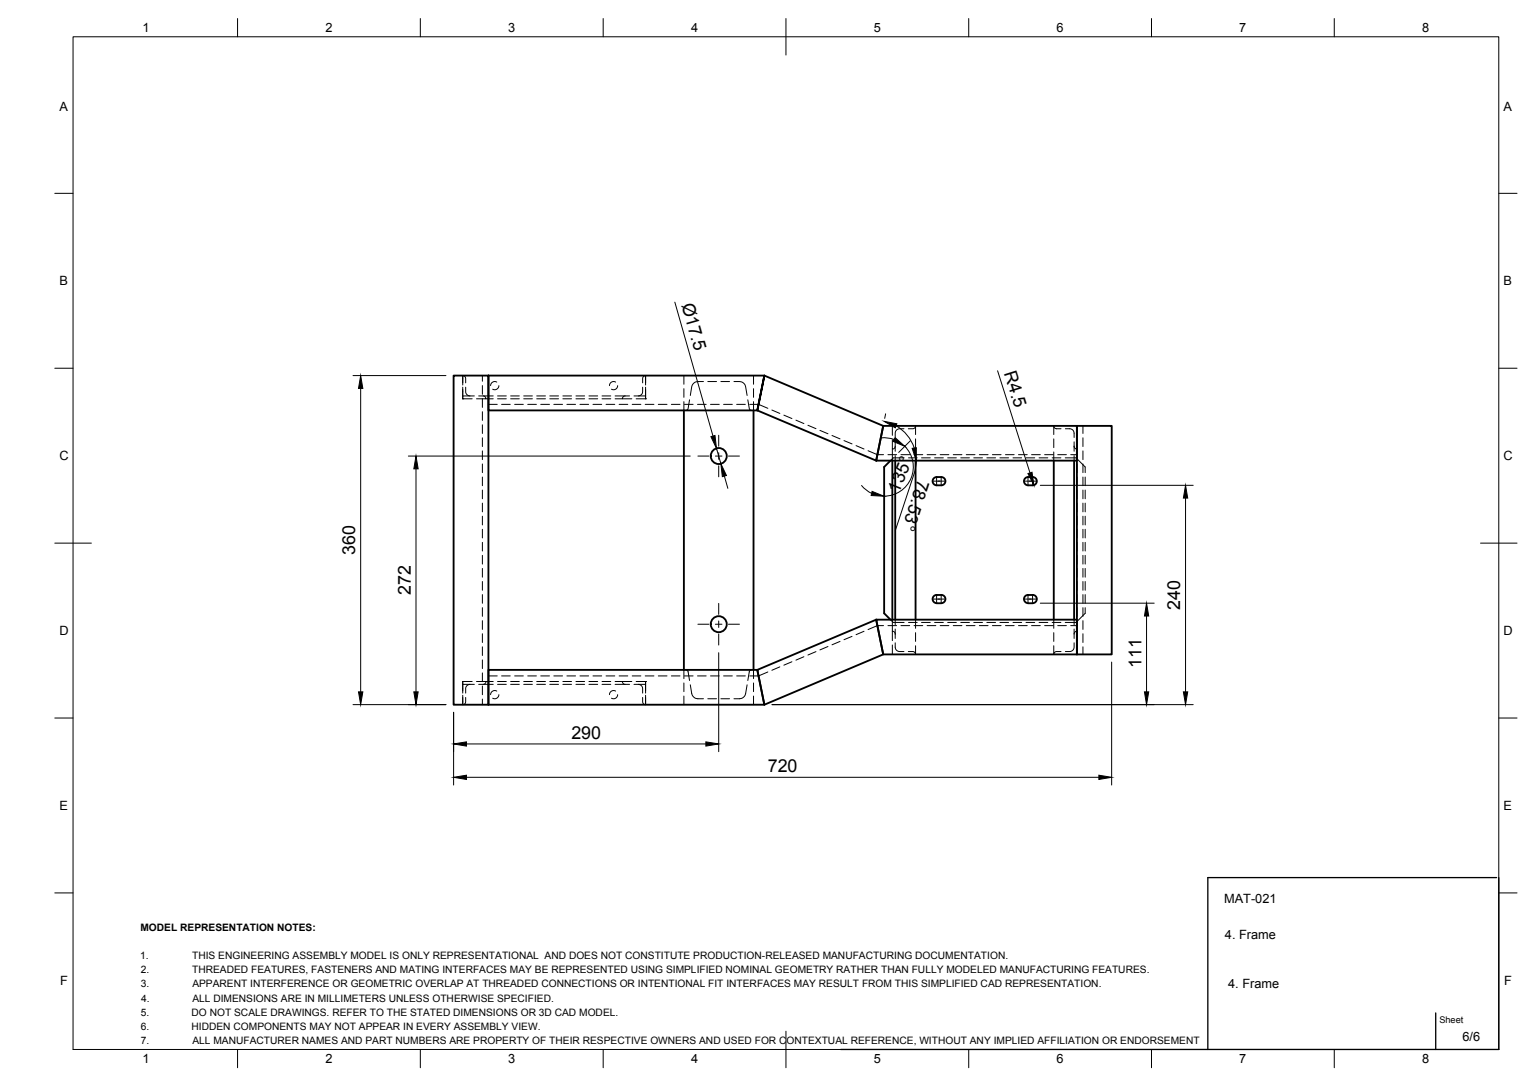
ISO-10303-21;
HEADER;
/* Generated by software containing ST-Developer
 * from STEP Tools, Inc. (www.steptools.com) 
 */

FILE_DESCRIPTION(
/* description */ ('STEP AP214'),
/* implementation_level */ '2;1');

FILE_NAME(
/* name */ '4. Frame.step',
/* time_stamp */ '2026-11-14T06:27:21-08:00',
/* author */ (''),
/* organization */ (''),
/* preprocessor_version */ 'ST-DEVELOPER v20.2',
/* originating_system */ 'Autodesk Translation Framework v15.17.0.0',
/* authorisation */ '');

FILE_SCHEMA (('AUTOMOTIVE_DESIGN { 1 0 10303 214 3 1 1 }'));
ENDSEC;

DATA;
#10=MECHANICAL_DESIGN_GEOMETRIC_PRESENTATION_REPRESENTATION('',(#38,#39,#40,#41,#42,#43,#44,#45,#46,#47,#48,#49,#50,#51,#52,#53,#54,#55,#56,#57,#58,#59,#60,#61),#27541);
#30=SHAPE_REPRESENTATION_RELATIONSHIP('SRR','None',#27564,#34);
#34=ADVANCED_BREP_SHAPE_REPRESENTATION('',(#65,#66,#67,#68,#69,#70,#71,
#72,#73,#74,#75,#76,#77,#78,#79,#80,#81,#82,#83,#84,#85,#86,#87,#88),#27540);
#38=STYLED_ITEM('',(#27590),#65);
#39=STYLED_ITEM('',(#27590),#66);
#40=STYLED_ITEM('',(#27590),#67);
#41=STYLED_ITEM('',(#27590),#68);
#42=STYLED_ITEM('',(#27590),#69);
#43=STYLED_ITEM('',(#27590),#70);
#44=STYLED_ITEM('',(#27590),#71);
#45=STYLED_ITEM('',(#27590),#72);
#46=STYLED_ITEM('',(#27590),#73);
#47=STYLED_ITEM('',(#27590),#74);
#48=STYLED_ITEM('',(#27590),#75);
#49=STYLED_ITEM('',(#27590),#76);
#50=STYLED_ITEM('',(#27590),#77);
#51=STYLED_ITEM('',(#27590),#78);
#52=STYLED_ITEM('',(#27590),#79);
#53=STYLED_ITEM('',(#27590),#80);
#54=STYLED_ITEM('',(#27590),#81);
#55=STYLED_ITEM('',(#27590),#82);
#56=STYLED_ITEM('',(#27590),#83);
#57=STYLED_ITEM('',(#27590),#84);
#58=STYLED_ITEM('',(#27590),#85);
#59=STYLED_ITEM('',(#27590),#86);
#60=STYLED_ITEM('',(#27590),#87);
#61=STYLED_ITEM('',(#27590),#88);
#65=MANIFOLD_SOLID_BREP('Body1',#11826);
#66=MANIFOLD_SOLID_BREP('Body2',#11827);
#67=MANIFOLD_SOLID_BREP('Body3',#11828);
#68=MANIFOLD_SOLID_BREP('Body4',#11829);
#69=MANIFOLD_SOLID_BREP('Body5',#11830);
#70=MANIFOLD_SOLID_BREP('Body6',#11831);
#71=MANIFOLD_SOLID_BREP('Body7',#11832);
#72=MANIFOLD_SOLID_BREP('Body8',#11833);
#73=MANIFOLD_SOLID_BREP('Body9',#11834);
#74=MANIFOLD_SOLID_BREP('Body10',#11835);
#75=MANIFOLD_SOLID_BREP('Body11',#11836);
#76=MANIFOLD_SOLID_BREP('Body12',#11837);
#77=MANIFOLD_SOLID_BREP('Body13',#11838);
#78=MANIFOLD_SOLID_BREP('Body14',#11839);
#79=MANIFOLD_SOLID_BREP('Body15',#11840);
#80=MANIFOLD_SOLID_BREP('Body16',#11841);
#81=MANIFOLD_SOLID_BREP('Body17',#11842);
#82=MANIFOLD_SOLID_BREP('Body18',#11843);
#83=MANIFOLD_SOLID_BREP('Body19',#11844);
#84=MANIFOLD_SOLID_BREP('Body20',#11845);
#85=MANIFOLD_SOLID_BREP('Body21',#11846);
#86=MANIFOLD_SOLID_BREP('Body22',#11847);
#87=MANIFOLD_SOLID_BREP('Body23',#11848);
#88=MANIFOLD_SOLID_BREP('Body24',#11849);
#133=ELLIPSE('',#12698,2.59172390171958,2.54000000000056);
#134=ELLIPSE('',#12701,6.9976545346413,6.85800000000022);
#135=ELLIPSE('',#12704,6.99765453464393,6.85800000000241);
#136=ELLIPSE('',#12707,2.59172390171943,2.54000000000021);
#137=ELLIPSE('',#12712,2.59172390172017,2.54000000000112);
#138=ELLIPSE('',#12713,6.99765453464255,6.8580000000014);
#139=ELLIPSE('',#12714,6.99765453464257,6.85800000000131);
#140=ELLIPSE('',#12715,2.59172390172489,2.5400000000054);
#141=ELLIPSE('',#12720,2.59172390172243,2.54000000000345);
#142=ELLIPSE('',#12723,6.99765453464225,6.85800000000097);
#143=ELLIPSE('',#12726,6.99765453464551,6.8580000000038);
#144=ELLIPSE('',#12729,2.59172390171343,2.53999999999498);
#145=ELLIPSE('',#12737,2.59172390171873,2.53999999999979);
#146=ELLIPSE('',#12741,6.99765453464068,6.85799999999964);
#147=ELLIPSE('',#12745,6.99765453464442,6.85800000000265);
#148=ELLIPSE('',#12749,2.5917239017157,2.53999999999687);
#149=ELLIPSE('',#12786,2.59172390172123,2.54000000000197);
#150=ELLIPSE('',#12789,6.99765453463971,6.85799999999854);
#151=ELLIPSE('',#12792,6.99765453464465,6.85800000000273);
#152=ELLIPSE('',#12795,2.59172390171767,2.53999999999863);
#153=ELLIPSE('',#12802,2.59172390172269,2.54000000000292);
#154=ELLIPSE('',#12806,6.99765453464155,6.85800000000042);
#155=ELLIPSE('',#12810,6.99765453463736,6.85799999999707);
#156=ELLIPSE('',#12814,2.59172390171622,2.5399999999978);
#157=ELLIPSE('',#12822,2.59172390171995,2.54000000000139);
#158=ELLIPSE('',#12823,6.99765453464566,6.85800000000388);
#159=ELLIPSE('',#12824,6.99765453464157,6.85800000000006);
#160=ELLIPSE('',#12825,2.59172390171781,2.53999999999902);
#161=ELLIPSE('',#12830,2.59172390171478,2.53999999999635);
#162=ELLIPSE('',#12833,6.99765453464405,6.85800000000235);
#163=ELLIPSE('',#12836,6.99765453464219,6.85800000000072);
#164=ELLIPSE('',#12839,2.59172390171126,2.53999999999298);
#165=ELLIPSE('',#12852,3.59210244842959,2.54000000000127);
#166=ELLIPSE('',#12855,9.69867661075609,6.8580000000008);
#167=ELLIPSE('',#12858,9.69867661075375,6.85799999999966);
#168=ELLIPSE('',#12861,3.59210244842762,2.54000000000046);
#169=ELLIPSE('',#12874,3.59210244842275,2.53999999999717);
#170=ELLIPSE('',#12877,9.69867661074225,6.8579999999926);
#171=ELLIPSE('',#12880,9.69867661075566,6.85800000000089);
#172=ELLIPSE('',#12883,3.59210244842444,2.53999999999849);
#173=ELLIPSE('',#12962,4.48294385563966,3.16992000000064);
#174=ELLIPSE('',#12965,6.73519209081142,4.76250000000638);
#175=ELLIPSE('',#12968,4.48294385563524,3.16991999999855);
#176=ELLIPSE('',#12975,4.48294385564325,3.16992000000392);
#177=ELLIPSE('',#12976,4.48294385563259,3.16991999999665);
#178=ELLIPSE('',#12979,6.73519209080091,4.76249999999985);
#179=ELLIPSE('',#12980,6.735192090809,4.76250000000462);
#180=ELLIPSE('',#12983,4.48294385564188,3.16992000000291);
#181=ELLIPSE('',#12984,4.48294385563158,3.16991999999587);
#182=ELLIPSE('',#12996,4.48294385563683,3.16991999999945);
#183=ELLIPSE('',#12999,6.73519209079765,4.7624999999967);
#184=ELLIPSE('',#13002,4.48294385564503,3.16992000000453);
#185=ELLIPSE('',#13013,4.482943855623,3.16991999998934);
#186=ELLIPSE('',#13016,6.73519209079788,4.76249999999742);
#187=ELLIPSE('',#13019,4.48294385563564,3.16991999999873);
#188=ELLIPSE('',#13026,4.48294385563249,3.16991999999556);
#189=ELLIPSE('',#13027,4.48294385564679,3.16992000000566);
#190=ELLIPSE('',#13030,6.73519209079125,4.76249999999378);
#191=ELLIPSE('',#13031,6.73519209079818,4.76249999999747);
#192=ELLIPSE('',#13034,4.48294385563025,3.16991999999552);
#193=ELLIPSE('',#13035,4.48294385563672,3.16991999999823);
#194=ELLIPSE('',#13047,4.48294385564801,3.16992000000646);
#195=ELLIPSE('',#13050,6.73519209080312,4.76250000000048);
#196=ELLIPSE('',#13053,4.48294385563554,3.16991999999886);
#197=ELLIPSE('',#13108,3.59210244842469,2.53999999999847);
#198=ELLIPSE('',#13109,3.59210244843125,2.54000000000209);
#199=ELLIPSE('',#13112,9.69867661075553,6.85800000000037);
#200=ELLIPSE('',#13113,9.69867661075507,6.85800000000035);
#201=ELLIPSE('',#13116,9.69867661075306,6.85799999999952);
#202=ELLIPSE('',#13117,9.6986766107561,6.85800000000094);
#203=ELLIPSE('',#13120,3.592102448417,2.53999999999353);
#204=ELLIPSE('',#13121,3.59210244843681,2.54000000000594);
#318=PLANE('',#12667);
#319=PLANE('',#12668);
#320=PLANE('',#12672);
#321=PLANE('',#12676);
#322=PLANE('',#12680);
#323=PLANE('',#12684);
#324=PLANE('',#12685);
#325=PLANE('',#12686);
#326=PLANE('',#12687);
#327=PLANE('',#12688);
#328=PLANE('',#12689);
#329=PLANE('',#12694);
#330=PLANE('',#12695);
#331=PLANE('',#12696);
#332=PLANE('',#12699);
#333=PLANE('',#12702);
#334=PLANE('',#12705);
#335=PLANE('',#12708);
#336=PLANE('',#12709);
#337=PLANE('',#12710);
#338=PLANE('',#12711);
#339=PLANE('',#12716);
#340=PLANE('',#12717);
#341=PLANE('',#12718);
#342=PLANE('',#12721);
#343=PLANE('',#12724);
#344=PLANE('',#12727);
#345=PLANE('',#12730);
#346=PLANE('',#12731);
#347=PLANE('',#12732);
#348=PLANE('',#12733);
#349=PLANE('',#12734);
#350=PLANE('',#12738);
#351=PLANE('',#12742);
#352=PLANE('',#12746);
#353=PLANE('',#12750);
#354=PLANE('',#12751);
#355=PLANE('',#12752);
#356=PLANE('',#12753);
#357=PLANE('',#12754);
#358=PLANE('',#12755);
#359=PLANE('',#12756);
#360=PLANE('',#12760);
#361=PLANE('',#12764);
#362=PLANE('',#12768);
#363=PLANE('',#12772);
#364=PLANE('',#12773);
#365=PLANE('',#12774);
#366=PLANE('',#12775);
#367=PLANE('',#12776);
#368=PLANE('',#12777);
#369=PLANE('',#12782);
#370=PLANE('',#12783);
#371=PLANE('',#12784);
#372=PLANE('',#12787);
#373=PLANE('',#12790);
#374=PLANE('',#12793);
#375=PLANE('',#12796);
#376=PLANE('',#12797);
#377=PLANE('',#12798);
#378=PLANE('',#12799);
#379=PLANE('',#12800);
#380=PLANE('',#12804);
#381=PLANE('',#12808);
#382=PLANE('',#12812);
#383=PLANE('',#12816);
#384=PLANE('',#12817);
#385=PLANE('',#12818);
#386=PLANE('',#12819);
#387=PLANE('',#12820);
#388=PLANE('',#12821);
#389=PLANE('',#12826);
#390=PLANE('',#12827);
#391=PLANE('',#12828);
#392=PLANE('',#12831);
#393=PLANE('',#12834);
#394=PLANE('',#12837);
#395=PLANE('',#12840);
#396=PLANE('',#12841);
#397=PLANE('',#12842);
#398=PLANE('',#12843);
#399=PLANE('',#12848);
#400=PLANE('',#12849);
#401=PLANE('',#12850);
#402=PLANE('',#12853);
#403=PLANE('',#12856);
#404=PLANE('',#12859);
#405=PLANE('',#12862);
#406=PLANE('',#12863);
#407=PLANE('',#12864);
#408=PLANE('',#12865);
#409=PLANE('',#12870);
#410=PLANE('',#12871);
#411=PLANE('',#12872);
#412=PLANE('',#12875);
#413=PLANE('',#12878);
#414=PLANE('',#12881);
#415=PLANE('',#12884);
#416=PLANE('',#12885);
#417=PLANE('',#12886);
#418=PLANE('',#12887);
#419=PLANE('',#12888);
#420=PLANE('',#12892);
#421=PLANE('',#12896);
#422=PLANE('',#12900);
#423=PLANE('',#12901);
#424=PLANE('',#12902);
#425=PLANE('',#12903);
#426=PLANE('',#12904);
#427=PLANE('',#12905);
#428=PLANE('',#12909);
#429=PLANE('',#12913);
#430=PLANE('',#12917);
#431=PLANE('',#12918);
#432=PLANE('',#12919);
#433=PLANE('',#12920);
#434=PLANE('',#12921);
#435=PLANE('',#12922);
#436=PLANE('',#12926);
#437=PLANE('',#12930);
#438=PLANE('',#12934);
#439=PLANE('',#12935);
#440=PLANE('',#12936);
#441=PLANE('',#12937);
#442=PLANE('',#12938);
#443=PLANE('',#12939);
#444=PLANE('',#12943);
#445=PLANE('',#12947);
#446=PLANE('',#12951);
#447=PLANE('',#12952);
#448=PLANE('',#12953);
#449=PLANE('',#12954);
#450=PLANE('',#12955);
#451=PLANE('',#12959);
#452=PLANE('',#12960);
#453=PLANE('',#12963);
#454=PLANE('',#12966);
#455=PLANE('',#12969);
#456=PLANE('',#12970);
#457=PLANE('',#12971);
#458=PLANE('',#12972);
#459=PLANE('',#12973);
#460=PLANE('',#12977);
#461=PLANE('',#12981);
#462=PLANE('',#12985);
#463=PLANE('',#12986);
#464=PLANE('',#12987);
#465=PLANE('',#12988);
#466=PLANE('',#12989);
#467=PLANE('',#12993);
#468=PLANE('',#12994);
#469=PLANE('',#12997);
#470=PLANE('',#13000);
#471=PLANE('',#13003);
#472=PLANE('',#13004);
#473=PLANE('',#13005);
#474=PLANE('',#13006);
#475=PLANE('',#13010);
#476=PLANE('',#13011);
#477=PLANE('',#13014);
#478=PLANE('',#13017);
#479=PLANE('',#13020);
#480=PLANE('',#13021);
#481=PLANE('',#13022);
#482=PLANE('',#13023);
#483=PLANE('',#13024);
#484=PLANE('',#13028);
#485=PLANE('',#13032);
#486=PLANE('',#13036);
#487=PLANE('',#13037);
#488=PLANE('',#13038);
#489=PLANE('',#13039);
#490=PLANE('',#13040);
#491=PLANE('',#13044);
#492=PLANE('',#13045);
#493=PLANE('',#13048);
#494=PLANE('',#13051);
#495=PLANE('',#13054);
#496=PLANE('',#13055);
#497=PLANE('',#13056);
#498=PLANE('',#13069);
#499=PLANE('',#13070);
#500=PLANE('',#13071);
#501=PLANE('',#13072);
#502=PLANE('',#13073);
#503=PLANE('',#13078);
#504=PLANE('',#13083);
#505=PLANE('',#13085);
#506=PLANE('',#13086);
#507=PLANE('',#13088);
#508=PLANE('',#13089);
#509=PLANE('',#13091);
#510=PLANE('',#13092);
#511=PLANE('',#13094);
#512=PLANE('',#13095);
#513=PLANE('',#13096);
#514=PLANE('',#13097);
#515=PLANE('',#13098);
#516=PLANE('',#13105);
#517=PLANE('',#13106);
#518=PLANE('',#13110);
#519=PLANE('',#13114);
#520=PLANE('',#13118);
#521=PLANE('',#13122);
#522=PLANE('',#13123);
#523=PLANE('',#13124);
#524=PLANE('',#13125);
#525=PLANE('',#13126);
#526=PLANE('',#13133);
#527=PLANE('',#13134);
#528=PLANE('',#13138);
#529=PLANE('',#13142);
#530=PLANE('',#13146);
#531=PLANE('',#13147);
#532=PLANE('',#13148);
#533=PLANE('',#13149);
#534=PLANE('',#13156);
#535=PLANE('',#13157);
#536=PLANE('',#13161);
#537=PLANE('',#13165);
#538=PLANE('',#13169);
#539=PLANE('',#13170);
#540=PLANE('',#13171);
#541=PLANE('',#13172);
#597=FACE_BOUND('',#2061,.T.);
#598=FACE_BOUND('',#2062,.T.);
#599=FACE_BOUND('',#2063,.T.);
#600=FACE_BOUND('',#2064,.T.);
#601=FACE_BOUND('',#2066,.T.);
#602=FACE_BOUND('',#2067,.T.);
#603=FACE_BOUND('',#2068,.T.);
#604=FACE_BOUND('',#2069,.T.);
#605=FACE_BOUND('',#2094,.T.);
#606=FACE_BOUND('',#2095,.T.);
#607=FACE_BOUND('',#2102,.T.);
#608=FACE_BOUND('',#2103,.T.);
#609=FACE_BOUND('',#2109,.T.);
#610=FACE_BOUND('',#2110,.T.);
#611=FACE_BOUND('',#2114,.T.);
#612=FACE_BOUND('',#2115,.T.);
#613=FACE_BOUND('',#2126,.T.);
#614=FACE_BOUND('',#2127,.T.);
#615=FACE_BOUND('',#2131,.T.);
#616=FACE_BOUND('',#2132,.T.);
#1066=FACE_OUTER_BOUND('',#1802,.T.);
#1067=FACE_OUTER_BOUND('',#1803,.T.);
#1068=FACE_OUTER_BOUND('',#1804,.T.);
#1069=FACE_OUTER_BOUND('',#1805,.T.);
#1070=FACE_OUTER_BOUND('',#1806,.T.);
#1071=FACE_OUTER_BOUND('',#1807,.T.);
#1072=FACE_OUTER_BOUND('',#1808,.T.);
#1073=FACE_OUTER_BOUND('',#1809,.T.);
#1074=FACE_OUTER_BOUND('',#1810,.T.);
#1075=FACE_OUTER_BOUND('',#1811,.T.);
#1076=FACE_OUTER_BOUND('',#1812,.T.);
#1077=FACE_OUTER_BOUND('',#1813,.T.);
#1078=FACE_OUTER_BOUND('',#1814,.T.);
#1079=FACE_OUTER_BOUND('',#1815,.T.);
#1080=FACE_OUTER_BOUND('',#1816,.T.);
#1081=FACE_OUTER_BOUND('',#1817,.T.);
#1082=FACE_OUTER_BOUND('',#1818,.T.);
#1083=FACE_OUTER_BOUND('',#1819,.T.);
#1084=FACE_OUTER_BOUND('',#1820,.T.);
#1085=FACE_OUTER_BOUND('',#1821,.T.);
#1086=FACE_OUTER_BOUND('',#1822,.T.);
#1087=FACE_OUTER_BOUND('',#1823,.T.);
#1088=FACE_OUTER_BOUND('',#1824,.T.);
#1089=FACE_OUTER_BOUND('',#1825,.T.);
#1090=FACE_OUTER_BOUND('',#1826,.T.);
#1091=FACE_OUTER_BOUND('',#1827,.T.);
#1092=FACE_OUTER_BOUND('',#1828,.T.);
#1093=FACE_OUTER_BOUND('',#1829,.T.);
#1094=FACE_OUTER_BOUND('',#1830,.T.);
#1095=FACE_OUTER_BOUND('',#1831,.T.);
#1096=FACE_OUTER_BOUND('',#1832,.T.);
#1097=FACE_OUTER_BOUND('',#1833,.T.);
#1098=FACE_OUTER_BOUND('',#1834,.T.);
#1099=FACE_OUTER_BOUND('',#1835,.T.);
#1100=FACE_OUTER_BOUND('',#1836,.T.);
#1101=FACE_OUTER_BOUND('',#1837,.T.);
#1102=FACE_OUTER_BOUND('',#1838,.T.);
#1103=FACE_OUTER_BOUND('',#1839,.T.);
#1104=FACE_OUTER_BOUND('',#1840,.T.);
#1105=FACE_OUTER_BOUND('',#1841,.T.);
#1106=FACE_OUTER_BOUND('',#1842,.T.);
#1107=FACE_OUTER_BOUND('',#1843,.T.);
#1108=FACE_OUTER_BOUND('',#1844,.T.);
#1109=FACE_OUTER_BOUND('',#1845,.T.);
#1110=FACE_OUTER_BOUND('',#1846,.T.);
#1111=FACE_OUTER_BOUND('',#1847,.T.);
#1112=FACE_OUTER_BOUND('',#1848,.T.);
#1113=FACE_OUTER_BOUND('',#1849,.T.);
#1114=FACE_OUTER_BOUND('',#1850,.T.);
#1115=FACE_OUTER_BOUND('',#1851,.T.);
#1116=FACE_OUTER_BOUND('',#1852,.T.);
#1117=FACE_OUTER_BOUND('',#1853,.T.);
#1118=FACE_OUTER_BOUND('',#1854,.T.);
#1119=FACE_OUTER_BOUND('',#1855,.T.);
#1120=FACE_OUTER_BOUND('',#1856,.T.);
#1121=FACE_OUTER_BOUND('',#1857,.T.);
#1122=FACE_OUTER_BOUND('',#1858,.T.);
#1123=FACE_OUTER_BOUND('',#1859,.T.);
#1124=FACE_OUTER_BOUND('',#1860,.T.);
#1125=FACE_OUTER_BOUND('',#1861,.T.);
#1126=FACE_OUTER_BOUND('',#1862,.T.);
#1127=FACE_OUTER_BOUND('',#1863,.T.);
#1128=FACE_OUTER_BOUND('',#1864,.T.);
#1129=FACE_OUTER_BOUND('',#1865,.T.);
#1130=FACE_OUTER_BOUND('',#1866,.T.);
#1131=FACE_OUTER_BOUND('',#1867,.T.);
#1132=FACE_OUTER_BOUND('',#1868,.T.);
#1133=FACE_OUTER_BOUND('',#1869,.T.);
#1134=FACE_OUTER_BOUND('',#1870,.T.);
#1135=FACE_OUTER_BOUND('',#1871,.T.);
#1136=FACE_OUTER_BOUND('',#1872,.T.);
#1137=FACE_OUTER_BOUND('',#1873,.T.);
#1138=FACE_OUTER_BOUND('',#1874,.T.);
#1139=FACE_OUTER_BOUND('',#1875,.T.);
#1140=FACE_OUTER_BOUND('',#1876,.T.);
#1141=FACE_OUTER_BOUND('',#1877,.T.);
#1142=FACE_OUTER_BOUND('',#1878,.T.);
#1143=FACE_OUTER_BOUND('',#1879,.T.);
#1144=FACE_OUTER_BOUND('',#1880,.T.);
#1145=FACE_OUTER_BOUND('',#1881,.T.);
#1146=FACE_OUTER_BOUND('',#1882,.T.);
#1147=FACE_OUTER_BOUND('',#1883,.T.);
#1148=FACE_OUTER_BOUND('',#1884,.T.);
#1149=FACE_OUTER_BOUND('',#1885,.T.);
#1150=FACE_OUTER_BOUND('',#1886,.T.);
#1151=FACE_OUTER_BOUND('',#1887,.T.);
#1152=FACE_OUTER_BOUND('',#1888,.T.);
#1153=FACE_OUTER_BOUND('',#1889,.T.);
#1154=FACE_OUTER_BOUND('',#1890,.T.);
#1155=FACE_OUTER_BOUND('',#1891,.T.);
#1156=FACE_OUTER_BOUND('',#1892,.T.);
#1157=FACE_OUTER_BOUND('',#1893,.T.);
#1158=FACE_OUTER_BOUND('',#1894,.T.);
#1159=FACE_OUTER_BOUND('',#1895,.T.);
#1160=FACE_OUTER_BOUND('',#1896,.T.);
#1161=FACE_OUTER_BOUND('',#1897,.T.);
#1162=FACE_OUTER_BOUND('',#1898,.T.);
#1163=FACE_OUTER_BOUND('',#1899,.T.);
#1164=FACE_OUTER_BOUND('',#1900,.T.);
#1165=FACE_OUTER_BOUND('',#1901,.T.);
#1166=FACE_OUTER_BOUND('',#1902,.T.);
#1167=FACE_OUTER_BOUND('',#1903,.T.);
#1168=FACE_OUTER_BOUND('',#1904,.T.);
#1169=FACE_OUTER_BOUND('',#1905,.T.);
#1170=FACE_OUTER_BOUND('',#1906,.T.);
#1171=FACE_OUTER_BOUND('',#1907,.T.);
#1172=FACE_OUTER_BOUND('',#1908,.T.);
#1173=FACE_OUTER_BOUND('',#1909,.T.);
#1174=FACE_OUTER_BOUND('',#1910,.T.);
#1175=FACE_OUTER_BOUND('',#1911,.T.);
#1176=FACE_OUTER_BOUND('',#1912,.T.);
#1177=FACE_OUTER_BOUND('',#1913,.T.);
#1178=FACE_OUTER_BOUND('',#1914,.T.);
#1179=FACE_OUTER_BOUND('',#1915,.T.);
#1180=FACE_OUTER_BOUND('',#1916,.T.);
#1181=FACE_OUTER_BOUND('',#1917,.T.);
#1182=FACE_OUTER_BOUND('',#1918,.T.);
#1183=FACE_OUTER_BOUND('',#1919,.T.);
#1184=FACE_OUTER_BOUND('',#1920,.T.);
#1185=FACE_OUTER_BOUND('',#1921,.T.);
#1186=FACE_OUTER_BOUND('',#1922,.T.);
#1187=FACE_OUTER_BOUND('',#1923,.T.);
#1188=FACE_OUTER_BOUND('',#1924,.T.);
#1189=FACE_OUTER_BOUND('',#1925,.T.);
#1190=FACE_OUTER_BOUND('',#1926,.T.);
#1191=FACE_OUTER_BOUND('',#1927,.T.);
#1192=FACE_OUTER_BOUND('',#1928,.T.);
#1193=FACE_OUTER_BOUND('',#1929,.T.);
#1194=FACE_OUTER_BOUND('',#1930,.T.);
#1195=FACE_OUTER_BOUND('',#1931,.T.);
#1196=FACE_OUTER_BOUND('',#1932,.T.);
#1197=FACE_OUTER_BOUND('',#1933,.T.);
#1198=FACE_OUTER_BOUND('',#1934,.T.);
#1199=FACE_OUTER_BOUND('',#1935,.T.);
#1200=FACE_OUTER_BOUND('',#1936,.T.);
#1201=FACE_OUTER_BOUND('',#1937,.T.);
#1202=FACE_OUTER_BOUND('',#1938,.T.);
#1203=FACE_OUTER_BOUND('',#1939,.T.);
#1204=FACE_OUTER_BOUND('',#1940,.T.);
#1205=FACE_OUTER_BOUND('',#1941,.T.);
#1206=FACE_OUTER_BOUND('',#1942,.T.);
#1207=FACE_OUTER_BOUND('',#1943,.T.);
#1208=FACE_OUTER_BOUND('',#1944,.T.);
#1209=FACE_OUTER_BOUND('',#1945,.T.);
#1210=FACE_OUTER_BOUND('',#1946,.T.);
#1211=FACE_OUTER_BOUND('',#1947,.T.);
#1212=FACE_OUTER_BOUND('',#1948,.T.);
#1213=FACE_OUTER_BOUND('',#1949,.T.);
#1214=FACE_OUTER_BOUND('',#1950,.T.);
#1215=FACE_OUTER_BOUND('',#1951,.T.);
#1216=FACE_OUTER_BOUND('',#1952,.T.);
#1217=FACE_OUTER_BOUND('',#1953,.T.);
#1218=FACE_OUTER_BOUND('',#1954,.T.);
#1219=FACE_OUTER_BOUND('',#1955,.T.);
#1220=FACE_OUTER_BOUND('',#1956,.T.);
#1221=FACE_OUTER_BOUND('',#1957,.T.);
#1222=FACE_OUTER_BOUND('',#1958,.T.);
#1223=FACE_OUTER_BOUND('',#1959,.T.);
#1224=FACE_OUTER_BOUND('',#1960,.T.);
#1225=FACE_OUTER_BOUND('',#1961,.T.);
#1226=FACE_OUTER_BOUND('',#1962,.T.);
#1227=FACE_OUTER_BOUND('',#1963,.T.);
#1228=FACE_OUTER_BOUND('',#1964,.T.);
#1229=FACE_OUTER_BOUND('',#1965,.T.);
#1230=FACE_OUTER_BOUND('',#1966,.T.);
#1231=FACE_OUTER_BOUND('',#1967,.T.);
#1232=FACE_OUTER_BOUND('',#1968,.T.);
#1233=FACE_OUTER_BOUND('',#1969,.T.);
#1234=FACE_OUTER_BOUND('',#1970,.T.);
#1235=FACE_OUTER_BOUND('',#1971,.T.);
#1236=FACE_OUTER_BOUND('',#1972,.T.);
#1237=FACE_OUTER_BOUND('',#1973,.T.);
#1238=FACE_OUTER_BOUND('',#1974,.T.);
#1239=FACE_OUTER_BOUND('',#1975,.T.);
#1240=FACE_OUTER_BOUND('',#1976,.T.);
#1241=FACE_OUTER_BOUND('',#1977,.T.);
#1242=FACE_OUTER_BOUND('',#1978,.T.);
#1243=FACE_OUTER_BOUND('',#1979,.T.);
#1244=FACE_OUTER_BOUND('',#1980,.T.);
#1245=FACE_OUTER_BOUND('',#1981,.T.);
#1246=FACE_OUTER_BOUND('',#1982,.T.);
#1247=FACE_OUTER_BOUND('',#1983,.T.);
#1248=FACE_OUTER_BOUND('',#1984,.T.);
#1249=FACE_OUTER_BOUND('',#1985,.T.);
#1250=FACE_OUTER_BOUND('',#1986,.T.);
#1251=FACE_OUTER_BOUND('',#1987,.T.);
#1252=FACE_OUTER_BOUND('',#1988,.T.);
#1253=FACE_OUTER_BOUND('',#1989,.T.);
#1254=FACE_OUTER_BOUND('',#1990,.T.);
#1255=FACE_OUTER_BOUND('',#1991,.T.);
#1256=FACE_OUTER_BOUND('',#1992,.T.);
#1257=FACE_OUTER_BOUND('',#1993,.T.);
#1258=FACE_OUTER_BOUND('',#1994,.T.);
#1259=FACE_OUTER_BOUND('',#1995,.T.);
#1260=FACE_OUTER_BOUND('',#1996,.T.);
#1261=FACE_OUTER_BOUND('',#1997,.T.);
#1262=FACE_OUTER_BOUND('',#1998,.T.);
#1263=FACE_OUTER_BOUND('',#1999,.T.);
#1264=FACE_OUTER_BOUND('',#2000,.T.);
#1265=FACE_OUTER_BOUND('',#2001,.T.);
#1266=FACE_OUTER_BOUND('',#2002,.T.);
#1267=FACE_OUTER_BOUND('',#2003,.T.);
#1268=FACE_OUTER_BOUND('',#2004,.T.);
#1269=FACE_OUTER_BOUND('',#2005,.T.);
#1270=FACE_OUTER_BOUND('',#2006,.T.);
#1271=FACE_OUTER_BOUND('',#2007,.T.);
#1272=FACE_OUTER_BOUND('',#2008,.T.);
#1273=FACE_OUTER_BOUND('',#2009,.T.);
#1274=FACE_OUTER_BOUND('',#2010,.T.);
#1275=FACE_OUTER_BOUND('',#2011,.T.);
#1276=FACE_OUTER_BOUND('',#2012,.T.);
#1277=FACE_OUTER_BOUND('',#2013,.T.);
#1278=FACE_OUTER_BOUND('',#2014,.T.);
#1279=FACE_OUTER_BOUND('',#2015,.T.);
#1280=FACE_OUTER_BOUND('',#2016,.T.);
#1281=FACE_OUTER_BOUND('',#2017,.T.);
#1282=FACE_OUTER_BOUND('',#2018,.T.);
#1283=FACE_OUTER_BOUND('',#2019,.T.);
#1284=FACE_OUTER_BOUND('',#2020,.T.);
#1285=FACE_OUTER_BOUND('',#2021,.T.);
#1286=FACE_OUTER_BOUND('',#2022,.T.);
#1287=FACE_OUTER_BOUND('',#2023,.T.);
#1288=FACE_OUTER_BOUND('',#2024,.T.);
#1289=FACE_OUTER_BOUND('',#2025,.T.);
#1290=FACE_OUTER_BOUND('',#2026,.T.);
#1291=FACE_OUTER_BOUND('',#2027,.T.);
#1292=FACE_OUTER_BOUND('',#2028,.T.);
#1293=FACE_OUTER_BOUND('',#2029,.T.);
#1294=FACE_OUTER_BOUND('',#2030,.T.);
#1295=FACE_OUTER_BOUND('',#2031,.T.);
#1296=FACE_OUTER_BOUND('',#2032,.T.);
#1297=FACE_OUTER_BOUND('',#2033,.T.);
#1298=FACE_OUTER_BOUND('',#2034,.T.);
#1299=FACE_OUTER_BOUND('',#2035,.T.);
#1300=FACE_OUTER_BOUND('',#2036,.T.);
#1301=FACE_OUTER_BOUND('',#2037,.T.);
#1302=FACE_OUTER_BOUND('',#2038,.T.);
#1303=FACE_OUTER_BOUND('',#2039,.T.);
#1304=FACE_OUTER_BOUND('',#2040,.T.);
#1305=FACE_OUTER_BOUND('',#2041,.T.);
#1306=FACE_OUTER_BOUND('',#2042,.T.);
#1307=FACE_OUTER_BOUND('',#2043,.T.);
#1308=FACE_OUTER_BOUND('',#2044,.T.);
#1309=FACE_OUTER_BOUND('',#2045,.T.);
#1310=FACE_OUTER_BOUND('',#2046,.T.);
#1311=FACE_OUTER_BOUND('',#2047,.T.);
#1312=FACE_OUTER_BOUND('',#2048,.T.);
#1313=FACE_OUTER_BOUND('',#2049,.T.);
#1314=FACE_OUTER_BOUND('',#2050,.T.);
#1315=FACE_OUTER_BOUND('',#2051,.T.);
#1316=FACE_OUTER_BOUND('',#2052,.T.);
#1317=FACE_OUTER_BOUND('',#2053,.T.);
#1318=FACE_OUTER_BOUND('',#2054,.T.);
#1319=FACE_OUTER_BOUND('',#2055,.T.);
#1320=FACE_OUTER_BOUND('',#2056,.T.);
#1321=FACE_OUTER_BOUND('',#2057,.T.);
#1322=FACE_OUTER_BOUND('',#2058,.T.);
#1323=FACE_OUTER_BOUND('',#2059,.T.);
#1324=FACE_OUTER_BOUND('',#2060,.T.);
#1325=FACE_OUTER_BOUND('',#2065,.T.);
#1326=FACE_OUTER_BOUND('',#2070,.T.);
#1327=FACE_OUTER_BOUND('',#2071,.T.);
#1328=FACE_OUTER_BOUND('',#2072,.T.);
#1329=FACE_OUTER_BOUND('',#2073,.T.);
#1330=FACE_OUTER_BOUND('',#2074,.T.);
#1331=FACE_OUTER_BOUND('',#2075,.T.);
#1332=FACE_OUTER_BOUND('',#2076,.T.);
#1333=FACE_OUTER_BOUND('',#2077,.T.);
#1334=FACE_OUTER_BOUND('',#2078,.T.);
#1335=FACE_OUTER_BOUND('',#2079,.T.);
#1336=FACE_OUTER_BOUND('',#2080,.T.);
#1337=FACE_OUTER_BOUND('',#2081,.T.);
#1338=FACE_OUTER_BOUND('',#2082,.T.);
#1339=FACE_OUTER_BOUND('',#2083,.T.);
#1340=FACE_OUTER_BOUND('',#2084,.T.);
#1341=FACE_OUTER_BOUND('',#2085,.T.);
#1342=FACE_OUTER_BOUND('',#2086,.T.);
#1343=FACE_OUTER_BOUND('',#2087,.T.);
#1344=FACE_OUTER_BOUND('',#2088,.T.);
#1345=FACE_OUTER_BOUND('',#2089,.T.);
#1346=FACE_OUTER_BOUND('',#2090,.T.);
#1347=FACE_OUTER_BOUND('',#2091,.T.);
#1348=FACE_OUTER_BOUND('',#2092,.T.);
#1349=FACE_OUTER_BOUND('',#2093,.T.);
#1350=FACE_OUTER_BOUND('',#2096,.T.);
#1351=FACE_OUTER_BOUND('',#2097,.T.);
#1352=FACE_OUTER_BOUND('',#2098,.T.);
#1353=FACE_OUTER_BOUND('',#2099,.T.);
#1354=FACE_OUTER_BOUND('',#2100,.T.);
#1355=FACE_OUTER_BOUND('',#2101,.T.);
#1356=FACE_OUTER_BOUND('',#2104,.T.);
#1357=FACE_OUTER_BOUND('',#2105,.T.);
#1358=FACE_OUTER_BOUND('',#2106,.T.);
#1359=FACE_OUTER_BOUND('',#2107,.T.);
#1360=FACE_OUTER_BOUND('',#2108,.T.);
#1361=FACE_OUTER_BOUND('',#2111,.T.);
#1362=FACE_OUTER_BOUND('',#2112,.T.);
#1363=FACE_OUTER_BOUND('',#2113,.T.);
#1364=FACE_OUTER_BOUND('',#2116,.T.);
#1365=FACE_OUTER_BOUND('',#2117,.T.);
#1366=FACE_OUTER_BOUND('',#2118,.T.);
#1367=FACE_OUTER_BOUND('',#2119,.T.);
#1368=FACE_OUTER_BOUND('',#2120,.T.);
#1369=FACE_OUTER_BOUND('',#2121,.T.);
#1370=FACE_OUTER_BOUND('',#2122,.T.);
#1371=FACE_OUTER_BOUND('',#2123,.T.);
#1372=FACE_OUTER_BOUND('',#2124,.T.);
#1373=FACE_OUTER_BOUND('',#2125,.T.);
#1374=FACE_OUTER_BOUND('',#2128,.T.);
#1375=FACE_OUTER_BOUND('',#2129,.T.);
#1376=FACE_OUTER_BOUND('',#2130,.T.);
#1377=FACE_OUTER_BOUND('',#2133,.T.);
#1378=FACE_OUTER_BOUND('',#2134,.T.);
#1379=FACE_OUTER_BOUND('',#2135,.T.);
#1380=FACE_OUTER_BOUND('',#2136,.T.);
#1381=FACE_OUTER_BOUND('',#2137,.T.);
#1382=FACE_OUTER_BOUND('',#2138,.T.);
#1383=FACE_OUTER_BOUND('',#2139,.T.);
#1802=EDGE_LOOP('',(#9300,#9301,#9302,#9303));
#1803=EDGE_LOOP('',(#9304,#9305,#9306,#9307));
#1804=EDGE_LOOP('',(#9308,#9309,#9310,#9311));
#1805=EDGE_LOOP('',(#9312,#9313,#9314,#9315));
#1806=EDGE_LOOP('',(#9316,#9317,#9318,#9319));
#1807=EDGE_LOOP('',(#9320,#9321,#9322,#9323));
#1808=EDGE_LOOP('',(#9324,#9325,#9326,#9327));
#1809=EDGE_LOOP('',(#9328,#9329,#9330,#9331));
#1810=EDGE_LOOP('',(#9332,#9333,#9334,#9335));
#1811=EDGE_LOOP('',(#9336,#9337,#9338,#9339));
#1812=EDGE_LOOP('',(#9340,#9341,#9342,#9343));
#1813=EDGE_LOOP('',(#9344,#9345,#9346,#9347));
#1814=EDGE_LOOP('',(#9348,#9349,#9350,#9351,#9352,#9353,#9354,#9355,#9356,
#9357,#9358,#9359));
#1815=EDGE_LOOP('',(#9360,#9361,#9362,#9363,#9364,#9365,#9366,#9367,#9368,
#9369,#9370,#9371));
#1816=EDGE_LOOP('',(#9372,#9373,#9374,#9375,#9376,#9377,#9378,#9379,#9380,
#9381,#9382,#9383));
#1817=EDGE_LOOP('',(#9384,#9385,#9386,#9387));
#1818=EDGE_LOOP('',(#9388,#9389,#9390,#9391));
#1819=EDGE_LOOP('',(#9392,#9393,#9394,#9395));
#1820=EDGE_LOOP('',(#9396,#9397,#9398,#9399));
#1821=EDGE_LOOP('',(#9400,#9401,#9402,#9403));
#1822=EDGE_LOOP('',(#9404,#9405,#9406,#9407));
#1823=EDGE_LOOP('',(#9408,#9409,#9410,#9411));
#1824=EDGE_LOOP('',(#9412,#9413,#9414,#9415));
#1825=EDGE_LOOP('',(#9416,#9417,#9418,#9419));
#1826=EDGE_LOOP('',(#9420,#9421,#9422,#9423));
#1827=EDGE_LOOP('',(#9424,#9425,#9426,#9427));
#1828=EDGE_LOOP('',(#9428,#9429,#9430,#9431));
#1829=EDGE_LOOP('',(#9432,#9433,#9434,#9435,#9436,#9437,#9438,#9439,#9440,
#9441,#9442,#9443));
#1830=EDGE_LOOP('',(#9444,#9445,#9446,#9447,#9448,#9449,#9450,#9451,#9452,
#9453,#9454,#9455));
#1831=EDGE_LOOP('',(#9456,#9457,#9458,#9459));
#1832=EDGE_LOOP('',(#9460,#9461,#9462,#9463));
#1833=EDGE_LOOP('',(#9464,#9465,#9466,#9467));
#1834=EDGE_LOOP('',(#9468,#9469,#9470,#9471));
#1835=EDGE_LOOP('',(#9472,#9473,#9474,#9475));
#1836=EDGE_LOOP('',(#9476,#9477,#9478,#9479));
#1837=EDGE_LOOP('',(#9480,#9481,#9482,#9483));
#1838=EDGE_LOOP('',(#9484,#9485,#9486,#9487));
#1839=EDGE_LOOP('',(#9488,#9489,#9490,#9491));
#1840=EDGE_LOOP('',(#9492,#9493,#9494,#9495));
#1841=EDGE_LOOP('',(#9496,#9497,#9498,#9499));
#1842=EDGE_LOOP('',(#9500,#9501,#9502,#9503));
#1843=EDGE_LOOP('',(#9504,#9505,#9506,#9507,#9508,#9509,#9510,#9511,#9512,
#9513,#9514,#9515));
#1844=EDGE_LOOP('',(#9516,#9517,#9518,#9519));
#1845=EDGE_LOOP('',(#9520,#9521,#9522,#9523));
#1846=EDGE_LOOP('',(#9524,#9525,#9526,#9527));
#1847=EDGE_LOOP('',(#9528,#9529,#9530,#9531));
#1848=EDGE_LOOP('',(#9532,#9533,#9534,#9535));
#1849=EDGE_LOOP('',(#9536,#9537,#9538,#9539));
#1850=EDGE_LOOP('',(#9540,#9541,#9542,#9543));
#1851=EDGE_LOOP('',(#9544,#9545,#9546,#9547));
#1852=EDGE_LOOP('',(#9548,#9549,#9550,#9551));
#1853=EDGE_LOOP('',(#9552,#9553,#9554,#9555));
#1854=EDGE_LOOP('',(#9556,#9557,#9558,#9559));
#1855=EDGE_LOOP('',(#9560,#9561,#9562,#9563));
#1856=EDGE_LOOP('',(#9564,#9565,#9566,#9567,#9568,#9569,#9570,#9571,#9572,
#9573,#9574,#9575));
#1857=EDGE_LOOP('',(#9576,#9577,#9578,#9579,#9580,#9581,#9582,#9583,#9584,
#9585,#9586,#9587));
#1858=EDGE_LOOP('',(#9588,#9589,#9590,#9591));
#1859=EDGE_LOOP('',(#9592,#9593,#9594,#9595));
#1860=EDGE_LOOP('',(#9596,#9597,#9598,#9599));
#1861=EDGE_LOOP('',(#9600,#9601,#9602,#9603));
#1862=EDGE_LOOP('',(#9604,#9605,#9606,#9607));
#1863=EDGE_LOOP('',(#9608,#9609,#9610,#9611));
#1864=EDGE_LOOP('',(#9612,#9613,#9614,#9615));
#1865=EDGE_LOOP('',(#9616,#9617,#9618,#9619));
#1866=EDGE_LOOP('',(#9620,#9621,#9622,#9623));
#1867=EDGE_LOOP('',(#9624,#9625,#9626,#9627));
#1868=EDGE_LOOP('',(#9628,#9629,#9630,#9631));
#1869=EDGE_LOOP('',(#9632,#9633,#9634,#9635));
#1870=EDGE_LOOP('',(#9636,#9637,#9638,#9639,#9640,#9641,#9642,#9643,#9644,
#9645,#9646,#9647));
#1871=EDGE_LOOP('',(#9648,#9649,#9650,#9651,#9652,#9653,#9654,#9655,#9656,
#9657,#9658,#9659));
#1872=EDGE_LOOP('',(#9660,#9661,#9662,#9663,#9664,#9665,#9666,#9667,#9668,
#9669,#9670,#9671));
#1873=EDGE_LOOP('',(#9672,#9673,#9674,#9675));
#1874=EDGE_LOOP('',(#9676,#9677,#9678,#9679));
#1875=EDGE_LOOP('',(#9680,#9681,#9682,#9683));
#1876=EDGE_LOOP('',(#9684,#9685,#9686,#9687));
#1877=EDGE_LOOP('',(#9688,#9689,#9690,#9691));
#1878=EDGE_LOOP('',(#9692,#9693,#9694,#9695));
#1879=EDGE_LOOP('',(#9696,#9697,#9698,#9699));
#1880=EDGE_LOOP('',(#9700,#9701,#9702,#9703));
#1881=EDGE_LOOP('',(#9704,#9705,#9706,#9707));
#1882=EDGE_LOOP('',(#9708,#9709,#9710,#9711));
#1883=EDGE_LOOP('',(#9712,#9713,#9714,#9715));
#1884=EDGE_LOOP('',(#9716,#9717,#9718,#9719));
#1885=EDGE_LOOP('',(#9720,#9721,#9722,#9723,#9724,#9725,#9726,#9727,#9728,
#9729,#9730,#9731));
#1886=EDGE_LOOP('',(#9732,#9733,#9734,#9735));
#1887=EDGE_LOOP('',(#9736,#9737,#9738,#9739));
#1888=EDGE_LOOP('',(#9740,#9741,#9742,#9743));
#1889=EDGE_LOOP('',(#9744,#9745,#9746,#9747));
#1890=EDGE_LOOP('',(#9748,#9749,#9750,#9751));
#1891=EDGE_LOOP('',(#9752,#9753,#9754,#9755));
#1892=EDGE_LOOP('',(#9756,#9757,#9758,#9759));
#1893=EDGE_LOOP('',(#9760,#9761,#9762,#9763));
#1894=EDGE_LOOP('',(#9764,#9765,#9766,#9767));
#1895=EDGE_LOOP('',(#9768,#9769,#9770,#9771));
#1896=EDGE_LOOP('',(#9772,#9773,#9774,#9775));
#1897=EDGE_LOOP('',(#9776,#9777,#9778,#9779));
#1898=EDGE_LOOP('',(#9780,#9781,#9782,#9783,#9784,#9785,#9786,#9787,#9788,
#9789,#9790,#9791));
#1899=EDGE_LOOP('',(#9792,#9793,#9794,#9795,#9796,#9797,#9798,#9799,#9800,
#9801,#9802,#9803));
#1900=EDGE_LOOP('',(#9804,#9805,#9806,#9807,#9808,#9809,#9810,#9811,#9812,
#9813,#9814,#9815));
#1901=EDGE_LOOP('',(#9816,#9817,#9818,#9819));
#1902=EDGE_LOOP('',(#9820,#9821,#9822,#9823));
#1903=EDGE_LOOP('',(#9824,#9825,#9826,#9827));
#1904=EDGE_LOOP('',(#9828,#9829,#9830,#9831));
#1905=EDGE_LOOP('',(#9832,#9833,#9834,#9835));
#1906=EDGE_LOOP('',(#9836,#9837,#9838,#9839));
#1907=EDGE_LOOP('',(#9840,#9841,#9842,#9843));
#1908=EDGE_LOOP('',(#9844,#9845,#9846,#9847));
#1909=EDGE_LOOP('',(#9848,#9849,#9850,#9851));
#1910=EDGE_LOOP('',(#9852,#9853,#9854,#9855));
#1911=EDGE_LOOP('',(#9856,#9857,#9858,#9859));
#1912=EDGE_LOOP('',(#9860,#9861,#9862,#9863));
#1913=EDGE_LOOP('',(#9864,#9865,#9866,#9867,#9868,#9869,#9870,#9871,#9872,
#9873,#9874,#9875));
#1914=EDGE_LOOP('',(#9876,#9877,#9878,#9879,#9880,#9881,#9882,#9883,#9884,
#9885,#9886,#9887));
#1915=EDGE_LOOP('',(#9888,#9889,#9890,#9891));
#1916=EDGE_LOOP('',(#9892,#9893,#9894,#9895));
#1917=EDGE_LOOP('',(#9896,#9897,#9898,#9899));
#1918=EDGE_LOOP('',(#9900,#9901,#9902,#9903));
#1919=EDGE_LOOP('',(#9904,#9905,#9906,#9907));
#1920=EDGE_LOOP('',(#9908,#9909,#9910,#9911));
#1921=EDGE_LOOP('',(#9912,#9913,#9914,#9915));
#1922=EDGE_LOOP('',(#9916,#9917,#9918,#9919));
#1923=EDGE_LOOP('',(#9920,#9921,#9922,#9923));
#1924=EDGE_LOOP('',(#9924,#9925,#9926,#9927));
#1925=EDGE_LOOP('',(#9928,#9929,#9930,#9931));
#1926=EDGE_LOOP('',(#9932,#9933,#9934,#9935));
#1927=EDGE_LOOP('',(#9936,#9937,#9938,#9939,#9940,#9941,#9942,#9943,#9944,
#9945,#9946,#9947));
#1928=EDGE_LOOP('',(#9948,#9949,#9950,#9951,#9952,#9953,#9954,#9955,#9956,
#9957,#9958,#9959));
#1929=EDGE_LOOP('',(#9960,#9961,#9962,#9963));
#1930=EDGE_LOOP('',(#9964,#9965,#9966,#9967));
#1931=EDGE_LOOP('',(#9968,#9969,#9970,#9971));
#1932=EDGE_LOOP('',(#9972,#9973,#9974,#9975));
#1933=EDGE_LOOP('',(#9976,#9977,#9978,#9979));
#1934=EDGE_LOOP('',(#9980,#9981,#9982,#9983));
#1935=EDGE_LOOP('',(#9984,#9985,#9986,#9987));
#1936=EDGE_LOOP('',(#9988,#9989,#9990,#9991));
#1937=EDGE_LOOP('',(#9992,#9993,#9994,#9995));
#1938=EDGE_LOOP('',(#9996,#9997,#9998,#9999));
#1939=EDGE_LOOP('',(#10000,#10001,#10002,#10003));
#1940=EDGE_LOOP('',(#10004,#10005,#10006,#10007));
#1941=EDGE_LOOP('',(#10008,#10009,#10010,#10011,#10012,#10013,#10014,#10015,
#10016,#10017,#10018,#10019));
#1942=EDGE_LOOP('',(#10020,#10021,#10022,#10023));
#1943=EDGE_LOOP('',(#10024,#10025,#10026,#10027));
#1944=EDGE_LOOP('',(#10028,#10029,#10030,#10031));
#1945=EDGE_LOOP('',(#10032,#10033,#10034,#10035));
#1946=EDGE_LOOP('',(#10036,#10037,#10038,#10039));
#1947=EDGE_LOOP('',(#10040,#10041,#10042,#10043));
#1948=EDGE_LOOP('',(#10044,#10045,#10046,#10047));
#1949=EDGE_LOOP('',(#10048,#10049,#10050,#10051));
#1950=EDGE_LOOP('',(#10052,#10053,#10054,#10055));
#1951=EDGE_LOOP('',(#10056,#10057,#10058,#10059,#10060,#10061,#10062,#10063,
#10064));
#1952=EDGE_LOOP('',(#10065,#10066,#10067,#10068,#10069,#10070,#10071,#10072,
#10073));
#1953=EDGE_LOOP('',(#10074,#10075,#10076,#10077));
#1954=EDGE_LOOP('',(#10078,#10079,#10080,#10081));
#1955=EDGE_LOOP('',(#10082,#10083,#10084,#10085));
#1956=EDGE_LOOP('',(#10086,#10087,#10088,#10089));
#1957=EDGE_LOOP('',(#10090,#10091,#10092,#10093));
#1958=EDGE_LOOP('',(#10094,#10095,#10096,#10097));
#1959=EDGE_LOOP('',(#10098,#10099,#10100,#10101));
#1960=EDGE_LOOP('',(#10102,#10103,#10104,#10105));
#1961=EDGE_LOOP('',(#10106,#10107,#10108,#10109));
#1962=EDGE_LOOP('',(#10110,#10111,#10112,#10113,#10114,#10115,#10116,#10117,
#10118));
#1963=EDGE_LOOP('',(#10119,#10120,#10121,#10122,#10123,#10124,#10125,#10126,
#10127));
#1964=EDGE_LOOP('',(#10128,#10129,#10130,#10131));
#1965=EDGE_LOOP('',(#10132,#10133,#10134,#10135));
#1966=EDGE_LOOP('',(#10136,#10137,#10138,#10139));
#1967=EDGE_LOOP('',(#10140,#10141,#10142,#10143));
#1968=EDGE_LOOP('',(#10144,#10145,#10146,#10147));
#1969=EDGE_LOOP('',(#10148,#10149,#10150,#10151));
#1970=EDGE_LOOP('',(#10152,#10153,#10154,#10155));
#1971=EDGE_LOOP('',(#10156,#10157,#10158,#10159));
#1972=EDGE_LOOP('',(#10160,#10161,#10162,#10163));
#1973=EDGE_LOOP('',(#10164,#10165,#10166,#10167,#10168,#10169,#10170,#10171,
#10172));
#1974=EDGE_LOOP('',(#10173,#10174,#10175,#10176,#10177,#10178,#10179,#10180,
#10181));
#1975=EDGE_LOOP('',(#10182,#10183,#10184,#10185));
#1976=EDGE_LOOP('',(#10186,#10187,#10188,#10189));
#1977=EDGE_LOOP('',(#10190,#10191,#10192,#10193));
#1978=EDGE_LOOP('',(#10194,#10195,#10196,#10197));
#1979=EDGE_LOOP('',(#10198,#10199,#10200,#10201));
#1980=EDGE_LOOP('',(#10202,#10203,#10204,#10205));
#1981=EDGE_LOOP('',(#10206,#10207,#10208,#10209));
#1982=EDGE_LOOP('',(#10210,#10211,#10212,#10213));
#1983=EDGE_LOOP('',(#10214,#10215,#10216,#10217));
#1984=EDGE_LOOP('',(#10218,#10219,#10220,#10221,#10222,#10223,#10224,#10225,
#10226));
#1985=EDGE_LOOP('',(#10227,#10228,#10229,#10230,#10231,#10232,#10233,#10234,
#10235));
#1986=EDGE_LOOP('',(#10236,#10237,#10238,#10239,#10240,#10241,#10242,#10243,
#10244));
#1987=EDGE_LOOP('',(#10245,#10246,#10247,#10248));
#1988=EDGE_LOOP('',(#10249,#10250,#10251,#10252));
#1989=EDGE_LOOP('',(#10253,#10254,#10255,#10256));
#1990=EDGE_LOOP('',(#10257,#10258,#10259,#10260));
#1991=EDGE_LOOP('',(#10261,#10262,#10263,#10264));
#1992=EDGE_LOOP('',(#10265,#10266,#10267,#10268));
#1993=EDGE_LOOP('',(#10269,#10270,#10271,#10272));
#1994=EDGE_LOOP('',(#10273,#10274,#10275,#10276));
#1995=EDGE_LOOP('',(#10277,#10278,#10279,#10280));
#1996=EDGE_LOOP('',(#10281,#10282,#10283,#10284,#10285,#10286,#10287,#10288,
#10289));
#1997=EDGE_LOOP('',(#10290,#10291,#10292,#10293));
#1998=EDGE_LOOP('',(#10294,#10295,#10296,#10297));
#1999=EDGE_LOOP('',(#10298,#10299,#10300,#10301));
#2000=EDGE_LOOP('',(#10302,#10303,#10304,#10305));
#2001=EDGE_LOOP('',(#10306,#10307,#10308,#10309));
#2002=EDGE_LOOP('',(#10310,#10311,#10312,#10313));
#2003=EDGE_LOOP('',(#10314,#10315,#10316,#10317));
#2004=EDGE_LOOP('',(#10318,#10319,#10320,#10321));
#2005=EDGE_LOOP('',(#10322,#10323,#10324,#10325));
#2006=EDGE_LOOP('',(#10326,#10327,#10328,#10329,#10330,#10331,#10332,#10333,
#10334));
#2007=EDGE_LOOP('',(#10335,#10336,#10337,#10338,#10339,#10340,#10341,#10342,
#10343));
#2008=EDGE_LOOP('',(#10344,#10345,#10346,#10347,#10348,#10349,#10350,#10351,
#10352));
#2009=EDGE_LOOP('',(#10353,#10354,#10355,#10356));
#2010=EDGE_LOOP('',(#10357,#10358,#10359,#10360));
#2011=EDGE_LOOP('',(#10361,#10362,#10363,#10364));
#2012=EDGE_LOOP('',(#10365,#10366,#10367,#10368));
#2013=EDGE_LOOP('',(#10369,#10370,#10371,#10372));
#2014=EDGE_LOOP('',(#10373,#10374,#10375,#10376));
#2015=EDGE_LOOP('',(#10377,#10378,#10379,#10380));
#2016=EDGE_LOOP('',(#10381,#10382,#10383,#10384));
#2017=EDGE_LOOP('',(#10385,#10386,#10387,#10388));
#2018=EDGE_LOOP('',(#10389,#10390,#10391,#10392,#10393,#10394,#10395,#10396,
#10397));
#2019=EDGE_LOOP('',(#10398,#10399,#10400,#10401,#10402,#10403,#10404,#10405,
#10406));
#2020=EDGE_LOOP('',(#10407,#10408,#10409,#10410));
#2021=EDGE_LOOP('',(#10411,#10412,#10413,#10414));
#2022=EDGE_LOOP('',(#10415,#10416,#10417,#10418));
#2023=EDGE_LOOP('',(#10419,#10420,#10421,#10422));
#2024=EDGE_LOOP('',(#10423,#10424,#10425,#10426));
#2025=EDGE_LOOP('',(#10427,#10428,#10429,#10430));
#2026=EDGE_LOOP('',(#10431,#10432,#10433,#10434));
#2027=EDGE_LOOP('',(#10435,#10436,#10437,#10438));
#2028=EDGE_LOOP('',(#10439,#10440,#10441,#10442));
#2029=EDGE_LOOP('',(#10443,#10444,#10445,#10446,#10447,#10448,#10449,#10450,
#10451));
#2030=EDGE_LOOP('',(#10452,#10453,#10454,#10455));
#2031=EDGE_LOOP('',(#10456,#10457,#10458,#10459));
#2032=EDGE_LOOP('',(#10460,#10461,#10462,#10463));
#2033=EDGE_LOOP('',(#10464,#10465,#10466,#10467));
#2034=EDGE_LOOP('',(#10468,#10469,#10470,#10471));
#2035=EDGE_LOOP('',(#10472,#10473,#10474,#10475));
#2036=EDGE_LOOP('',(#10476,#10477,#10478,#10479));
#2037=EDGE_LOOP('',(#10480,#10481,#10482,#10483));
#2038=EDGE_LOOP('',(#10484,#10485,#10486,#10487));
#2039=EDGE_LOOP('',(#10488,#10489,#10490,#10491,#10492,#10493,#10494,#10495,
#10496));
#2040=EDGE_LOOP('',(#10497,#10498,#10499,#10500,#10501,#10502,#10503,#10504,
#10505));
#2041=EDGE_LOOP('',(#10506,#10507,#10508,#10509,#10510,#10511,#10512,#10513,
#10514));
#2042=EDGE_LOOP('',(#10515,#10516,#10517,#10518));
#2043=EDGE_LOOP('',(#10519,#10520,#10521,#10522));
#2044=EDGE_LOOP('',(#10523,#10524,#10525,#10526));
#2045=EDGE_LOOP('',(#10527,#10528,#10529,#10530));
#2046=EDGE_LOOP('',(#10531,#10532,#10533,#10534));
#2047=EDGE_LOOP('',(#10535,#10536,#10537,#10538));
#2048=EDGE_LOOP('',(#10539,#10540,#10541,#10542));
#2049=EDGE_LOOP('',(#10543,#10544,#10545,#10546));
#2050=EDGE_LOOP('',(#10547,#10548,#10549,#10550));
#2051=EDGE_LOOP('',(#10551,#10552,#10553,#10554,#10555,#10556,#10557,#10558,
#10559));
#2052=EDGE_LOOP('',(#10560,#10561,#10562,#10563));
#2053=EDGE_LOOP('',(#10564,#10565,#10566,#10567));
#2054=EDGE_LOOP('',(#10568,#10569,#10570,#10571));
#2055=EDGE_LOOP('',(#10572,#10573,#10574,#10575));
#2056=EDGE_LOOP('',(#10576,#10577,#10578,#10579));
#2057=EDGE_LOOP('',(#10580,#10581,#10582,#10583));
#2058=EDGE_LOOP('',(#10584,#10585,#10586,#10587));
#2059=EDGE_LOOP('',(#10588,#10589,#10590,#10591));
#2060=EDGE_LOOP('',(#10592,#10593,#10594,#10595,#10596,#10597,#10598,#10599));
#2061=EDGE_LOOP('',(#10600,#10601,#10602,#10603));
#2062=EDGE_LOOP('',(#10604,#10605,#10606,#10607));
#2063=EDGE_LOOP('',(#10608,#10609,#10610,#10611));
#2064=EDGE_LOOP('',(#10612,#10613,#10614,#10615));
#2065=EDGE_LOOP('',(#10616,#10617,#10618,#10619,#10620,#10621,#10622,#10623));
#2066=EDGE_LOOP('',(#10624,#10625,#10626,#10627));
#2067=EDGE_LOOP('',(#10628,#10629,#10630,#10631));
#2068=EDGE_LOOP('',(#10632,#10633,#10634,#10635));
#2069=EDGE_LOOP('',(#10636,#10637,#10638,#10639));
#2070=EDGE_LOOP('',(#10640,#10641,#10642,#10643));
#2071=EDGE_LOOP('',(#10644,#10645,#10646,#10647));
#2072=EDGE_LOOP('',(#10648,#10649,#10650,#10651));
#2073=EDGE_LOOP('',(#10652,#10653,#10654,#10655));
#2074=EDGE_LOOP('',(#10656,#10657,#10658,#10659));
#2075=EDGE_LOOP('',(#10660,#10661,#10662,#10663));
#2076=EDGE_LOOP('',(#10664,#10665,#10666,#10667));
#2077=EDGE_LOOP('',(#10668,#10669,#10670,#10671));
#2078=EDGE_LOOP('',(#10672,#10673,#10674,#10675));
#2079=EDGE_LOOP('',(#10676,#10677,#10678,#10679));
#2080=EDGE_LOOP('',(#10680,#10681,#10682,#10683));
#2081=EDGE_LOOP('',(#10684,#10685,#10686,#10687));
#2082=EDGE_LOOP('',(#10688,#10689,#10690,#10691));
#2083=EDGE_LOOP('',(#10692,#10693,#10694,#10695));
#2084=EDGE_LOOP('',(#10696,#10697,#10698,#10699));
#2085=EDGE_LOOP('',(#10700,#10701,#10702,#10703));
#2086=EDGE_LOOP('',(#10704,#10705,#10706,#10707));
#2087=EDGE_LOOP('',(#10708,#10709,#10710,#10711));
#2088=EDGE_LOOP('',(#10712,#10713,#10714,#10715));
#2089=EDGE_LOOP('',(#10716,#10717,#10718,#10719));
#2090=EDGE_LOOP('',(#10720,#10721,#10722,#10723));
#2091=EDGE_LOOP('',(#10724,#10725,#10726,#10727));
#2092=EDGE_LOOP('',(#10728,#10729,#10730,#10731));
#2093=EDGE_LOOP('',(#10732,#10733,#10734,#10735));
#2094=EDGE_LOOP('',(#10736));
#2095=EDGE_LOOP('',(#10737));
#2096=EDGE_LOOP('',(#10738,#10739,#10740,#10741));
#2097=EDGE_LOOP('',(#10742,#10743,#10744,#10745));
#2098=EDGE_LOOP('',(#10746,#10747,#10748,#10749));
#2099=EDGE_LOOP('',(#10750,#10751,#10752,#10753));
#2100=EDGE_LOOP('',(#10754,#10755,#10756,#10757));
#2101=EDGE_LOOP('',(#10758,#10759,#10760,#10761));
#2102=EDGE_LOOP('',(#10762));
#2103=EDGE_LOOP('',(#10763));
#2104=EDGE_LOOP('',(#10764,#10765,#10766,#10767,#10768,#10769,#10770,#10771,
#10772,#10773,#10774,#10775));
#2105=EDGE_LOOP('',(#10776,#10777,#10778,#10779,#10780,#10781,#10782,#10783,
#10784,#10785,#10786,#10787));
#2106=EDGE_LOOP('',(#10788,#10789,#10790,#10791));
#2107=EDGE_LOOP('',(#10792,#10793,#10794,#10795));
#2108=EDGE_LOOP('',(#10796,#10797,#10798,#10799));
#2109=EDGE_LOOP('',(#10800));
#2110=EDGE_LOOP('',(#10801));
#2111=EDGE_LOOP('',(#10802,#10803,#10804,#10805));
#2112=EDGE_LOOP('',(#10806,#10807,#10808,#10809));
#2113=EDGE_LOOP('',(#10810,#10811,#10812,#10813));
#2114=EDGE_LOOP('',(#10814));
#2115=EDGE_LOOP('',(#10815));
#2116=EDGE_LOOP('',(#10816,#10817,#10818,#10819));
#2117=EDGE_LOOP('',(#10820,#10821,#10822,#10823));
#2118=EDGE_LOOP('',(#10824,#10825,#10826,#10827));
#2119=EDGE_LOOP('',(#10828,#10829,#10830,#10831));
#2120=EDGE_LOOP('',(#10832,#10833,#10834,#10835));
#2121=EDGE_LOOP('',(#10836,#10837,#10838,#10839,#10840,#10841,#10842,#10843,
#10844));
#2122=EDGE_LOOP('',(#10845,#10846,#10847,#10848,#10849,#10850,#10851,#10852,
#10853));
#2123=EDGE_LOOP('',(#10854,#10855,#10856,#10857));
#2124=EDGE_LOOP('',(#10858,#10859,#10860,#10861));
#2125=EDGE_LOOP('',(#10862,#10863,#10864,#10865));
#2126=EDGE_LOOP('',(#10866));
#2127=EDGE_LOOP('',(#10867));
#2128=EDGE_LOOP('',(#10868,#10869,#10870,#10871));
#2129=EDGE_LOOP('',(#10872,#10873,#10874,#10875));
#2130=EDGE_LOOP('',(#10876,#10877,#10878,#10879));
#2131=EDGE_LOOP('',(#10880));
#2132=EDGE_LOOP('',(#10881));
#2133=EDGE_LOOP('',(#10882,#10883,#10884,#10885));
#2134=EDGE_LOOP('',(#10886,#10887,#10888,#10889));
#2135=EDGE_LOOP('',(#10890,#10891,#10892,#10893));
#2136=EDGE_LOOP('',(#10894,#10895,#10896,#10897));
#2137=EDGE_LOOP('',(#10898,#10899,#10900,#10901));
#2138=EDGE_LOOP('',(#10902,#10903,#10904,#10905,#10906,#10907,#10908,#10909,
#10910));
#2139=EDGE_LOOP('',(#10911,#10912,#10913,#10914,#10915,#10916,#10917,#10918,
#10919));
#2572=CIRCLE('',#12670,2.54);
#2573=CIRCLE('',#12671,2.54);
#2574=CIRCLE('',#12674,6.85800000000002);
#2575=CIRCLE('',#12675,6.85800000000002);
#2576=CIRCLE('',#12678,6.85800000000002);
#2577=CIRCLE('',#12679,6.85800000000001);
#2578=CIRCLE('',#12682,2.54);
#2579=CIRCLE('',#12683,2.54);
#2580=CIRCLE('',#12690,2.53999999999999);
#2581=CIRCLE('',#12691,6.85800000000003);
#2582=CIRCLE('',#12692,6.85800000000003);
#2583=CIRCLE('',#12693,2.53999999999999);
#2584=CIRCLE('',#12736,2.54);
#2585=CIRCLE('',#12740,6.858);
#2586=CIRCLE('',#12744,6.85800000000002);
#2587=CIRCLE('',#12748,2.53999999999999);
#2588=CIRCLE('',#12758,2.53999999999999);
#2589=CIRCLE('',#12759,2.53999999999999);
#2590=CIRCLE('',#12762,6.85799999999992);
#2591=CIRCLE('',#12763,6.85799999999992);
#2592=CIRCLE('',#12766,6.85799999999992);
#2593=CIRCLE('',#12767,6.85799999999992);
#2594=CIRCLE('',#12770,2.53999999999999);
#2595=CIRCLE('',#12771,2.53999999999999);
#2596=CIRCLE('',#12778,2.53999999999999);
#2597=CIRCLE('',#12779,6.85800000000003);
#2598=CIRCLE('',#12780,6.85800000000003);
#2599=CIRCLE('',#12781,2.53999999999999);
#2600=CIRCLE('',#12803,2.54);
#2601=CIRCLE('',#12807,6.85800000000003);
#2602=CIRCLE('',#12811,6.85800000000003);
#2603=CIRCLE('',#12815,2.53999999999999);
#2604=CIRCLE('',#12844,2.53999999999999);
#2605=CIRCLE('',#12845,6.85800000000003);
#2606=CIRCLE('',#12846,6.858);
#2607=CIRCLE('',#12847,2.53999999999999);
#2608=CIRCLE('',#12866,2.53999999999999);
#2609=CIRCLE('',#12867,6.858);
#2610=CIRCLE('',#12868,6.85800000000003);
#2611=CIRCLE('',#12869,2.53999999999999);
#2612=CIRCLE('',#12890,3.16991999999999);
#2613=CIRCLE('',#12891,3.16991999999999);
#2614=CIRCLE('',#12894,4.7625);
#2615=CIRCLE('',#12895,4.7625);
#2616=CIRCLE('',#12898,3.16991999999999);
#2617=CIRCLE('',#12899,3.16991999999999);
#2618=CIRCLE('',#12907,3.16991999999999);
#2619=CIRCLE('',#12908,3.16991999999999);
#2620=CIRCLE('',#12911,4.7625);
#2621=CIRCLE('',#12912,4.7625);
#2622=CIRCLE('',#12915,3.16991999999999);
#2623=CIRCLE('',#12916,3.16991999999999);
#2624=CIRCLE('',#12924,3.16991999999999);
#2625=CIRCLE('',#12925,3.16991999999999);
#2626=CIRCLE('',#12928,4.7625);
#2627=CIRCLE('',#12929,4.7625);
#2628=CIRCLE('',#12932,3.16991999999999);
#2629=CIRCLE('',#12933,3.16991999999999);
#2630=CIRCLE('',#12941,3.16991999999999);
#2631=CIRCLE('',#12942,3.16991999999999);
#2632=CIRCLE('',#12945,4.7625);
#2633=CIRCLE('',#12946,4.7625);
#2634=CIRCLE('',#12949,3.16991999999999);
#2635=CIRCLE('',#12950,3.16991999999999);
#2636=CIRCLE('',#12956,3.16991999999999);
#2637=CIRCLE('',#12957,4.7625);
#2638=CIRCLE('',#12958,3.16991999999998);
#2639=CIRCLE('',#12990,3.16991999999996);
#2640=CIRCLE('',#12991,4.7625);
#2641=CIRCLE('',#12992,3.16991999999999);
#2642=CIRCLE('',#13007,3.16991999999996);
#2643=CIRCLE('',#13008,4.7625);
#2644=CIRCLE('',#13009,3.16991999999999);
#2645=CIRCLE('',#13041,3.16991999999999);
#2646=CIRCLE('',#13042,4.7625);
#2647=CIRCLE('',#13043,3.16991999999996);
#2648=CIRCLE('',#13058,4.50000000000006);
#2649=CIRCLE('',#13059,4.49999999999995);
#2650=CIRCLE('',#13061,4.49999999999995);
#2651=CIRCLE('',#13062,4.50000000000006);
#2652=CIRCLE('',#13064,4.49999999999995);
#2653=CIRCLE('',#13065,4.49999999999995);
#2654=CIRCLE('',#13067,4.49999999999995);
#2655=CIRCLE('',#13068,4.49999999999995);
#2656=CIRCLE('',#13074,4.49999999999995);
#2657=CIRCLE('',#13075,4.50000000000006);
#2658=CIRCLE('',#13076,4.49999999999995);
#2659=CIRCLE('',#13077,4.49999999999995);
#2660=CIRCLE('',#13079,4.50000000000006);
#2661=CIRCLE('',#13080,4.49999999999995);
#2662=CIRCLE('',#13081,4.49999999999995);
#2663=CIRCLE('',#13082,4.49999999999995);
#2664=CIRCLE('',#13100,8.74999999999998);
#2665=CIRCLE('',#13101,8.74999999999998);
#2666=CIRCLE('',#13103,8.74999999999998);
#2667=CIRCLE('',#13104,8.74999999999998);
#2668=CIRCLE('',#13128,4.5);
#2669=CIRCLE('',#13129,4.5);
#2670=CIRCLE('',#13131,4.5);
#2671=CIRCLE('',#13132,4.5);
#2672=CIRCLE('',#13136,3.16991999999999);
#2673=CIRCLE('',#13137,3.16991999999999);
#2674=CIRCLE('',#13140,4.7625);
#2675=CIRCLE('',#13141,4.7625);
#2676=CIRCLE('',#13144,3.16991999999999);
#2677=CIRCLE('',#13145,3.16991999999999);
#2678=CIRCLE('',#13151,4.5);
#2679=CIRCLE('',#13152,4.5);
#2680=CIRCLE('',#13154,4.5);
#2681=CIRCLE('',#13155,4.5);
#2682=CIRCLE('',#13159,3.16991999999999);
#2683=CIRCLE('',#13160,3.16991999999999);
#2684=CIRCLE('',#13163,4.7625);
#2685=CIRCLE('',#13164,4.7625);
#2686=CIRCLE('',#13167,3.16991999999999);
#2687=CIRCLE('',#13168,3.16991999999999);
#3134=LINE('',#25861,#4146);
#3135=LINE('',#25863,#4147);
#3136=LINE('',#25865,#4148);
#3137=LINE('',#25866,#4149);
#3138=LINE('',#25869,#4150);
#3139=LINE('',#25871,#4151);
#3140=LINE('',#25872,#4152);
#3141=LINE('',#25877,#4153);
#3142=LINE('',#25881,#4154);
#3143=LINE('',#25883,#4155);
#3144=LINE('',#25884,#4156);
#3145=LINE('',#25889,#4157);
#3146=LINE('',#25893,#4158);
#3147=LINE('',#25895,#4159);
#3148=LINE('',#25896,#4160);
#3149=LINE('',#25901,#4161);
#3150=LINE('',#25905,#4162);
#3151=LINE('',#25907,#4163);
#3152=LINE('',#25908,#4164);
#3153=LINE('',#25913,#4165);
#3154=LINE('',#25917,#4166);
#3155=LINE('',#25919,#4167);
#3156=LINE('',#25920,#4168);
#3157=LINE('',#25923,#4169);
#3158=LINE('',#25925,#4170);
#3159=LINE('',#25926,#4171);
#3160=LINE('',#25928,#4172);
#3161=LINE('',#25929,#4173);
#3162=LINE('',#25935,#4174);
#3163=LINE('',#25939,#4175);
#3164=LINE('',#25943,#4176);
#3165=LINE('',#25947,#4177);
#3166=LINE('',#25951,#4178);
#3167=LINE('',#25953,#4179);
#3168=LINE('',#25955,#4180);
#3169=LINE('',#25956,#4181);
#3170=LINE('',#25959,#4182);
#3171=LINE('',#25961,#4183);
#3172=LINE('',#25962,#4184);
#3173=LINE('',#25965,#4185);
#3174=LINE('',#25966,#4186);
#3175=LINE('',#25969,#4187);
#3176=LINE('',#25970,#4188);
#3177=LINE('',#25973,#4189);
#3178=LINE('',#25977,#4190);
#3179=LINE('',#25978,#4191);
#3180=LINE('',#25981,#4192);
#3181=LINE('',#25985,#4193);
#3182=LINE('',#25986,#4194);
#3183=LINE('',#25989,#4195);
#3184=LINE('',#25993,#4196);
#3185=LINE('',#25994,#4197);
#3186=LINE('',#25997,#4198);
#3187=LINE('',#26001,#4199);
#3188=LINE('',#26002,#4200);
#3189=LINE('',#26004,#4201);
#3190=LINE('',#26009,#4202);
#3191=LINE('',#26011,#4203);
#3192=LINE('',#26013,#4204);
#3193=LINE('',#26015,#4205);
#3194=LINE('',#26017,#4206);
#3195=LINE('',#26021,#4207);
#3196=LINE('',#26025,#4208);
#3197=LINE('',#26029,#4209);
#3198=LINE('',#26033,#4210);
#3199=LINE('',#26035,#4211);
#3200=LINE('',#26036,#4212);
#3201=LINE('',#26039,#4213);
#3202=LINE('',#26040,#4214);
#3203=LINE('',#26043,#4215);
#3204=LINE('',#26044,#4216);
#3205=LINE('',#26048,#4217);
#3206=LINE('',#26051,#4218);
#3207=LINE('',#26052,#4219);
#3208=LINE('',#26056,#4220);
#3209=LINE('',#26059,#4221);
#3210=LINE('',#26060,#4222);
#3211=LINE('',#26064,#4223);
#3212=LINE('',#26067,#4224);
#3213=LINE('',#26068,#4225);
#3214=LINE('',#26072,#4226);
#3215=LINE('',#26075,#4227);
#3216=LINE('',#26076,#4228);
#3217=LINE('',#26078,#4229);
#3218=LINE('',#26083,#4230);
#3219=LINE('',#26085,#4231);
#3220=LINE('',#26087,#4232);
#3221=LINE('',#26088,#4233);
#3222=LINE('',#26091,#4234);
#3223=LINE('',#26093,#4235);
#3224=LINE('',#26094,#4236);
#3225=LINE('',#26100,#4237);
#3226=LINE('',#26103,#4238);
#3227=LINE('',#26105,#4239);
#3228=LINE('',#26106,#4240);
#3229=LINE('',#26112,#4241);
#3230=LINE('',#26115,#4242);
#3231=LINE('',#26117,#4243);
#3232=LINE('',#26118,#4244);
#3233=LINE('',#26124,#4245);
#3234=LINE('',#26127,#4246);
#3235=LINE('',#26129,#4247);
#3236=LINE('',#26130,#4248);
#3237=LINE('',#26136,#4249);
#3238=LINE('',#26139,#4250);
#3239=LINE('',#26141,#4251);
#3240=LINE('',#26142,#4252);
#3241=LINE('',#26145,#4253);
#3242=LINE('',#26147,#4254);
#3243=LINE('',#26148,#4255);
#3244=LINE('',#26150,#4256);
#3245=LINE('',#26151,#4257);
#3246=LINE('',#26157,#4258);
#3247=LINE('',#26159,#4259);
#3248=LINE('',#26161,#4260);
#3249=LINE('',#26162,#4261);
#3250=LINE('',#26165,#4262);
#3251=LINE('',#26167,#4263);
#3252=LINE('',#26168,#4264);
#3253=LINE('',#26173,#4265);
#3254=LINE('',#26177,#4266);
#3255=LINE('',#26179,#4267);
#3256=LINE('',#26180,#4268);
#3257=LINE('',#26185,#4269);
#3258=LINE('',#26189,#4270);
#3259=LINE('',#26191,#4271);
#3260=LINE('',#26192,#4272);
#3261=LINE('',#26197,#4273);
#3262=LINE('',#26201,#4274);
#3263=LINE('',#26203,#4275);
#3264=LINE('',#26204,#4276);
#3265=LINE('',#26209,#4277);
#3266=LINE('',#26213,#4278);
#3267=LINE('',#26215,#4279);
#3268=LINE('',#26216,#4280);
#3269=LINE('',#26219,#4281);
#3270=LINE('',#26221,#4282);
#3271=LINE('',#26222,#4283);
#3272=LINE('',#26224,#4284);
#3273=LINE('',#26225,#4285);
#3274=LINE('',#26231,#4286);
#3275=LINE('',#26233,#4287);
#3276=LINE('',#26235,#4288);
#3277=LINE('',#26237,#4289);
#3278=LINE('',#26239,#4290);
#3279=LINE('',#26243,#4291);
#3280=LINE('',#26247,#4292);
#3281=LINE('',#26251,#4293);
#3282=LINE('',#26255,#4294);
#3283=LINE('',#26257,#4295);
#3284=LINE('',#26258,#4296);
#3285=LINE('',#26261,#4297);
#3286=LINE('',#26262,#4298);
#3287=LINE('',#26265,#4299);
#3288=LINE('',#26266,#4300);
#3289=LINE('',#26270,#4301);
#3290=LINE('',#26273,#4302);
#3291=LINE('',#26274,#4303);
#3292=LINE('',#26278,#4304);
#3293=LINE('',#26281,#4305);
#3294=LINE('',#26282,#4306);
#3295=LINE('',#26286,#4307);
#3296=LINE('',#26289,#4308);
#3297=LINE('',#26290,#4309);
#3298=LINE('',#26294,#4310);
#3299=LINE('',#26297,#4311);
#3300=LINE('',#26298,#4312);
#3301=LINE('',#26300,#4313);
#3302=LINE('',#26305,#4314);
#3303=LINE('',#26307,#4315);
#3304=LINE('',#26309,#4316);
#3305=LINE('',#26310,#4317);
#3306=LINE('',#26313,#4318);
#3307=LINE('',#26315,#4319);
#3308=LINE('',#26316,#4320);
#3309=LINE('',#26321,#4321);
#3310=LINE('',#26325,#4322);
#3311=LINE('',#26327,#4323);
#3312=LINE('',#26328,#4324);
#3313=LINE('',#26333,#4325);
#3314=LINE('',#26337,#4326);
#3315=LINE('',#26339,#4327);
#3316=LINE('',#26340,#4328);
#3317=LINE('',#26345,#4329);
#3318=LINE('',#26349,#4330);
#3319=LINE('',#26351,#4331);
#3320=LINE('',#26352,#4332);
#3321=LINE('',#26357,#4333);
#3322=LINE('',#26361,#4334);
#3323=LINE('',#26363,#4335);
#3324=LINE('',#26364,#4336);
#3325=LINE('',#26367,#4337);
#3326=LINE('',#26369,#4338);
#3327=LINE('',#26370,#4339);
#3328=LINE('',#26372,#4340);
#3329=LINE('',#26373,#4341);
#3330=LINE('',#26379,#4342);
#3331=LINE('',#26381,#4343);
#3332=LINE('',#26383,#4344);
#3333=LINE('',#26385,#4345);
#3334=LINE('',#26387,#4346);
#3335=LINE('',#26391,#4347);
#3336=LINE('',#26395,#4348);
#3337=LINE('',#26399,#4349);
#3338=LINE('',#26403,#4350);
#3339=LINE('',#26405,#4351);
#3340=LINE('',#26406,#4352);
#3341=LINE('',#26409,#4353);
#3342=LINE('',#26410,#4354);
#3343=LINE('',#26413,#4355);
#3344=LINE('',#26414,#4356);
#3345=LINE('',#26418,#4357);
#3346=LINE('',#26421,#4358);
#3347=LINE('',#26422,#4359);
#3348=LINE('',#26426,#4360);
#3349=LINE('',#26429,#4361);
#3350=LINE('',#26430,#4362);
#3351=LINE('',#26434,#4363);
#3352=LINE('',#26437,#4364);
#3353=LINE('',#26438,#4365);
#3354=LINE('',#26442,#4366);
#3355=LINE('',#26445,#4367);
#3356=LINE('',#26446,#4368);
#3357=LINE('',#26448,#4369);
#3358=LINE('',#26453,#4370);
#3359=LINE('',#26455,#4371);
#3360=LINE('',#26459,#4372);
#3361=LINE('',#26463,#4373);
#3362=LINE('',#26467,#4374);
#3363=LINE('',#26471,#4375);
#3364=LINE('',#26473,#4376);
#3365=LINE('',#26474,#4377);
#3366=LINE('',#26477,#4378);
#3367=LINE('',#26479,#4379);
#3368=LINE('',#26480,#4380);
#3369=LINE('',#26483,#4381);
#3370=LINE('',#26484,#4382);
#3371=LINE('',#26487,#4383);
#3372=LINE('',#26488,#4384);
#3373=LINE('',#26491,#4385);
#3374=LINE('',#26495,#4386);
#3375=LINE('',#26496,#4387);
#3376=LINE('',#26499,#4388);
#3377=LINE('',#26503,#4389);
#3378=LINE('',#26504,#4390);
#3379=LINE('',#26507,#4391);
#3380=LINE('',#26511,#4392);
#3381=LINE('',#26512,#4393);
#3382=LINE('',#26515,#4394);
#3383=LINE('',#26519,#4395);
#3384=LINE('',#26520,#4396);
#3385=LINE('',#26522,#4397);
#3386=LINE('',#26527,#4398);
#3387=LINE('',#26529,#4399);
#3388=LINE('',#26531,#4400);
#3389=LINE('',#26533,#4401);
#3390=LINE('',#26537,#4402);
#3391=LINE('',#26541,#4403);
#3392=LINE('',#26545,#4404);
#3393=LINE('',#26548,#4405);
#3394=LINE('',#26551,#4406);
#3395=LINE('',#26553,#4407);
#3396=LINE('',#26554,#4408);
#3397=LINE('',#26557,#4409);
#3398=LINE('',#26558,#4410);
#3399=LINE('',#26561,#4411);
#3400=LINE('',#26562,#4412);
#3401=LINE('',#26566,#4413);
#3402=LINE('',#26569,#4414);
#3403=LINE('',#26570,#4415);
#3404=LINE('',#26574,#4416);
#3405=LINE('',#26577,#4417);
#3406=LINE('',#26578,#4418);
#3407=LINE('',#26582,#4419);
#3408=LINE('',#26585,#4420);
#3409=LINE('',#26586,#4421);
#3410=LINE('',#26590,#4422);
#3411=LINE('',#26593,#4423);
#3412=LINE('',#26594,#4424);
#3413=LINE('',#26596,#4425);
#3414=LINE('',#26601,#4426);
#3415=LINE('',#26603,#4427);
#3416=LINE('',#26605,#4428);
#3417=LINE('',#26606,#4429);
#3418=LINE('',#26609,#4430);
#3419=LINE('',#26611,#4431);
#3420=LINE('',#26612,#4432);
#3421=LINE('',#26617,#4433);
#3422=LINE('',#26621,#4434);
#3423=LINE('',#26623,#4435);
#3424=LINE('',#26624,#4436);
#3425=LINE('',#26629,#4437);
#3426=LINE('',#26633,#4438);
#3427=LINE('',#26635,#4439);
#3428=LINE('',#26636,#4440);
#3429=LINE('',#26641,#4441);
#3430=LINE('',#26645,#4442);
#3431=LINE('',#26647,#4443);
#3432=LINE('',#26648,#4444);
#3433=LINE('',#26650,#4445);
#3434=LINE('',#26651,#4446);
#3435=LINE('',#26657,#4447);
#3436=LINE('',#26659,#4448);
#3437=LINE('',#26661,#4449);
#3438=LINE('',#26662,#4450);
#3439=LINE('',#26665,#4451);
#3440=LINE('',#26667,#4452);
#3441=LINE('',#26668,#4453);
#3442=LINE('',#26673,#4454);
#3443=LINE('',#26677,#4455);
#3444=LINE('',#26679,#4456);
#3445=LINE('',#26680,#4457);
#3446=LINE('',#26685,#4458);
#3447=LINE('',#26689,#4459);
#3448=LINE('',#26691,#4460);
#3449=LINE('',#26692,#4461);
#3450=LINE('',#26697,#4462);
#3451=LINE('',#26701,#4463);
#3452=LINE('',#26703,#4464);
#3453=LINE('',#26704,#4465);
#3454=LINE('',#26706,#4466);
#3455=LINE('',#26707,#4467);
#3456=LINE('',#26713,#4468);
#3457=LINE('',#26715,#4469);
#3458=LINE('',#26717,#4470);
#3459=LINE('',#26718,#4471);
#3460=LINE('',#26721,#4472);
#3461=LINE('',#26723,#4473);
#3462=LINE('',#26724,#4474);
#3463=LINE('',#26730,#4475);
#3464=LINE('',#26733,#4476);
#3465=LINE('',#26735,#4477);
#3466=LINE('',#26736,#4478);
#3467=LINE('',#26742,#4479);
#3468=LINE('',#26745,#4480);
#3469=LINE('',#26747,#4481);
#3470=LINE('',#26748,#4482);
#3471=LINE('',#26754,#4483);
#3472=LINE('',#26757,#4484);
#3473=LINE('',#26759,#4485);
#3474=LINE('',#26760,#4486);
#3475=LINE('',#26762,#4487);
#3476=LINE('',#26763,#4488);
#3477=LINE('',#26769,#4489);
#3478=LINE('',#26771,#4490);
#3479=LINE('',#26773,#4491);
#3480=LINE('',#26774,#4492);
#3481=LINE('',#26777,#4493);
#3482=LINE('',#26779,#4494);
#3483=LINE('',#26780,#4495);
#3484=LINE('',#26786,#4496);
#3485=LINE('',#26789,#4497);
#3486=LINE('',#26791,#4498);
#3487=LINE('',#26792,#4499);
#3488=LINE('',#26798,#4500);
#3489=LINE('',#26801,#4501);
#3490=LINE('',#26803,#4502);
#3491=LINE('',#26804,#4503);
#3492=LINE('',#26810,#4504);
#3493=LINE('',#26813,#4505);
#3494=LINE('',#26815,#4506);
#3495=LINE('',#26816,#4507);
#3496=LINE('',#26818,#4508);
#3497=LINE('',#26819,#4509);
#3498=LINE('',#26825,#4510);
#3499=LINE('',#26827,#4511);
#3500=LINE('',#26831,#4512);
#3501=LINE('',#26835,#4513);
#3502=LINE('',#26839,#4514);
#3503=LINE('',#26840,#4515);
#3504=LINE('',#26843,#4516);
#3505=LINE('',#26845,#4517);
#3506=LINE('',#26846,#4518);
#3507=LINE('',#26849,#4519);
#3508=LINE('',#26850,#4520);
#3509=LINE('',#26853,#4521);
#3510=LINE('',#26857,#4522);
#3511=LINE('',#26858,#4523);
#3512=LINE('',#26861,#4524);
#3513=LINE('',#26865,#4525);
#3514=LINE('',#26866,#4526);
#3515=LINE('',#26869,#4527);
#3516=LINE('',#26873,#4528);
#3517=LINE('',#26874,#4529);
#3518=LINE('',#26876,#4530);
#3519=LINE('',#26881,#4531);
#3520=LINE('',#26883,#4532);
#3521=LINE('',#26885,#4533);
#3522=LINE('',#26886,#4534);
#3523=LINE('',#26889,#4535);
#3524=LINE('',#26891,#4536);
#3525=LINE('',#26892,#4537);
#3526=LINE('',#26897,#4538);
#3527=LINE('',#26901,#4539);
#3528=LINE('',#26903,#4540);
#3529=LINE('',#26904,#4541);
#3530=LINE('',#26909,#4542);
#3531=LINE('',#26913,#4543);
#3532=LINE('',#26915,#4544);
#3533=LINE('',#26916,#4545);
#3534=LINE('',#26921,#4546);
#3535=LINE('',#26925,#4547);
#3536=LINE('',#26927,#4548);
#3537=LINE('',#26928,#4549);
#3538=LINE('',#26930,#4550);
#3539=LINE('',#26931,#4551);
#3540=LINE('',#26937,#4552);
#3541=LINE('',#26939,#4553);
#3542=LINE('',#26941,#4554);
#3543=LINE('',#26945,#4555);
#3544=LINE('',#26949,#4556);
#3545=LINE('',#26952,#4557);
#3546=LINE('',#26955,#4558);
#3547=LINE('',#26957,#4559);
#3548=LINE('',#26958,#4560);
#3549=LINE('',#26961,#4561);
#3550=LINE('',#26962,#4562);
#3551=LINE('',#26966,#4563);
#3552=LINE('',#26969,#4564);
#3553=LINE('',#26970,#4565);
#3554=LINE('',#26974,#4566);
#3555=LINE('',#26977,#4567);
#3556=LINE('',#26978,#4568);
#3557=LINE('',#26982,#4569);
#3558=LINE('',#26985,#4570);
#3559=LINE('',#26986,#4571);
#3560=LINE('',#26988,#4572);
#3561=LINE('',#26993,#4573);
#3562=LINE('',#26995,#4574);
#3563=LINE('',#26997,#4575);
#3564=LINE('',#27001,#4576);
#3565=LINE('',#27005,#4577);
#3566=LINE('',#27008,#4578);
#3567=LINE('',#27011,#4579);
#3568=LINE('',#27013,#4580);
#3569=LINE('',#27014,#4581);
#3570=LINE('',#27017,#4582);
#3571=LINE('',#27018,#4583);
#3572=LINE('',#27022,#4584);
#3573=LINE('',#27025,#4585);
#3574=LINE('',#27026,#4586);
#3575=LINE('',#27030,#4587);
#3576=LINE('',#27033,#4588);
#3577=LINE('',#27034,#4589);
#3578=LINE('',#27038,#4590);
#3579=LINE('',#27041,#4591);
#3580=LINE('',#27042,#4592);
#3581=LINE('',#27044,#4593);
#3582=LINE('',#27049,#4594);
#3583=LINE('',#27051,#4595);
#3584=LINE('',#27053,#4596);
#3585=LINE('',#27054,#4597);
#3586=LINE('',#27057,#4598);
#3587=LINE('',#27059,#4599);
#3588=LINE('',#27060,#4600);
#3589=LINE('',#27066,#4601);
#3590=LINE('',#27069,#4602);
#3591=LINE('',#27071,#4603);
#3592=LINE('',#27072,#4604);
#3593=LINE('',#27078,#4605);
#3594=LINE('',#27081,#4606);
#3595=LINE('',#27083,#4607);
#3596=LINE('',#27084,#4608);
#3597=LINE('',#27090,#4609);
#3598=LINE('',#27093,#4610);
#3599=LINE('',#27095,#4611);
#3600=LINE('',#27096,#4612);
#3601=LINE('',#27098,#4613);
#3602=LINE('',#27099,#4614);
#3603=LINE('',#27105,#4615);
#3604=LINE('',#27107,#4616);
#3605=LINE('',#27111,#4617);
#3606=LINE('',#27115,#4618);
#3607=LINE('',#27119,#4619);
#3608=LINE('',#27120,#4620);
#3609=LINE('',#27123,#4621);
#3610=LINE('',#27125,#4622);
#3611=LINE('',#27126,#4623);
#3612=LINE('',#27129,#4624);
#3613=LINE('',#27130,#4625);
#3614=LINE('',#27133,#4626);
#3615=LINE('',#27137,#4627);
#3616=LINE('',#27138,#4628);
#3617=LINE('',#27141,#4629);
#3618=LINE('',#27145,#4630);
#3619=LINE('',#27146,#4631);
#3620=LINE('',#27149,#4632);
#3621=LINE('',#27153,#4633);
#3622=LINE('',#27154,#4634);
#3623=LINE('',#27156,#4635);
#3624=LINE('',#27163,#4636);
#3625=LINE('',#27166,#4637);
#3626=LINE('',#27172,#4638);
#3627=LINE('',#27175,#4639);
#3628=LINE('',#27181,#4640);
#3629=LINE('',#27184,#4641);
#3630=LINE('',#27190,#4642);
#3631=LINE('',#27193,#4643);
#3632=LINE('',#27197,#4644);
#3633=LINE('',#27199,#4645);
#3634=LINE('',#27201,#4646);
#3635=LINE('',#27202,#4647);
#3636=LINE('',#27206,#4648);
#3637=LINE('',#27208,#4649);
#3638=LINE('',#27210,#4650);
#3639=LINE('',#27211,#4651);
#3640=LINE('',#27215,#4652);
#3641=LINE('',#27217,#4653);
#3642=LINE('',#27219,#4654);
#3643=LINE('',#27220,#4655);
#3644=LINE('',#27224,#4656);
#3645=LINE('',#27226,#4657);
#3646=LINE('',#27228,#4658);
#3647=LINE('',#27229,#4659);
#3648=LINE('',#27231,#4660);
#3649=LINE('',#27232,#4661);
#3650=LINE('',#27233,#4662);
#3651=LINE('',#27234,#4663);
#3652=LINE('',#27236,#4664);
#3653=LINE('',#27238,#4665);
#3654=LINE('',#27241,#4666);
#3655=LINE('',#27243,#4667);
#3656=LINE('',#27246,#4668);
#3657=LINE('',#27248,#4669);
#3658=LINE('',#27251,#4670);
#3659=LINE('',#27253,#4671);
#3660=LINE('',#27256,#4672);
#3661=LINE('',#27257,#4673);
#3662=LINE('',#27258,#4674);
#3663=LINE('',#27259,#4675);
#3664=LINE('',#27261,#4676);
#3665=LINE('',#27264,#4677);
#3666=LINE('',#27266,#4678);
#3667=LINE('',#27269,#4679);
#3668=LINE('',#27271,#4680);
#3669=LINE('',#27274,#4681);
#3670=LINE('',#27276,#4682);
#3671=LINE('',#27279,#4683);
#3672=LINE('',#27281,#4684);
#3673=LINE('',#27283,#4685);
#3674=LINE('',#27286,#4686);
#3675=LINE('',#27288,#4687);
#3676=LINE('',#27291,#4688);
#3677=LINE('',#27293,#4689);
#3678=LINE('',#27296,#4690);
#3679=LINE('',#27298,#4691);
#3680=LINE('',#27308,#4692);
#3681=LINE('',#27314,#4693);
#3682=LINE('',#27319,#4694);
#3683=LINE('',#27321,#4695);
#3684=LINE('',#27323,#4696);
#3685=LINE('',#27324,#4697);
#3686=LINE('',#27327,#4698);
#3687=LINE('',#27329,#4699);
#3688=LINE('',#27330,#4700);
#3689=LINE('',#27335,#4701);
#3690=LINE('',#27339,#4702);
#3691=LINE('',#27341,#4703);
#3692=LINE('',#27342,#4704);
#3693=LINE('',#27347,#4705);
#3694=LINE('',#27351,#4706);
#3695=LINE('',#27353,#4707);
#3696=LINE('',#27354,#4708);
#3697=LINE('',#27359,#4709);
#3698=LINE('',#27363,#4710);
#3699=LINE('',#27365,#4711);
#3700=LINE('',#27366,#4712);
#3701=LINE('',#27371,#4713);
#3702=LINE('',#27375,#4714);
#3703=LINE('',#27377,#4715);
#3704=LINE('',#27378,#4716);
#3705=LINE('',#27381,#4717);
#3706=LINE('',#27383,#4718);
#3707=LINE('',#27384,#4719);
#3708=LINE('',#27386,#4720);
#3709=LINE('',#27387,#4721);
#3710=LINE('',#27394,#4722);
#3711=LINE('',#27400,#4723);
#3712=LINE('',#27405,#4724);
#3713=LINE('',#27407,#4725);
#3714=LINE('',#27409,#4726);
#3715=LINE('',#27410,#4727);
#3716=LINE('',#27413,#4728);
#3717=LINE('',#27415,#4729);
#3718=LINE('',#27416,#4730);
#3719=LINE('',#27421,#4731);
#3720=LINE('',#27425,#4732);
#3721=LINE('',#27427,#4733);
#3722=LINE('',#27428,#4734);
#3723=LINE('',#27433,#4735);
#3724=LINE('',#27437,#4736);
#3725=LINE('',#27439,#4737);
#3726=LINE('',#27440,#4738);
#3727=LINE('',#27445,#4739);
#3728=LINE('',#27449,#4740);
#3729=LINE('',#27451,#4741);
#3730=LINE('',#27452,#4742);
#3731=LINE('',#27454,#4743);
#3732=LINE('',#27455,#4744);
#3733=LINE('',#27462,#4745);
#3734=LINE('',#27468,#4746);
#3735=LINE('',#27473,#4747);
#3736=LINE('',#27475,#4748);
#3737=LINE('',#27477,#4749);
#3738=LINE('',#27478,#4750);
#3739=LINE('',#27481,#4751);
#3740=LINE('',#27483,#4752);
#3741=LINE('',#27484,#4753);
#3742=LINE('',#27490,#4754);
#3743=LINE('',#27493,#4755);
#3744=LINE('',#27495,#4756);
#3745=LINE('',#27496,#4757);
#3746=LINE('',#27502,#4758);
#3747=LINE('',#27505,#4759);
#3748=LINE('',#27507,#4760);
#3749=LINE('',#27508,#4761);
#3750=LINE('',#27514,#4762);
#3751=LINE('',#27517,#4763);
#3752=LINE('',#27519,#4764);
#3753=LINE('',#27520,#4765);
#3754=LINE('',#27522,#4766);
#3755=LINE('',#27523,#4767);
#4146=VECTOR('',#15113,1000.);
#4147=VECTOR('',#15114,1000.);
#4148=VECTOR('',#15115,1000.);
#4149=VECTOR('',#15116,1000.);
#4150=VECTOR('',#15119,1000.);
#4151=VECTOR('',#15120,1000.);
#4152=VECTOR('',#15121,1000.);
#4153=VECTOR('',#15126,1000.);
#4154=VECTOR('',#15131,1000.);
#4155=VECTOR('',#15132,1000.);
#4156=VECTOR('',#15133,1000.);
#4157=VECTOR('',#15138,1000.);
#4158=VECTOR('',#15143,1000.);
#4159=VECTOR('',#15144,1000.);
#4160=VECTOR('',#15145,1000.);
#4161=VECTOR('',#15150,1000.);
#4162=VECTOR('',#15155,1000.);
#4163=VECTOR('',#15156,1000.);
#4164=VECTOR('',#15157,1000.);
#4165=VECTOR('',#15162,1000.);
#4166=VECTOR('',#15167,1000.);
#4167=VECTOR('',#15168,1000.);
#4168=VECTOR('',#15169,1000.);
#4169=VECTOR('',#15172,1000.);
#4170=VECTOR('',#15173,1000.);
#4171=VECTOR('',#15174,1000.);
#4172=VECTOR('',#15177,1000.);
#4173=VECTOR('',#15178,1000.);
#4174=VECTOR('',#15185,1000.);
#4175=VECTOR('',#15188,1000.);
#4176=VECTOR('',#15191,1000.);
#4177=VECTOR('',#15194,1000.);
#4178=VECTOR('',#15197,1000.);
#4179=VECTOR('',#15198,1000.);
#4180=VECTOR('',#15199,1000.);
#4181=VECTOR('',#15200,1000.);
#4182=VECTOR('',#15203,1000.);
#4183=VECTOR('',#15204,1000.);
#4184=VECTOR('',#15205,1000.);
#4185=VECTOR('',#15208,1000.);
#4186=VECTOR('',#15209,1000.);
#4187=VECTOR('',#15212,1000.);
#4188=VECTOR('',#15213,1000.);
#4189=VECTOR('',#15216,1000.);
#4190=VECTOR('',#15221,1000.);
#4191=VECTOR('',#15222,1000.);
#4192=VECTOR('',#15225,1000.);
#4193=VECTOR('',#15230,1000.);
#4194=VECTOR('',#15231,1000.);
#4195=VECTOR('',#15234,1000.);
#4196=VECTOR('',#15239,1000.);
#4197=VECTOR('',#15240,1000.);
#4198=VECTOR('',#15243,1000.);
#4199=VECTOR('',#15248,1000.);
#4200=VECTOR('',#15249,1000.);
#4201=VECTOR('',#15252,1000.);
#4202=VECTOR('',#15257,1000.);
#4203=VECTOR('',#15258,1000.);
#4204=VECTOR('',#15259,1000.);
#4205=VECTOR('',#15260,1000.);
#4206=VECTOR('',#15261,1000.);
#4207=VECTOR('',#15264,1000.);
#4208=VECTOR('',#15267,1000.);
#4209=VECTOR('',#15270,1000.);
#4210=VECTOR('',#15275,1000.);
#4211=VECTOR('',#15276,1000.);
#4212=VECTOR('',#15277,1000.);
#4213=VECTOR('',#15280,1000.);
#4214=VECTOR('',#15281,1000.);
#4215=VECTOR('',#15284,1000.);
#4216=VECTOR('',#15285,1000.);
#4217=VECTOR('',#15290,1000.);
#4218=VECTOR('',#15293,1000.);
#4219=VECTOR('',#15294,1000.);
#4220=VECTOR('',#15299,1000.);
#4221=VECTOR('',#15302,1000.);
#4222=VECTOR('',#15303,1000.);
#4223=VECTOR('',#15308,1000.);
#4224=VECTOR('',#15311,1000.);
#4225=VECTOR('',#15312,1000.);
#4226=VECTOR('',#15317,1000.);
#4227=VECTOR('',#15320,1000.);
#4228=VECTOR('',#15321,1000.);
#4229=VECTOR('',#15324,1000.);
#4230=VECTOR('',#15329,1000.);
#4231=VECTOR('',#15330,1000.);
#4232=VECTOR('',#15331,1000.);
#4233=VECTOR('',#15332,1000.);
#4234=VECTOR('',#15335,1000.);
#4235=VECTOR('',#15336,1000.);
#4236=VECTOR('',#15337,1000.);
#4237=VECTOR('',#15344,1000.);
#4238=VECTOR('',#15347,1000.);
#4239=VECTOR('',#15348,1000.);
#4240=VECTOR('',#15349,1000.);
#4241=VECTOR('',#15356,1000.);
#4242=VECTOR('',#15359,1000.);
#4243=VECTOR('',#15360,1000.);
#4244=VECTOR('',#15361,1000.);
#4245=VECTOR('',#15368,1000.);
#4246=VECTOR('',#15371,1000.);
#4247=VECTOR('',#15372,1000.);
#4248=VECTOR('',#15373,1000.);
#4249=VECTOR('',#15380,1000.);
#4250=VECTOR('',#15383,1000.);
#4251=VECTOR('',#15384,1000.);
#4252=VECTOR('',#15385,1000.);
#4253=VECTOR('',#15388,1000.);
#4254=VECTOR('',#15389,1000.);
#4255=VECTOR('',#15390,1000.);
#4256=VECTOR('',#15393,1000.);
#4257=VECTOR('',#15394,1000.);
#4258=VECTOR('',#15401,1000.);
#4259=VECTOR('',#15402,1000.);
#4260=VECTOR('',#15403,1000.);
#4261=VECTOR('',#15404,1000.);
#4262=VECTOR('',#15407,1000.);
#4263=VECTOR('',#15408,1000.);
#4264=VECTOR('',#15409,1000.);
#4265=VECTOR('',#15414,1000.);
#4266=VECTOR('',#15419,1000.);
#4267=VECTOR('',#15420,1000.);
#4268=VECTOR('',#15421,1000.);
#4269=VECTOR('',#15426,1000.);
#4270=VECTOR('',#15431,1000.);
#4271=VECTOR('',#15432,1000.);
#4272=VECTOR('',#15433,1000.);
#4273=VECTOR('',#15438,1000.);
#4274=VECTOR('',#15443,1000.);
#4275=VECTOR('',#15444,1000.);
#4276=VECTOR('',#15445,1000.);
#4277=VECTOR('',#15450,1000.);
#4278=VECTOR('',#15455,1000.);
#4279=VECTOR('',#15456,1000.);
#4280=VECTOR('',#15457,1000.);
#4281=VECTOR('',#15460,1000.);
#4282=VECTOR('',#15461,1000.);
#4283=VECTOR('',#15462,1000.);
#4284=VECTOR('',#15465,1000.);
#4285=VECTOR('',#15466,1000.);
#4286=VECTOR('',#15473,1000.);
#4287=VECTOR('',#15474,1000.);
#4288=VECTOR('',#15475,1000.);
#4289=VECTOR('',#15476,1000.);
#4290=VECTOR('',#15477,1000.);
#4291=VECTOR('',#15480,1000.);
#4292=VECTOR('',#15483,1000.);
#4293=VECTOR('',#15486,1000.);
#4294=VECTOR('',#15491,1000.);
#4295=VECTOR('',#15492,1000.);
#4296=VECTOR('',#15493,1000.);
#4297=VECTOR('',#15496,1000.);
#4298=VECTOR('',#15497,1000.);
#4299=VECTOR('',#15500,1000.);
#4300=VECTOR('',#15501,1000.);
#4301=VECTOR('',#15506,1000.);
#4302=VECTOR('',#15509,1000.);
#4303=VECTOR('',#15510,1000.);
#4304=VECTOR('',#15515,1000.);
#4305=VECTOR('',#15518,1000.);
#4306=VECTOR('',#15519,1000.);
#4307=VECTOR('',#15524,1000.);
#4308=VECTOR('',#15527,1000.);
#4309=VECTOR('',#15528,1000.);
#4310=VECTOR('',#15533,1000.);
#4311=VECTOR('',#15536,1000.);
#4312=VECTOR('',#15537,1000.);
#4313=VECTOR('',#15540,1000.);
#4314=VECTOR('',#15545,1000.);
#4315=VECTOR('',#15546,1000.);
#4316=VECTOR('',#15547,1000.);
#4317=VECTOR('',#15548,1000.);
#4318=VECTOR('',#15551,1000.);
#4319=VECTOR('',#15552,1000.);
#4320=VECTOR('',#15553,1000.);
#4321=VECTOR('',#15558,1000.);
#4322=VECTOR('',#15563,1000.);
#4323=VECTOR('',#15564,1000.);
#4324=VECTOR('',#15565,1000.);
#4325=VECTOR('',#15570,1000.);
#4326=VECTOR('',#15575,1000.);
#4327=VECTOR('',#15576,1000.);
#4328=VECTOR('',#15577,1000.);
#4329=VECTOR('',#15582,1000.);
#4330=VECTOR('',#15587,1000.);
#4331=VECTOR('',#15588,1000.);
#4332=VECTOR('',#15589,1000.);
#4333=VECTOR('',#15594,1000.);
#4334=VECTOR('',#15599,1000.);
#4335=VECTOR('',#15600,1000.);
#4336=VECTOR('',#15601,1000.);
#4337=VECTOR('',#15604,1000.);
#4338=VECTOR('',#15605,1000.);
#4339=VECTOR('',#15606,1000.);
#4340=VECTOR('',#15609,1000.);
#4341=VECTOR('',#15610,1000.);
#4342=VECTOR('',#15617,1000.);
#4343=VECTOR('',#15618,1000.);
#4344=VECTOR('',#15619,1000.);
#4345=VECTOR('',#15620,1000.);
#4346=VECTOR('',#15621,1000.);
#4347=VECTOR('',#15624,1000.);
#4348=VECTOR('',#15627,1000.);
#4349=VECTOR('',#15630,1000.);
#4350=VECTOR('',#15635,1000.);
#4351=VECTOR('',#15636,1000.);
#4352=VECTOR('',#15637,1000.);
#4353=VECTOR('',#15640,1000.);
#4354=VECTOR('',#15641,1000.);
#4355=VECTOR('',#15644,1000.);
#4356=VECTOR('',#15645,1000.);
#4357=VECTOR('',#15650,1000.);
#4358=VECTOR('',#15653,1000.);
#4359=VECTOR('',#15654,1000.);
#4360=VECTOR('',#15659,1000.);
#4361=VECTOR('',#15662,1000.);
#4362=VECTOR('',#15663,1000.);
#4363=VECTOR('',#15668,1000.);
#4364=VECTOR('',#15671,1000.);
#4365=VECTOR('',#15672,1000.);
#4366=VECTOR('',#15677,1000.);
#4367=VECTOR('',#15680,1000.);
#4368=VECTOR('',#15681,1000.);
#4369=VECTOR('',#15684,1000.);
#4370=VECTOR('',#15689,1000.);
#4371=VECTOR('',#15690,1000.);
#4372=VECTOR('',#15693,1000.);
#4373=VECTOR('',#15696,1000.);
#4374=VECTOR('',#15699,1000.);
#4375=VECTOR('',#15702,1000.);
#4376=VECTOR('',#15703,1000.);
#4377=VECTOR('',#15704,1000.);
#4378=VECTOR('',#15707,1000.);
#4379=VECTOR('',#15708,1000.);
#4380=VECTOR('',#15709,1000.);
#4381=VECTOR('',#15712,1000.);
#4382=VECTOR('',#15713,1000.);
#4383=VECTOR('',#15716,1000.);
#4384=VECTOR('',#15717,1000.);
#4385=VECTOR('',#15720,1000.);
#4386=VECTOR('',#15725,1000.);
#4387=VECTOR('',#15726,1000.);
#4388=VECTOR('',#15729,1000.);
#4389=VECTOR('',#15734,1000.);
#4390=VECTOR('',#15735,1000.);
#4391=VECTOR('',#15738,1000.);
#4392=VECTOR('',#15743,1000.);
#4393=VECTOR('',#15744,1000.);
#4394=VECTOR('',#15747,1000.);
#4395=VECTOR('',#15752,1000.);
#4396=VECTOR('',#15753,1000.);
#4397=VECTOR('',#15756,1000.);
#4398=VECTOR('',#15761,1000.);
#4399=VECTOR('',#15762,1000.);
#4400=VECTOR('',#15763,1000.);
#4401=VECTOR('',#15764,1000.);
#4402=VECTOR('',#15767,1000.);
#4403=VECTOR('',#15770,1000.);
#4404=VECTOR('',#15773,1000.);
#4405=VECTOR('',#15776,1000.);
#4406=VECTOR('',#15779,1000.);
#4407=VECTOR('',#15780,1000.);
#4408=VECTOR('',#15781,1000.);
#4409=VECTOR('',#15784,1000.);
#4410=VECTOR('',#15785,1000.);
#4411=VECTOR('',#15788,1000.);
#4412=VECTOR('',#15789,1000.);
#4413=VECTOR('',#15794,1000.);
#4414=VECTOR('',#15797,1000.);
#4415=VECTOR('',#15798,1000.);
#4416=VECTOR('',#15803,1000.);
#4417=VECTOR('',#15806,1000.);
#4418=VECTOR('',#15807,1000.);
#4419=VECTOR('',#15812,1000.);
#4420=VECTOR('',#15815,1000.);
#4421=VECTOR('',#15816,1000.);
#4422=VECTOR('',#15821,1000.);
#4423=VECTOR('',#15824,1000.);
#4424=VECTOR('',#15825,1000.);
#4425=VECTOR('',#15828,1000.);
#4426=VECTOR('',#15833,1000.);
#4427=VECTOR('',#15834,1000.);
#4428=VECTOR('',#15835,1000.);
#4429=VECTOR('',#15836,1000.);
#4430=VECTOR('',#15839,1000.);
#4431=VECTOR('',#15840,1000.);
#4432=VECTOR('',#15841,1000.);
#4433=VECTOR('',#15846,1000.);
#4434=VECTOR('',#15851,1000.);
#4435=VECTOR('',#15852,1000.);
#4436=VECTOR('',#15853,1000.);
#4437=VECTOR('',#15858,1000.);
#4438=VECTOR('',#15863,1000.);
#4439=VECTOR('',#15864,1000.);
#4440=VECTOR('',#15865,1000.);
#4441=VECTOR('',#15870,1000.);
#4442=VECTOR('',#15875,1000.);
#4443=VECTOR('',#15876,1000.);
#4444=VECTOR('',#15877,1000.);
#4445=VECTOR('',#15880,1000.);
#4446=VECTOR('',#15881,1000.);
#4447=VECTOR('',#15888,1000.);
#4448=VECTOR('',#15889,1000.);
#4449=VECTOR('',#15890,1000.);
#4450=VECTOR('',#15891,1000.);
#4451=VECTOR('',#15894,1000.);
#4452=VECTOR('',#15895,1000.);
#4453=VECTOR('',#15896,1000.);
#4454=VECTOR('',#15901,1000.);
#4455=VECTOR('',#15906,1000.);
#4456=VECTOR('',#15907,1000.);
#4457=VECTOR('',#15908,1000.);
#4458=VECTOR('',#15913,1000.);
#4459=VECTOR('',#15918,1000.);
#4460=VECTOR('',#15919,1000.);
#4461=VECTOR('',#15920,1000.);
#4462=VECTOR('',#15925,1000.);
#4463=VECTOR('',#15930,1000.);
#4464=VECTOR('',#15931,1000.);
#4465=VECTOR('',#15932,1000.);
#4466=VECTOR('',#15935,1000.);
#4467=VECTOR('',#15936,1000.);
#4468=VECTOR('',#15943,1000.);
#4469=VECTOR('',#15944,1000.);
#4470=VECTOR('',#15945,1000.);
#4471=VECTOR('',#15946,1000.);
#4472=VECTOR('',#15949,1000.);
#4473=VECTOR('',#15950,1000.);
#4474=VECTOR('',#15951,1000.);
#4475=VECTOR('',#15958,1000.);
#4476=VECTOR('',#15961,1000.);
#4477=VECTOR('',#15962,1000.);
#4478=VECTOR('',#15963,1000.);
#4479=VECTOR('',#15970,1000.);
#4480=VECTOR('',#15973,1000.);
#4481=VECTOR('',#15974,1000.);
#4482=VECTOR('',#15975,1000.);
#4483=VECTOR('',#15982,1000.);
#4484=VECTOR('',#15985,1000.);
#4485=VECTOR('',#15986,1000.);
#4486=VECTOR('',#15987,1000.);
#4487=VECTOR('',#15990,1000.);
#4488=VECTOR('',#15991,1000.);
#4489=VECTOR('',#15998,1000.);
#4490=VECTOR('',#15999,1000.);
#4491=VECTOR('',#16000,1000.);
#4492=VECTOR('',#16001,1000.);
#4493=VECTOR('',#16004,1000.);
#4494=VECTOR('',#16005,1000.);
#4495=VECTOR('',#16006,1000.);
#4496=VECTOR('',#16013,1000.);
#4497=VECTOR('',#16016,1000.);
#4498=VECTOR('',#16017,1000.);
#4499=VECTOR('',#16018,1000.);
#4500=VECTOR('',#16025,1000.);
#4501=VECTOR('',#16028,1000.);
#4502=VECTOR('',#16029,1000.);
#4503=VECTOR('',#16030,1000.);
#4504=VECTOR('',#16037,1000.);
#4505=VECTOR('',#16040,1000.);
#4506=VECTOR('',#16041,1000.);
#4507=VECTOR('',#16042,1000.);
#4508=VECTOR('',#16045,1000.);
#4509=VECTOR('',#16046,1000.);
#4510=VECTOR('',#16053,1000.);
#4511=VECTOR('',#16054,1000.);
#4512=VECTOR('',#16057,1000.);
#4513=VECTOR('',#16060,1000.);
#4514=VECTOR('',#16063,1000.);
#4515=VECTOR('',#16064,1000.);
#4516=VECTOR('',#16067,1000.);
#4517=VECTOR('',#16068,1000.);
#4518=VECTOR('',#16069,1000.);
#4519=VECTOR('',#16072,1000.);
#4520=VECTOR('',#16073,1000.);
#4521=VECTOR('',#16076,1000.);
#4522=VECTOR('',#16081,1000.);
#4523=VECTOR('',#16082,1000.);
#4524=VECTOR('',#16085,1000.);
#4525=VECTOR('',#16090,1000.);
#4526=VECTOR('',#16091,1000.);
#4527=VECTOR('',#16094,1000.);
#4528=VECTOR('',#16099,1000.);
#4529=VECTOR('',#16100,1000.);
#4530=VECTOR('',#16103,1000.);
#4531=VECTOR('',#16108,1000.);
#4532=VECTOR('',#16109,1000.);
#4533=VECTOR('',#16110,1000.);
#4534=VECTOR('',#16111,1000.);
#4535=VECTOR('',#16114,1000.);
#4536=VECTOR('',#16115,1000.);
#4537=VECTOR('',#16116,1000.);
#4538=VECTOR('',#16121,1000.);
#4539=VECTOR('',#16126,1000.);
#4540=VECTOR('',#16127,1000.);
#4541=VECTOR('',#16128,1000.);
#4542=VECTOR('',#16133,1000.);
#4543=VECTOR('',#16138,1000.);
#4544=VECTOR('',#16139,1000.);
#4545=VECTOR('',#16140,1000.);
#4546=VECTOR('',#16145,1000.);
#4547=VECTOR('',#16150,1000.);
#4548=VECTOR('',#16151,1000.);
#4549=VECTOR('',#16152,1000.);
#4550=VECTOR('',#16155,1000.);
#4551=VECTOR('',#16156,1000.);
#4552=VECTOR('',#16163,1000.);
#4553=VECTOR('',#16164,1000.);
#4554=VECTOR('',#16165,1000.);
#4555=VECTOR('',#16168,1000.);
#4556=VECTOR('',#16171,1000.);
#4557=VECTOR('',#16174,1000.);
#4558=VECTOR('',#16177,1000.);
#4559=VECTOR('',#16178,1000.);
#4560=VECTOR('',#16179,1000.);
#4561=VECTOR('',#16182,1000.);
#4562=VECTOR('',#16183,1000.);
#4563=VECTOR('',#16188,1000.);
#4564=VECTOR('',#16191,1000.);
#4565=VECTOR('',#16192,1000.);
#4566=VECTOR('',#16197,1000.);
#4567=VECTOR('',#16200,1000.);
#4568=VECTOR('',#16201,1000.);
#4569=VECTOR('',#16206,1000.);
#4570=VECTOR('',#16209,1000.);
#4571=VECTOR('',#16210,1000.);
#4572=VECTOR('',#16213,1000.);
#4573=VECTOR('',#16218,1000.);
#4574=VECTOR('',#16219,1000.);
#4575=VECTOR('',#16220,1000.);
#4576=VECTOR('',#16223,1000.);
#4577=VECTOR('',#16226,1000.);
#4578=VECTOR('',#16229,1000.);
#4579=VECTOR('',#16232,1000.);
#4580=VECTOR('',#16233,1000.);
#4581=VECTOR('',#16234,1000.);
#4582=VECTOR('',#16237,1000.);
#4583=VECTOR('',#16238,1000.);
#4584=VECTOR('',#16243,1000.);
#4585=VECTOR('',#16246,1000.);
#4586=VECTOR('',#16247,1000.);
#4587=VECTOR('',#16252,1000.);
#4588=VECTOR('',#16255,1000.);
#4589=VECTOR('',#16256,1000.);
#4590=VECTOR('',#16261,1000.);
#4591=VECTOR('',#16264,1000.);
#4592=VECTOR('',#16265,1000.);
#4593=VECTOR('',#16268,1000.);
#4594=VECTOR('',#16273,1000.);
#4595=VECTOR('',#16274,1000.);
#4596=VECTOR('',#16275,1000.);
#4597=VECTOR('',#16276,1000.);
#4598=VECTOR('',#16279,1000.);
#4599=VECTOR('',#16280,1000.);
#4600=VECTOR('',#16281,1000.);
#4601=VECTOR('',#16288,1000.);
#4602=VECTOR('',#16291,1000.);
#4603=VECTOR('',#16292,1000.);
#4604=VECTOR('',#16293,1000.);
#4605=VECTOR('',#16300,1000.);
#4606=VECTOR('',#16303,1000.);
#4607=VECTOR('',#16304,1000.);
#4608=VECTOR('',#16305,1000.);
#4609=VECTOR('',#16312,1000.);
#4610=VECTOR('',#16315,1000.);
#4611=VECTOR('',#16316,1000.);
#4612=VECTOR('',#16317,1000.);
#4613=VECTOR('',#16320,1000.);
#4614=VECTOR('',#16321,1000.);
#4615=VECTOR('',#16328,1000.);
#4616=VECTOR('',#16329,1000.);
#4617=VECTOR('',#16332,1000.);
#4618=VECTOR('',#16335,1000.);
#4619=VECTOR('',#16338,1000.);
#4620=VECTOR('',#16339,1000.);
#4621=VECTOR('',#16342,1000.);
#4622=VECTOR('',#16343,1000.);
#4623=VECTOR('',#16344,1000.);
#4624=VECTOR('',#16347,1000.);
#4625=VECTOR('',#16348,1000.);
#4626=VECTOR('',#16351,1000.);
#4627=VECTOR('',#16356,1000.);
#4628=VECTOR('',#16357,1000.);
#4629=VECTOR('',#16360,1000.);
#4630=VECTOR('',#16365,1000.);
#4631=VECTOR('',#16366,1000.);
#4632=VECTOR('',#16369,1000.);
#4633=VECTOR('',#16374,1000.);
#4634=VECTOR('',#16375,1000.);
#4635=VECTOR('',#16378,1000.);
#4636=VECTOR('',#16385,1000.);
#4637=VECTOR('',#16388,1000.);
#4638=VECTOR('',#16393,1000.);
#4639=VECTOR('',#16396,1000.);
#4640=VECTOR('',#16401,1000.);
#4641=VECTOR('',#16404,1000.);
#4642=VECTOR('',#16409,1000.);
#4643=VECTOR('',#16412,1000.);
#4644=VECTOR('',#16415,1000.);
#4645=VECTOR('',#16416,1000.);
#4646=VECTOR('',#16417,1000.);
#4647=VECTOR('',#16418,1000.);
#4648=VECTOR('',#16421,1000.);
#4649=VECTOR('',#16422,1000.);
#4650=VECTOR('',#16423,1000.);
#4651=VECTOR('',#16424,1000.);
#4652=VECTOR('',#16427,1000.);
#4653=VECTOR('',#16428,1000.);
#4654=VECTOR('',#16429,1000.);
#4655=VECTOR('',#16430,1000.);
#4656=VECTOR('',#16433,1000.);
#4657=VECTOR('',#16434,1000.);
#4658=VECTOR('',#16435,1000.);
#4659=VECTOR('',#16436,1000.);
#4660=VECTOR('',#16439,1000.);
#4661=VECTOR('',#16440,1000.);
#4662=VECTOR('',#16441,1000.);
#4663=VECTOR('',#16442,1000.);
#4664=VECTOR('',#16443,1000.);
#4665=VECTOR('',#16444,1000.);
#4666=VECTOR('',#16447,1000.);
#4667=VECTOR('',#16448,1000.);
#4668=VECTOR('',#16451,1000.);
#4669=VECTOR('',#16452,1000.);
#4670=VECTOR('',#16455,1000.);
#4671=VECTOR('',#16456,1000.);
#4672=VECTOR('',#16461,1000.);
#4673=VECTOR('',#16462,1000.);
#4674=VECTOR('',#16463,1000.);
#4675=VECTOR('',#16464,1000.);
#4676=VECTOR('',#16465,1000.);
#4677=VECTOR('',#16468,1000.);
#4678=VECTOR('',#16469,1000.);
#4679=VECTOR('',#16472,1000.);
#4680=VECTOR('',#16473,1000.);
#4681=VECTOR('',#16476,1000.);
#4682=VECTOR('',#16477,1000.);
#4683=VECTOR('',#16480,1000.);
#4684=VECTOR('',#16483,1000.);
#4685=VECTOR('',#16486,1000.);
#4686=VECTOR('',#16491,1000.);
#4687=VECTOR('',#16494,1000.);
#4688=VECTOR('',#16499,1000.);
#4689=VECTOR('',#16502,1000.);
#4690=VECTOR('',#16507,1000.);
#4691=VECTOR('',#16510,1000.);
#4692=VECTOR('',#16525,8.74999999999998);
#4693=VECTOR('',#16532,8.74999999999998);
#4694=VECTOR('',#16537,1000.);
#4695=VECTOR('',#16538,1000.);
#4696=VECTOR('',#16539,1000.);
#4697=VECTOR('',#16540,1000.);
#4698=VECTOR('',#16543,1000.);
#4699=VECTOR('',#16544,1000.);
#4700=VECTOR('',#16545,1000.);
#4701=VECTOR('',#16550,1000.);
#4702=VECTOR('',#16555,1000.);
#4703=VECTOR('',#16556,1000.);
#4704=VECTOR('',#16557,1000.);
#4705=VECTOR('',#16562,1000.);
#4706=VECTOR('',#16567,1000.);
#4707=VECTOR('',#16568,1000.);
#4708=VECTOR('',#16569,1000.);
#4709=VECTOR('',#16574,1000.);
#4710=VECTOR('',#16579,1000.);
#4711=VECTOR('',#16580,1000.);
#4712=VECTOR('',#16581,1000.);
#4713=VECTOR('',#16586,1000.);
#4714=VECTOR('',#16591,1000.);
#4715=VECTOR('',#16592,1000.);
#4716=VECTOR('',#16593,1000.);
#4717=VECTOR('',#16596,1000.);
#4718=VECTOR('',#16597,1000.);
#4719=VECTOR('',#16598,1000.);
#4720=VECTOR('',#16601,1000.);
#4721=VECTOR('',#16602,1000.);
#4722=VECTOR('',#16611,4.5);
#4723=VECTOR('',#16618,4.5);
#4724=VECTOR('',#16623,1000.);
#4725=VECTOR('',#16624,1000.);
#4726=VECTOR('',#16625,1000.);
#4727=VECTOR('',#16626,1000.);
#4728=VECTOR('',#16629,1000.);
#4729=VECTOR('',#16630,1000.);
#4730=VECTOR('',#16631,1000.);
#4731=VECTOR('',#16636,1000.);
#4732=VECTOR('',#16641,1000.);
#4733=VECTOR('',#16642,1000.);
#4734=VECTOR('',#16643,1000.);
#4735=VECTOR('',#16648,1000.);
#4736=VECTOR('',#16653,1000.);
#4737=VECTOR('',#16654,1000.);
#4738=VECTOR('',#16655,1000.);
#4739=VECTOR('',#16660,1000.);
#4740=VECTOR('',#16665,1000.);
#4741=VECTOR('',#16666,1000.);
#4742=VECTOR('',#16667,1000.);
#4743=VECTOR('',#16670,1000.);
#4744=VECTOR('',#16671,1000.);
#4745=VECTOR('',#16680,4.5);
#4746=VECTOR('',#16687,4.5);
#4747=VECTOR('',#16692,1000.);
#4748=VECTOR('',#16693,1000.);
#4749=VECTOR('',#16694,1000.);
#4750=VECTOR('',#16695,1000.);
#4751=VECTOR('',#16698,1000.);
#4752=VECTOR('',#16699,1000.);
#4753=VECTOR('',#16700,1000.);
#4754=VECTOR('',#16707,1000.);
#4755=VECTOR('',#16710,1000.);
#4756=VECTOR('',#16711,1000.);
#4757=VECTOR('',#16712,1000.);
#4758=VECTOR('',#16719,1000.);
#4759=VECTOR('',#16722,1000.);
#4760=VECTOR('',#16723,1000.);
#4761=VECTOR('',#16724,1000.);
#4762=VECTOR('',#16731,1000.);
#4763=VECTOR('',#16734,1000.);
#4764=VECTOR('',#16735,1000.);
#4765=VECTOR('',#16736,1000.);
#4766=VECTOR('',#16739,1000.);
#4767=VECTOR('',#16740,1000.);
#5292=VERTEX_POINT('',#25859);
#5293=VERTEX_POINT('',#25860);
#5294=VERTEX_POINT('',#25862);
#5295=VERTEX_POINT('',#25864);
#5296=VERTEX_POINT('',#25868);
#5297=VERTEX_POINT('',#25870);
#5298=VERTEX_POINT('',#25874);
#5299=VERTEX_POINT('',#25876);
#5300=VERTEX_POINT('',#25880);
#5301=VERTEX_POINT('',#25882);
#5302=VERTEX_POINT('',#25886);
#5303=VERTEX_POINT('',#25888);
#5304=VERTEX_POINT('',#25892);
#5305=VERTEX_POINT('',#25894);
#5306=VERTEX_POINT('',#25898);
#5307=VERTEX_POINT('',#25900);
#5308=VERTEX_POINT('',#25904);
#5309=VERTEX_POINT('',#25906);
#5310=VERTEX_POINT('',#25910);
#5311=VERTEX_POINT('',#25912);
#5312=VERTEX_POINT('',#25916);
#5313=VERTEX_POINT('',#25918);
#5314=VERTEX_POINT('',#25922);
#5315=VERTEX_POINT('',#25924);
#5316=VERTEX_POINT('',#25933);
#5317=VERTEX_POINT('',#25934);
#5318=VERTEX_POINT('',#25936);
#5319=VERTEX_POINT('',#25938);
#5320=VERTEX_POINT('',#25940);
#5321=VERTEX_POINT('',#25942);
#5322=VERTEX_POINT('',#25944);
#5323=VERTEX_POINT('',#25946);
#5324=VERTEX_POINT('',#25948);
#5325=VERTEX_POINT('',#25950);
#5326=VERTEX_POINT('',#25952);
#5327=VERTEX_POINT('',#25954);
#5328=VERTEX_POINT('',#25958);
#5329=VERTEX_POINT('',#25960);
#5330=VERTEX_POINT('',#25964);
#5331=VERTEX_POINT('',#25968);
#5332=VERTEX_POINT('',#25972);
#5333=VERTEX_POINT('',#25976);
#5334=VERTEX_POINT('',#25980);
#5335=VERTEX_POINT('',#25984);
#5336=VERTEX_POINT('',#25988);
#5337=VERTEX_POINT('',#25992);
#5338=VERTEX_POINT('',#25996);
#5339=VERTEX_POINT('',#26000);
#5340=VERTEX_POINT('',#26007);
#5341=VERTEX_POINT('',#26008);
#5342=VERTEX_POINT('',#26010);
#5343=VERTEX_POINT('',#26012);
#5344=VERTEX_POINT('',#26014);
#5345=VERTEX_POINT('',#26016);
#5346=VERTEX_POINT('',#26018);
#5347=VERTEX_POINT('',#26020);
#5348=VERTEX_POINT('',#26022);
#5349=VERTEX_POINT('',#26024);
#5350=VERTEX_POINT('',#26026);
#5351=VERTEX_POINT('',#26028);
#5352=VERTEX_POINT('',#26032);
#5353=VERTEX_POINT('',#26034);
#5354=VERTEX_POINT('',#26038);
#5355=VERTEX_POINT('',#26042);
#5356=VERTEX_POINT('',#26046);
#5357=VERTEX_POINT('',#26050);
#5358=VERTEX_POINT('',#26054);
#5359=VERTEX_POINT('',#26058);
#5360=VERTEX_POINT('',#26062);
#5361=VERTEX_POINT('',#26066);
#5362=VERTEX_POINT('',#26070);
#5363=VERTEX_POINT('',#26074);
#5364=VERTEX_POINT('',#26081);
#5365=VERTEX_POINT('',#26082);
#5366=VERTEX_POINT('',#26084);
#5367=VERTEX_POINT('',#26086);
#5368=VERTEX_POINT('',#26090);
#5369=VERTEX_POINT('',#26092);
#5370=VERTEX_POINT('',#26096);
#5371=VERTEX_POINT('',#26098);
#5372=VERTEX_POINT('',#26102);
#5373=VERTEX_POINT('',#26104);
#5374=VERTEX_POINT('',#26108);
#5375=VERTEX_POINT('',#26110);
#5376=VERTEX_POINT('',#26114);
#5377=VERTEX_POINT('',#26116);
#5378=VERTEX_POINT('',#26120);
#5379=VERTEX_POINT('',#26122);
#5380=VERTEX_POINT('',#26126);
#5381=VERTEX_POINT('',#26128);
#5382=VERTEX_POINT('',#26132);
#5383=VERTEX_POINT('',#26134);
#5384=VERTEX_POINT('',#26138);
#5385=VERTEX_POINT('',#26140);
#5386=VERTEX_POINT('',#26144);
#5387=VERTEX_POINT('',#26146);
#5388=VERTEX_POINT('',#26155);
#5389=VERTEX_POINT('',#26156);
#5390=VERTEX_POINT('',#26158);
#5391=VERTEX_POINT('',#26160);
#5392=VERTEX_POINT('',#26164);
#5393=VERTEX_POINT('',#26166);
#5394=VERTEX_POINT('',#26170);
#5395=VERTEX_POINT('',#26172);
#5396=VERTEX_POINT('',#26176);
#5397=VERTEX_POINT('',#26178);
#5398=VERTEX_POINT('',#26182);
#5399=VERTEX_POINT('',#26184);
#5400=VERTEX_POINT('',#26188);
#5401=VERTEX_POINT('',#26190);
#5402=VERTEX_POINT('',#26194);
#5403=VERTEX_POINT('',#26196);
#5404=VERTEX_POINT('',#26200);
#5405=VERTEX_POINT('',#26202);
#5406=VERTEX_POINT('',#26206);
#5407=VERTEX_POINT('',#26208);
#5408=VERTEX_POINT('',#26212);
#5409=VERTEX_POINT('',#26214);
#5410=VERTEX_POINT('',#26218);
#5411=VERTEX_POINT('',#26220);
#5412=VERTEX_POINT('',#26229);
#5413=VERTEX_POINT('',#26230);
#5414=VERTEX_POINT('',#26232);
#5415=VERTEX_POINT('',#26234);
#5416=VERTEX_POINT('',#26236);
#5417=VERTEX_POINT('',#26238);
#5418=VERTEX_POINT('',#26240);
#5419=VERTEX_POINT('',#26242);
#5420=VERTEX_POINT('',#26244);
#5421=VERTEX_POINT('',#26246);
#5422=VERTEX_POINT('',#26248);
#5423=VERTEX_POINT('',#26250);
#5424=VERTEX_POINT('',#26254);
#5425=VERTEX_POINT('',#26256);
#5426=VERTEX_POINT('',#26260);
#5427=VERTEX_POINT('',#26264);
#5428=VERTEX_POINT('',#26268);
#5429=VERTEX_POINT('',#26272);
#5430=VERTEX_POINT('',#26276);
#5431=VERTEX_POINT('',#26280);
#5432=VERTEX_POINT('',#26284);
#5433=VERTEX_POINT('',#26288);
#5434=VERTEX_POINT('',#26292);
#5435=VERTEX_POINT('',#26296);
#5436=VERTEX_POINT('',#26303);
#5437=VERTEX_POINT('',#26304);
#5438=VERTEX_POINT('',#26306);
#5439=VERTEX_POINT('',#26308);
#5440=VERTEX_POINT('',#26312);
#5441=VERTEX_POINT('',#26314);
#5442=VERTEX_POINT('',#26318);
#5443=VERTEX_POINT('',#26320);
#5444=VERTEX_POINT('',#26324);
#5445=VERTEX_POINT('',#26326);
#5446=VERTEX_POINT('',#26330);
#5447=VERTEX_POINT('',#26332);
#5448=VERTEX_POINT('',#26336);
#5449=VERTEX_POINT('',#26338);
#5450=VERTEX_POINT('',#26342);
#5451=VERTEX_POINT('',#26344);
#5452=VERTEX_POINT('',#26348);
#5453=VERTEX_POINT('',#26350);
#5454=VERTEX_POINT('',#26354);
#5455=VERTEX_POINT('',#26356);
#5456=VERTEX_POINT('',#26360);
#5457=VERTEX_POINT('',#26362);
#5458=VERTEX_POINT('',#26366);
#5459=VERTEX_POINT('',#26368);
#5460=VERTEX_POINT('',#26377);
#5461=VERTEX_POINT('',#26378);
#5462=VERTEX_POINT('',#26380);
#5463=VERTEX_POINT('',#26382);
#5464=VERTEX_POINT('',#26384);
#5465=VERTEX_POINT('',#26386);
#5466=VERTEX_POINT('',#26388);
#5467=VERTEX_POINT('',#26390);
#5468=VERTEX_POINT('',#26392);
#5469=VERTEX_POINT('',#26394);
#5470=VERTEX_POINT('',#26396);
#5471=VERTEX_POINT('',#26398);
#5472=VERTEX_POINT('',#26402);
#5473=VERTEX_POINT('',#26404);
#5474=VERTEX_POINT('',#26408);
#5475=VERTEX_POINT('',#26412);
#5476=VERTEX_POINT('',#26416);
#5477=VERTEX_POINT('',#26420);
#5478=VERTEX_POINT('',#26424);
#5479=VERTEX_POINT('',#26428);
#5480=VERTEX_POINT('',#26432);
#5481=VERTEX_POINT('',#26436);
#5482=VERTEX_POINT('',#26440);
#5483=VERTEX_POINT('',#26444);
#5484=VERTEX_POINT('',#26451);
#5485=VERTEX_POINT('',#26452);
#5486=VERTEX_POINT('',#26454);
#5487=VERTEX_POINT('',#26456);
#5488=VERTEX_POINT('',#26458);
#5489=VERTEX_POINT('',#26460);
#5490=VERTEX_POINT('',#26462);
#5491=VERTEX_POINT('',#26464);
#5492=VERTEX_POINT('',#26466);
#5493=VERTEX_POINT('',#26468);
#5494=VERTEX_POINT('',#26470);
#5495=VERTEX_POINT('',#26472);
#5496=VERTEX_POINT('',#26476);
#5497=VERTEX_POINT('',#26478);
#5498=VERTEX_POINT('',#26482);
#5499=VERTEX_POINT('',#26486);
#5500=VERTEX_POINT('',#26490);
#5501=VERTEX_POINT('',#26494);
#5502=VERTEX_POINT('',#26498);
#5503=VERTEX_POINT('',#26502);
#5504=VERTEX_POINT('',#26506);
#5505=VERTEX_POINT('',#26510);
#5506=VERTEX_POINT('',#26514);
#5507=VERTEX_POINT('',#26518);
#5508=VERTEX_POINT('',#26525);
#5509=VERTEX_POINT('',#26526);
#5510=VERTEX_POINT('',#26528);
#5511=VERTEX_POINT('',#26530);
#5512=VERTEX_POINT('',#26532);
#5513=VERTEX_POINT('',#26534);
#5514=VERTEX_POINT('',#26536);
#5515=VERTEX_POINT('',#26538);
#5516=VERTEX_POINT('',#26540);
#5517=VERTEX_POINT('',#26542);
#5518=VERTEX_POINT('',#26544);
#5519=VERTEX_POINT('',#26546);
#5520=VERTEX_POINT('',#26550);
#5521=VERTEX_POINT('',#26552);
#5522=VERTEX_POINT('',#26556);
#5523=VERTEX_POINT('',#26560);
#5524=VERTEX_POINT('',#26564);
#5525=VERTEX_POINT('',#26568);
#5526=VERTEX_POINT('',#26572);
#5527=VERTEX_POINT('',#26576);
#5528=VERTEX_POINT('',#26580);
#5529=VERTEX_POINT('',#26584);
#5530=VERTEX_POINT('',#26588);
#5531=VERTEX_POINT('',#26592);
#5532=VERTEX_POINT('',#26599);
#5533=VERTEX_POINT('',#26600);
#5534=VERTEX_POINT('',#26602);
#5535=VERTEX_POINT('',#26604);
#5536=VERTEX_POINT('',#26608);
#5537=VERTEX_POINT('',#26610);
#5538=VERTEX_POINT('',#26614);
#5539=VERTEX_POINT('',#26616);
#5540=VERTEX_POINT('',#26620);
#5541=VERTEX_POINT('',#26622);
#5542=VERTEX_POINT('',#26626);
#5543=VERTEX_POINT('',#26628);
#5544=VERTEX_POINT('',#26632);
#5545=VERTEX_POINT('',#26634);
#5546=VERTEX_POINT('',#26638);
#5547=VERTEX_POINT('',#26640);
#5548=VERTEX_POINT('',#26644);
#5549=VERTEX_POINT('',#26646);
#5550=VERTEX_POINT('',#26655);
#5551=VERTEX_POINT('',#26656);
#5552=VERTEX_POINT('',#26658);
#5553=VERTEX_POINT('',#26660);
#5554=VERTEX_POINT('',#26664);
#5555=VERTEX_POINT('',#26666);
#5556=VERTEX_POINT('',#26670);
#5557=VERTEX_POINT('',#26672);
#5558=VERTEX_POINT('',#26676);
#5559=VERTEX_POINT('',#26678);
#5560=VERTEX_POINT('',#26682);
#5561=VERTEX_POINT('',#26684);
#5562=VERTEX_POINT('',#26688);
#5563=VERTEX_POINT('',#26690);
#5564=VERTEX_POINT('',#26694);
#5565=VERTEX_POINT('',#26696);
#5566=VERTEX_POINT('',#26700);
#5567=VERTEX_POINT('',#26702);
#5568=VERTEX_POINT('',#26711);
#5569=VERTEX_POINT('',#26712);
#5570=VERTEX_POINT('',#26714);
#5571=VERTEX_POINT('',#26716);
#5572=VERTEX_POINT('',#26720);
#5573=VERTEX_POINT('',#26722);
#5574=VERTEX_POINT('',#26726);
#5575=VERTEX_POINT('',#26728);
#5576=VERTEX_POINT('',#26732);
#5577=VERTEX_POINT('',#26734);
#5578=VERTEX_POINT('',#26738);
#5579=VERTEX_POINT('',#26740);
#5580=VERTEX_POINT('',#26744);
#5581=VERTEX_POINT('',#26746);
#5582=VERTEX_POINT('',#26750);
#5583=VERTEX_POINT('',#26752);
#5584=VERTEX_POINT('',#26756);
#5585=VERTEX_POINT('',#26758);
#5586=VERTEX_POINT('',#26767);
#5587=VERTEX_POINT('',#26768);
#5588=VERTEX_POINT('',#26770);
#5589=VERTEX_POINT('',#26772);
#5590=VERTEX_POINT('',#26776);
#5591=VERTEX_POINT('',#26778);
#5592=VERTEX_POINT('',#26782);
#5593=VERTEX_POINT('',#26784);
#5594=VERTEX_POINT('',#26788);
#5595=VERTEX_POINT('',#26790);
#5596=VERTEX_POINT('',#26794);
#5597=VERTEX_POINT('',#26796);
#5598=VERTEX_POINT('',#26800);
#5599=VERTEX_POINT('',#26802);
#5600=VERTEX_POINT('',#26806);
#5601=VERTEX_POINT('',#26808);
#5602=VERTEX_POINT('',#26812);
#5603=VERTEX_POINT('',#26814);
#5604=VERTEX_POINT('',#26823);
#5605=VERTEX_POINT('',#26824);
#5606=VERTEX_POINT('',#26826);
#5607=VERTEX_POINT('',#26828);
#5608=VERTEX_POINT('',#26830);
#5609=VERTEX_POINT('',#26832);
#5610=VERTEX_POINT('',#26834);
#5611=VERTEX_POINT('',#26836);
#5612=VERTEX_POINT('',#26838);
#5613=VERTEX_POINT('',#26842);
#5614=VERTEX_POINT('',#26844);
#5615=VERTEX_POINT('',#26848);
#5616=VERTEX_POINT('',#26852);
#5617=VERTEX_POINT('',#26856);
#5618=VERTEX_POINT('',#26860);
#5619=VERTEX_POINT('',#26864);
#5620=VERTEX_POINT('',#26868);
#5621=VERTEX_POINT('',#26872);
#5622=VERTEX_POINT('',#26879);
#5623=VERTEX_POINT('',#26880);
#5624=VERTEX_POINT('',#26882);
#5625=VERTEX_POINT('',#26884);
#5626=VERTEX_POINT('',#26888);
#5627=VERTEX_POINT('',#26890);
#5628=VERTEX_POINT('',#26894);
#5629=VERTEX_POINT('',#26896);
#5630=VERTEX_POINT('',#26900);
#5631=VERTEX_POINT('',#26902);
#5632=VERTEX_POINT('',#26906);
#5633=VERTEX_POINT('',#26908);
#5634=VERTEX_POINT('',#26912);
#5635=VERTEX_POINT('',#26914);
#5636=VERTEX_POINT('',#26918);
#5637=VERTEX_POINT('',#26920);
#5638=VERTEX_POINT('',#26924);
#5639=VERTEX_POINT('',#26926);
#5640=VERTEX_POINT('',#26935);
#5641=VERTEX_POINT('',#26936);
#5642=VERTEX_POINT('',#26938);
#5643=VERTEX_POINT('',#26940);
#5644=VERTEX_POINT('',#26942);
#5645=VERTEX_POINT('',#26944);
#5646=VERTEX_POINT('',#26946);
#5647=VERTEX_POINT('',#26948);
#5648=VERTEX_POINT('',#26950);
#5649=VERTEX_POINT('',#26954);
#5650=VERTEX_POINT('',#26956);
#5651=VERTEX_POINT('',#26960);
#5652=VERTEX_POINT('',#26964);
#5653=VERTEX_POINT('',#26968);
#5654=VERTEX_POINT('',#26972);
#5655=VERTEX_POINT('',#26976);
#5656=VERTEX_POINT('',#26980);
#5657=VERTEX_POINT('',#26984);
#5658=VERTEX_POINT('',#26991);
#5659=VERTEX_POINT('',#26992);
#5660=VERTEX_POINT('',#26994);
#5661=VERTEX_POINT('',#26996);
#5662=VERTEX_POINT('',#26998);
#5663=VERTEX_POINT('',#27000);
#5664=VERTEX_POINT('',#27002);
#5665=VERTEX_POINT('',#27004);
#5666=VERTEX_POINT('',#27006);
#5667=VERTEX_POINT('',#27010);
#5668=VERTEX_POINT('',#27012);
#5669=VERTEX_POINT('',#27016);
#5670=VERTEX_POINT('',#27020);
#5671=VERTEX_POINT('',#27024);
#5672=VERTEX_POINT('',#27028);
#5673=VERTEX_POINT('',#27032);
#5674=VERTEX_POINT('',#27036);
#5675=VERTEX_POINT('',#27040);
#5676=VERTEX_POINT('',#27047);
#5677=VERTEX_POINT('',#27048);
#5678=VERTEX_POINT('',#27050);
#5679=VERTEX_POINT('',#27052);
#5680=VERTEX_POINT('',#27056);
#5681=VERTEX_POINT('',#27058);
#5682=VERTEX_POINT('',#27062);
#5683=VERTEX_POINT('',#27064);
#5684=VERTEX_POINT('',#27068);
#5685=VERTEX_POINT('',#27070);
#5686=VERTEX_POINT('',#27074);
#5687=VERTEX_POINT('',#27076);
#5688=VERTEX_POINT('',#27080);
#5689=VERTEX_POINT('',#27082);
#5690=VERTEX_POINT('',#27086);
#5691=VERTEX_POINT('',#27088);
#5692=VERTEX_POINT('',#27092);
#5693=VERTEX_POINT('',#27094);
#5694=VERTEX_POINT('',#27103);
#5695=VERTEX_POINT('',#27104);
#5696=VERTEX_POINT('',#27106);
#5697=VERTEX_POINT('',#27108);
#5698=VERTEX_POINT('',#27110);
#5699=VERTEX_POINT('',#27112);
#5700=VERTEX_POINT('',#27114);
#5701=VERTEX_POINT('',#27116);
#5702=VERTEX_POINT('',#27118);
#5703=VERTEX_POINT('',#27122);
#5704=VERTEX_POINT('',#27124);
#5705=VERTEX_POINT('',#27128);
#5706=VERTEX_POINT('',#27132);
#5707=VERTEX_POINT('',#27136);
#5708=VERTEX_POINT('',#27140);
#5709=VERTEX_POINT('',#27144);
#5710=VERTEX_POINT('',#27148);
#5711=VERTEX_POINT('',#27152);
#5712=VERTEX_POINT('',#27159);
#5713=VERTEX_POINT('',#27160);
#5714=VERTEX_POINT('',#27162);
#5715=VERTEX_POINT('',#27164);
#5716=VERTEX_POINT('',#27168);
#5717=VERTEX_POINT('',#27169);
#5718=VERTEX_POINT('',#27171);
#5719=VERTEX_POINT('',#27173);
#5720=VERTEX_POINT('',#27177);
#5721=VERTEX_POINT('',#27178);
#5722=VERTEX_POINT('',#27180);
#5723=VERTEX_POINT('',#27182);
#5724=VERTEX_POINT('',#27186);
#5725=VERTEX_POINT('',#27187);
#5726=VERTEX_POINT('',#27189);
#5727=VERTEX_POINT('',#27191);
#5728=VERTEX_POINT('',#27195);
#5729=VERTEX_POINT('',#27196);
#5730=VERTEX_POINT('',#27198);
#5731=VERTEX_POINT('',#27200);
#5732=VERTEX_POINT('',#27204);
#5733=VERTEX_POINT('',#27205);
#5734=VERTEX_POINT('',#27207);
#5735=VERTEX_POINT('',#27209);
#5736=VERTEX_POINT('',#27213);
#5737=VERTEX_POINT('',#27214);
#5738=VERTEX_POINT('',#27216);
#5739=VERTEX_POINT('',#27218);
#5740=VERTEX_POINT('',#27222);
#5741=VERTEX_POINT('',#27223);
#5742=VERTEX_POINT('',#27225);
#5743=VERTEX_POINT('',#27227);
#5744=VERTEX_POINT('',#27235);
#5745=VERTEX_POINT('',#27237);
#5746=VERTEX_POINT('',#27240);
#5747=VERTEX_POINT('',#27242);
#5748=VERTEX_POINT('',#27245);
#5749=VERTEX_POINT('',#27247);
#5750=VERTEX_POINT('',#27250);
#5751=VERTEX_POINT('',#27252);
#5752=VERTEX_POINT('',#27260);
#5753=VERTEX_POINT('',#27262);
#5754=VERTEX_POINT('',#27265);
#5755=VERTEX_POINT('',#27267);
#5756=VERTEX_POINT('',#27270);
#5757=VERTEX_POINT('',#27272);
#5758=VERTEX_POINT('',#27275);
#5759=VERTEX_POINT('',#27277);
#5760=VERTEX_POINT('',#27305);
#5761=VERTEX_POINT('',#27307);
#5762=VERTEX_POINT('',#27311);
#5763=VERTEX_POINT('',#27313);
#5764=VERTEX_POINT('',#27317);
#5765=VERTEX_POINT('',#27318);
#5766=VERTEX_POINT('',#27320);
#5767=VERTEX_POINT('',#27322);
#5768=VERTEX_POINT('',#27326);
#5769=VERTEX_POINT('',#27328);
#5770=VERTEX_POINT('',#27332);
#5771=VERTEX_POINT('',#27334);
#5772=VERTEX_POINT('',#27338);
#5773=VERTEX_POINT('',#27340);
#5774=VERTEX_POINT('',#27344);
#5775=VERTEX_POINT('',#27346);
#5776=VERTEX_POINT('',#27350);
#5777=VERTEX_POINT('',#27352);
#5778=VERTEX_POINT('',#27356);
#5779=VERTEX_POINT('',#27358);
#5780=VERTEX_POINT('',#27362);
#5781=VERTEX_POINT('',#27364);
#5782=VERTEX_POINT('',#27368);
#5783=VERTEX_POINT('',#27370);
#5784=VERTEX_POINT('',#27374);
#5785=VERTEX_POINT('',#27376);
#5786=VERTEX_POINT('',#27380);
#5787=VERTEX_POINT('',#27382);
#5788=VERTEX_POINT('',#27391);
#5789=VERTEX_POINT('',#27393);
#5790=VERTEX_POINT('',#27397);
#5791=VERTEX_POINT('',#27399);
#5792=VERTEX_POINT('',#27403);
#5793=VERTEX_POINT('',#27404);
#5794=VERTEX_POINT('',#27406);
#5795=VERTEX_POINT('',#27408);
#5796=VERTEX_POINT('',#27412);
#5797=VERTEX_POINT('',#27414);
#5798=VERTEX_POINT('',#27418);
#5799=VERTEX_POINT('',#27420);
#5800=VERTEX_POINT('',#27424);
#5801=VERTEX_POINT('',#27426);
#5802=VERTEX_POINT('',#27430);
#5803=VERTEX_POINT('',#27432);
#5804=VERTEX_POINT('',#27436);
#5805=VERTEX_POINT('',#27438);
#5806=VERTEX_POINT('',#27442);
#5807=VERTEX_POINT('',#27444);
#5808=VERTEX_POINT('',#27448);
#5809=VERTEX_POINT('',#27450);
#5810=VERTEX_POINT('',#27459);
#5811=VERTEX_POINT('',#27461);
#5812=VERTEX_POINT('',#27465);
#5813=VERTEX_POINT('',#27467);
#5814=VERTEX_POINT('',#27471);
#5815=VERTEX_POINT('',#27472);
#5816=VERTEX_POINT('',#27474);
#5817=VERTEX_POINT('',#27476);
#5818=VERTEX_POINT('',#27480);
#5819=VERTEX_POINT('',#27482);
#5820=VERTEX_POINT('',#27486);
#5821=VERTEX_POINT('',#27488);
#5822=VERTEX_POINT('',#27492);
#5823=VERTEX_POINT('',#27494);
#5824=VERTEX_POINT('',#27498);
#5825=VERTEX_POINT('',#27500);
#5826=VERTEX_POINT('',#27504);
#5827=VERTEX_POINT('',#27506);
#5828=VERTEX_POINT('',#27510);
#5829=VERTEX_POINT('',#27512);
#5830=VERTEX_POINT('',#27516);
#5831=VERTEX_POINT('',#27518);
#6718=EDGE_CURVE('',#5292,#5293,#3134,.T.);
#6719=EDGE_CURVE('',#5294,#5292,#3135,.T.);
#6720=EDGE_CURVE('',#5295,#5294,#3136,.T.);
#6721=EDGE_CURVE('',#5295,#5293,#3137,.T.);
#6722=EDGE_CURVE('',#5296,#5292,#3138,.T.);
#6723=EDGE_CURVE('',#5297,#5296,#3139,.T.);
#6724=EDGE_CURVE('',#5294,#5297,#3140,.T.);
#6725=EDGE_CURVE('',#5298,#5296,#2572,.T.);
#6726=EDGE_CURVE('',#5299,#5298,#3141,.T.);
#6727=EDGE_CURVE('',#5297,#5299,#2573,.T.);
#6728=EDGE_CURVE('',#5300,#5298,#3142,.T.);
#6729=EDGE_CURVE('',#5301,#5300,#3143,.T.);
#6730=EDGE_CURVE('',#5299,#5301,#3144,.T.);
#6731=EDGE_CURVE('',#5302,#5300,#2574,.T.);
#6732=EDGE_CURVE('',#5303,#5302,#3145,.T.);
#6733=EDGE_CURVE('',#5301,#5303,#2575,.T.);
#6734=EDGE_CURVE('',#5304,#5302,#3146,.T.);
#6735=EDGE_CURVE('',#5305,#5304,#3147,.T.);
#6736=EDGE_CURVE('',#5303,#5305,#3148,.T.);
#6737=EDGE_CURVE('',#5306,#5304,#2576,.T.);
#6738=EDGE_CURVE('',#5307,#5306,#3149,.T.);
#6739=EDGE_CURVE('',#5305,#5307,#2577,.T.);
#6740=EDGE_CURVE('',#5308,#5306,#3150,.T.);
#6741=EDGE_CURVE('',#5309,#5308,#3151,.T.);
#6742=EDGE_CURVE('',#5307,#5309,#3152,.T.);
#6743=EDGE_CURVE('',#5310,#5308,#2578,.T.);
#6744=EDGE_CURVE('',#5311,#5310,#3153,.T.);
#6745=EDGE_CURVE('',#5309,#5311,#2579,.T.);
#6746=EDGE_CURVE('',#5312,#5310,#3154,.T.);
#6747=EDGE_CURVE('',#5313,#5312,#3155,.T.);
#6748=EDGE_CURVE('',#5311,#5313,#3156,.T.);
#6749=EDGE_CURVE('',#5314,#5312,#3157,.T.);
#6750=EDGE_CURVE('',#5315,#5314,#3158,.T.);
#6751=EDGE_CURVE('',#5313,#5315,#3159,.T.);
#6752=EDGE_CURVE('',#5293,#5314,#3160,.T.);
#6753=EDGE_CURVE('',#5315,#5295,#3161,.T.);
#6754=EDGE_CURVE('',#5316,#5317,#3162,.T.);
#6755=EDGE_CURVE('',#5317,#5318,#2580,.T.);
#6756=EDGE_CURVE('',#5318,#5319,#3163,.T.);
#6757=EDGE_CURVE('',#5319,#5320,#2581,.T.);
#6758=EDGE_CURVE('',#5320,#5321,#3164,.T.);
#6759=EDGE_CURVE('',#5321,#5322,#2582,.T.);
#6760=EDGE_CURVE('',#5322,#5323,#3165,.T.);
#6761=EDGE_CURVE('',#5323,#5324,#2583,.T.);
#6762=EDGE_CURVE('',#5324,#5325,#3166,.T.);
#6763=EDGE_CURVE('',#5326,#5325,#3167,.T.);
#6764=EDGE_CURVE('',#5326,#5327,#3168,.T.);
#6765=EDGE_CURVE('',#5327,#5316,#3169,.T.);
#6766=EDGE_CURVE('',#5326,#5328,#3170,.T.);
#6767=EDGE_CURVE('',#5328,#5329,#3171,.T.);
#6768=EDGE_CURVE('',#5327,#5329,#3172,.T.);
#6769=EDGE_CURVE('',#5325,#5330,#3173,.T.);
#6770=EDGE_CURVE('',#5330,#5328,#3174,.T.);
#6771=EDGE_CURVE('',#5324,#5331,#3175,.T.);
#6772=EDGE_CURVE('',#5331,#5330,#3176,.T.);
#6773=EDGE_CURVE('',#5323,#5332,#3177,.T.);
#6774=EDGE_CURVE('',#5332,#5331,#133,.T.);
#6775=EDGE_CURVE('',#5322,#5333,#3178,.T.);
#6776=EDGE_CURVE('',#5333,#5332,#3179,.T.);
#6777=EDGE_CURVE('',#5321,#5334,#3180,.T.);
#6778=EDGE_CURVE('',#5334,#5333,#134,.T.);
#6779=EDGE_CURVE('',#5320,#5335,#3181,.T.);
#6780=EDGE_CURVE('',#5335,#5334,#3182,.T.);
#6781=EDGE_CURVE('',#5319,#5336,#3183,.T.);
#6782=EDGE_CURVE('',#5336,#5335,#135,.T.);
#6783=EDGE_CURVE('',#5318,#5337,#3184,.T.);
#6784=EDGE_CURVE('',#5337,#5336,#3185,.T.);
#6785=EDGE_CURVE('',#5317,#5338,#3186,.T.);
#6786=EDGE_CURVE('',#5338,#5337,#136,.T.);
#6787=EDGE_CURVE('',#5316,#5339,#3187,.T.);
#6788=EDGE_CURVE('',#5339,#5338,#3188,.T.);
#6789=EDGE_CURVE('',#5329,#5339,#3189,.T.);
#6790=EDGE_CURVE('',#5340,#5341,#3190,.T.);
#6791=EDGE_CURVE('',#5341,#5342,#3191,.T.);
#6792=EDGE_CURVE('',#5342,#5343,#3192,.T.);
#6793=EDGE_CURVE('',#5343,#5344,#3193,.T.);
#6794=EDGE_CURVE('',#5344,#5345,#3194,.T.);
#6795=EDGE_CURVE('',#5345,#5346,#137,.T.);
#6796=EDGE_CURVE('',#5346,#5347,#3195,.T.);
#6797=EDGE_CURVE('',#5347,#5348,#138,.T.);
#6798=EDGE_CURVE('',#5348,#5349,#3196,.T.);
#6799=EDGE_CURVE('',#5349,#5350,#139,.T.);
#6800=EDGE_CURVE('',#5350,#5351,#3197,.T.);
#6801=EDGE_CURVE('',#5351,#5340,#140,.T.);
#6802=EDGE_CURVE('',#5352,#5342,#3198,.T.);
#6803=EDGE_CURVE('',#5352,#5353,#3199,.T.);
#6804=EDGE_CURVE('',#5353,#5343,#3200,.T.);
#6805=EDGE_CURVE('',#5353,#5354,#3201,.T.);
#6806=EDGE_CURVE('',#5354,#5344,#3202,.T.);
#6807=EDGE_CURVE('',#5354,#5355,#3203,.T.);
#6808=EDGE_CURVE('',#5355,#5345,#3204,.T.);
#6809=EDGE_CURVE('',#5355,#5356,#141,.T.);
#6810=EDGE_CURVE('',#5356,#5346,#3205,.T.);
#6811=EDGE_CURVE('',#5356,#5357,#3206,.T.);
#6812=EDGE_CURVE('',#5357,#5347,#3207,.T.);
#6813=EDGE_CURVE('',#5357,#5358,#142,.T.);
#6814=EDGE_CURVE('',#5358,#5348,#3208,.T.);
#6815=EDGE_CURVE('',#5358,#5359,#3209,.T.);
#6816=EDGE_CURVE('',#5359,#5349,#3210,.T.);
#6817=EDGE_CURVE('',#5359,#5360,#143,.T.);
#6818=EDGE_CURVE('',#5360,#5350,#3211,.T.);
#6819=EDGE_CURVE('',#5360,#5361,#3212,.T.);
#6820=EDGE_CURVE('',#5361,#5351,#3213,.T.);
#6821=EDGE_CURVE('',#5361,#5362,#144,.T.);
#6822=EDGE_CURVE('',#5362,#5340,#3214,.T.);
#6823=EDGE_CURVE('',#5362,#5363,#3215,.T.);
#6824=EDGE_CURVE('',#5363,#5341,#3216,.T.);
#6825=EDGE_CURVE('',#5363,#5352,#3217,.T.);
#6826=EDGE_CURVE('',#5364,#5365,#3218,.T.);
#6827=EDGE_CURVE('',#5365,#5366,#3219,.T.);
#6828=EDGE_CURVE('',#5367,#5366,#3220,.T.);
#6829=EDGE_CURVE('',#5364,#5367,#3221,.T.);
#6830=EDGE_CURVE('',#5364,#5368,#3222,.T.);
#6831=EDGE_CURVE('',#5369,#5367,#3223,.T.);
#6832=EDGE_CURVE('',#5368,#5369,#3224,.T.);
#6833=EDGE_CURVE('',#5368,#5370,#2584,.T.);
#6834=EDGE_CURVE('',#5371,#5369,#145,.T.);
#6835=EDGE_CURVE('',#5370,#5371,#3225,.T.);
#6836=EDGE_CURVE('',#5370,#5372,#3226,.T.);
#6837=EDGE_CURVE('',#5373,#5371,#3227,.T.);
#6838=EDGE_CURVE('',#5372,#5373,#3228,.T.);
#6839=EDGE_CURVE('',#5372,#5374,#2585,.T.);
#6840=EDGE_CURVE('',#5375,#5373,#146,.T.);
#6841=EDGE_CURVE('',#5374,#5375,#3229,.T.);
#6842=EDGE_CURVE('',#5374,#5376,#3230,.T.);
#6843=EDGE_CURVE('',#5377,#5375,#3231,.T.);
#6844=EDGE_CURVE('',#5376,#5377,#3232,.T.);
#6845=EDGE_CURVE('',#5376,#5378,#2586,.T.);
#6846=EDGE_CURVE('',#5379,#5377,#147,.T.);
#6847=EDGE_CURVE('',#5378,#5379,#3233,.T.);
#6848=EDGE_CURVE('',#5378,#5380,#3234,.T.);
#6849=EDGE_CURVE('',#5381,#5379,#3235,.T.);
#6850=EDGE_CURVE('',#5380,#5381,#3236,.T.);
#6851=EDGE_CURVE('',#5380,#5382,#2587,.T.);
#6852=EDGE_CURVE('',#5383,#5381,#148,.T.);
#6853=EDGE_CURVE('',#5382,#5383,#3237,.T.);
#6854=EDGE_CURVE('',#5382,#5384,#3238,.T.);
#6855=EDGE_CURVE('',#5385,#5383,#3239,.T.);
#6856=EDGE_CURVE('',#5384,#5385,#3240,.T.);
#6857=EDGE_CURVE('',#5384,#5386,#3241,.T.);
#6858=EDGE_CURVE('',#5387,#5385,#3242,.T.);
#6859=EDGE_CURVE('',#5386,#5387,#3243,.T.);
#6860=EDGE_CURVE('',#5386,#5365,#3244,.T.);
#6861=EDGE_CURVE('',#5366,#5387,#3245,.T.);
#6862=EDGE_CURVE('',#5388,#5389,#3246,.T.);
#6863=EDGE_CURVE('',#5390,#5388,#3247,.T.);
#6864=EDGE_CURVE('',#5391,#5390,#3248,.T.);
#6865=EDGE_CURVE('',#5391,#5389,#3249,.T.);
#6866=EDGE_CURVE('',#5392,#5388,#3250,.T.);
#6867=EDGE_CURVE('',#5393,#5392,#3251,.T.);
#6868=EDGE_CURVE('',#5390,#5393,#3252,.T.);
#6869=EDGE_CURVE('',#5394,#5392,#2588,.T.);
#6870=EDGE_CURVE('',#5395,#5394,#3253,.T.);
#6871=EDGE_CURVE('',#5393,#5395,#2589,.T.);
#6872=EDGE_CURVE('',#5396,#5394,#3254,.T.);
#6873=EDGE_CURVE('',#5397,#5396,#3255,.T.);
#6874=EDGE_CURVE('',#5395,#5397,#3256,.T.);
#6875=EDGE_CURVE('',#5398,#5396,#2590,.T.);
#6876=EDGE_CURVE('',#5399,#5398,#3257,.T.);
#6877=EDGE_CURVE('',#5397,#5399,#2591,.T.);
#6878=EDGE_CURVE('',#5400,#5398,#3258,.T.);
#6879=EDGE_CURVE('',#5401,#5400,#3259,.T.);
#6880=EDGE_CURVE('',#5399,#5401,#3260,.T.);
#6881=EDGE_CURVE('',#5402,#5400,#2592,.T.);
#6882=EDGE_CURVE('',#5403,#5402,#3261,.T.);
#6883=EDGE_CURVE('',#5401,#5403,#2593,.T.);
#6884=EDGE_CURVE('',#5404,#5402,#3262,.T.);
#6885=EDGE_CURVE('',#5405,#5404,#3263,.T.);
#6886=EDGE_CURVE('',#5403,#5405,#3264,.T.);
#6887=EDGE_CURVE('',#5406,#5404,#2594,.T.);
#6888=EDGE_CURVE('',#5407,#5406,#3265,.T.);
#6889=EDGE_CURVE('',#5405,#5407,#2595,.T.);
#6890=EDGE_CURVE('',#5408,#5406,#3266,.T.);
#6891=EDGE_CURVE('',#5409,#5408,#3267,.T.);
#6892=EDGE_CURVE('',#5407,#5409,#3268,.T.);
#6893=EDGE_CURVE('',#5410,#5408,#3269,.T.);
#6894=EDGE_CURVE('',#5411,#5410,#3270,.T.);
#6895=EDGE_CURVE('',#5409,#5411,#3271,.T.);
#6896=EDGE_CURVE('',#5389,#5410,#3272,.T.);
#6897=EDGE_CURVE('',#5411,#5391,#3273,.T.);
#6898=EDGE_CURVE('',#5412,#5413,#3274,.T.);
#6899=EDGE_CURVE('',#5413,#5414,#3275,.T.);
#6900=EDGE_CURVE('',#5414,#5415,#3276,.T.);
#6901=EDGE_CURVE('',#5416,#5415,#3277,.T.);
#6902=EDGE_CURVE('',#5416,#5417,#3278,.T.);
#6903=EDGE_CURVE('',#5417,#5418,#2596,.T.);
#6904=EDGE_CURVE('',#5418,#5419,#3279,.T.);
#6905=EDGE_CURVE('',#5419,#5420,#2597,.T.);
#6906=EDGE_CURVE('',#5420,#5421,#3280,.T.);
#6907=EDGE_CURVE('',#5421,#5422,#2598,.T.);
#6908=EDGE_CURVE('',#5422,#5423,#3281,.T.);
#6909=EDGE_CURVE('',#5423,#5412,#2599,.T.);
#6910=EDGE_CURVE('',#5424,#5414,#3282,.T.);
#6911=EDGE_CURVE('',#5424,#5425,#3283,.T.);
#6912=EDGE_CURVE('',#5425,#5415,#3284,.T.);
#6913=EDGE_CURVE('',#5425,#5426,#3285,.T.);
#6914=EDGE_CURVE('',#5426,#5416,#3286,.T.);
#6915=EDGE_CURVE('',#5426,#5427,#3287,.T.);
#6916=EDGE_CURVE('',#5427,#5417,#3288,.T.);
#6917=EDGE_CURVE('',#5427,#5428,#149,.T.);
#6918=EDGE_CURVE('',#5428,#5418,#3289,.T.);
#6919=EDGE_CURVE('',#5428,#5429,#3290,.T.);
#6920=EDGE_CURVE('',#5429,#5419,#3291,.T.);
#6921=EDGE_CURVE('',#5429,#5430,#150,.T.);
#6922=EDGE_CURVE('',#5430,#5420,#3292,.T.);
#6923=EDGE_CURVE('',#5430,#5431,#3293,.T.);
#6924=EDGE_CURVE('',#5431,#5421,#3294,.T.);
#6925=EDGE_CURVE('',#5431,#5432,#151,.T.);
#6926=EDGE_CURVE('',#5432,#5422,#3295,.T.);
#6927=EDGE_CURVE('',#5432,#5433,#3296,.T.);
#6928=EDGE_CURVE('',#5433,#5423,#3297,.T.);
#6929=EDGE_CURVE('',#5433,#5434,#152,.T.);
#6930=EDGE_CURVE('',#5434,#5412,#3298,.T.);
#6931=EDGE_CURVE('',#5434,#5435,#3299,.T.);
#6932=EDGE_CURVE('',#5435,#5413,#3300,.T.);
#6933=EDGE_CURVE('',#5435,#5424,#3301,.T.);
#6934=EDGE_CURVE('',#5436,#5437,#3302,.T.);
#6935=EDGE_CURVE('',#5438,#5436,#3303,.T.);
#6936=EDGE_CURVE('',#5439,#5438,#3304,.T.);
#6937=EDGE_CURVE('',#5439,#5437,#3305,.T.);
#6938=EDGE_CURVE('',#5440,#5436,#3306,.T.);
#6939=EDGE_CURVE('',#5441,#5440,#3307,.T.);
#6940=EDGE_CURVE('',#5438,#5441,#3308,.T.);
#6941=EDGE_CURVE('',#5442,#5440,#153,.T.);
#6942=EDGE_CURVE('',#5443,#5442,#3309,.T.);
#6943=EDGE_CURVE('',#5441,#5443,#2600,.T.);
#6944=EDGE_CURVE('',#5444,#5442,#3310,.T.);
#6945=EDGE_CURVE('',#5445,#5444,#3311,.T.);
#6946=EDGE_CURVE('',#5443,#5445,#3312,.T.);
#6947=EDGE_CURVE('',#5446,#5444,#154,.T.);
#6948=EDGE_CURVE('',#5447,#5446,#3313,.T.);
#6949=EDGE_CURVE('',#5445,#5447,#2601,.T.);
#6950=EDGE_CURVE('',#5448,#5446,#3314,.T.);
#6951=EDGE_CURVE('',#5449,#5448,#3315,.T.);
#6952=EDGE_CURVE('',#5447,#5449,#3316,.T.);
#6953=EDGE_CURVE('',#5450,#5448,#155,.T.);
#6954=EDGE_CURVE('',#5451,#5450,#3317,.T.);
#6955=EDGE_CURVE('',#5449,#5451,#2602,.T.);
#6956=EDGE_CURVE('',#5452,#5450,#3318,.T.);
#6957=EDGE_CURVE('',#5453,#5452,#3319,.T.);
#6958=EDGE_CURVE('',#5451,#5453,#3320,.T.);
#6959=EDGE_CURVE('',#5454,#5452,#156,.T.);
#6960=EDGE_CURVE('',#5455,#5454,#3321,.T.);
#6961=EDGE_CURVE('',#5453,#5455,#2603,.T.);
#6962=EDGE_CURVE('',#5456,#5454,#3322,.T.);
#6963=EDGE_CURVE('',#5457,#5456,#3323,.T.);
#6964=EDGE_CURVE('',#5455,#5457,#3324,.T.);
#6965=EDGE_CURVE('',#5458,#5456,#3325,.T.);
#6966=EDGE_CURVE('',#5459,#5458,#3326,.T.);
#6967=EDGE_CURVE('',#5459,#5457,#3327,.T.);
#6968=EDGE_CURVE('',#5437,#5458,#3328,.T.);
#6969=EDGE_CURVE('',#5459,#5439,#3329,.T.);
#6970=EDGE_CURVE('',#5460,#5461,#3330,.T.);
#6971=EDGE_CURVE('',#5461,#5462,#3331,.T.);
#6972=EDGE_CURVE('',#5462,#5463,#3332,.T.);
#6973=EDGE_CURVE('',#5463,#5464,#3333,.T.);
#6974=EDGE_CURVE('',#5464,#5465,#3334,.T.);
#6975=EDGE_CURVE('',#5465,#5466,#157,.T.);
#6976=EDGE_CURVE('',#5466,#5467,#3335,.T.);
#6977=EDGE_CURVE('',#5467,#5468,#158,.T.);
#6978=EDGE_CURVE('',#5468,#5469,#3336,.T.);
#6979=EDGE_CURVE('',#5469,#5470,#159,.T.);
#6980=EDGE_CURVE('',#5470,#5471,#3337,.T.);
#6981=EDGE_CURVE('',#5471,#5460,#160,.T.);
#6982=EDGE_CURVE('',#5472,#5462,#3338,.T.);
#6983=EDGE_CURVE('',#5472,#5473,#3339,.T.);
#6984=EDGE_CURVE('',#5473,#5463,#3340,.T.);
#6985=EDGE_CURVE('',#5473,#5474,#3341,.T.);
#6986=EDGE_CURVE('',#5474,#5464,#3342,.T.);
#6987=EDGE_CURVE('',#5474,#5475,#3343,.T.);
#6988=EDGE_CURVE('',#5475,#5465,#3344,.T.);
#6989=EDGE_CURVE('',#5475,#5476,#161,.T.);
#6990=EDGE_CURVE('',#5476,#5466,#3345,.T.);
#6991=EDGE_CURVE('',#5476,#5477,#3346,.T.);
#6992=EDGE_CURVE('',#5477,#5467,#3347,.T.);
#6993=EDGE_CURVE('',#5477,#5478,#162,.T.);
#6994=EDGE_CURVE('',#5478,#5468,#3348,.T.);
#6995=EDGE_CURVE('',#5478,#5479,#3349,.T.);
#6996=EDGE_CURVE('',#5479,#5469,#3350,.T.);
#6997=EDGE_CURVE('',#5479,#5480,#163,.T.);
#6998=EDGE_CURVE('',#5480,#5470,#3351,.T.);
#6999=EDGE_CURVE('',#5480,#5481,#3352,.T.);
#7000=EDGE_CURVE('',#5481,#5471,#3353,.T.);
#7001=EDGE_CURVE('',#5481,#5482,#164,.T.);
#7002=EDGE_CURVE('',#5482,#5460,#3354,.T.);
#7003=EDGE_CURVE('',#5482,#5483,#3355,.T.);
#7004=EDGE_CURVE('',#5483,#5461,#3356,.T.);
#7005=EDGE_CURVE('',#5483,#5472,#3357,.T.);
#7006=EDGE_CURVE('',#5484,#5485,#3358,.T.);
#7007=EDGE_CURVE('',#5485,#5486,#3359,.T.);
#7008=EDGE_CURVE('',#5486,#5487,#2604,.T.);
#7009=EDGE_CURVE('',#5487,#5488,#3360,.T.);
#7010=EDGE_CURVE('',#5488,#5489,#2605,.T.);
#7011=EDGE_CURVE('',#5489,#5490,#3361,.T.);
#7012=EDGE_CURVE('',#5490,#5491,#2606,.T.);
#7013=EDGE_CURVE('',#5491,#5492,#3362,.T.);
#7014=EDGE_CURVE('',#5492,#5493,#2607,.T.);
#7015=EDGE_CURVE('',#5493,#5494,#3363,.T.);
#7016=EDGE_CURVE('',#5494,#5495,#3364,.T.);
#7017=EDGE_CURVE('',#5495,#5484,#3365,.T.);
#7018=EDGE_CURVE('',#5495,#5496,#3366,.T.);
#7019=EDGE_CURVE('',#5496,#5497,#3367,.T.);
#7020=EDGE_CURVE('',#5484,#5497,#3368,.T.);
#7021=EDGE_CURVE('',#5494,#5498,#3369,.T.);
#7022=EDGE_CURVE('',#5498,#5496,#3370,.T.);
#7023=EDGE_CURVE('',#5493,#5499,#3371,.T.);
#7024=EDGE_CURVE('',#5499,#5498,#3372,.T.);
#7025=EDGE_CURVE('',#5492,#5500,#3373,.T.);
#7026=EDGE_CURVE('',#5500,#5499,#165,.T.);
#7027=EDGE_CURVE('',#5491,#5501,#3374,.T.);
#7028=EDGE_CURVE('',#5501,#5500,#3375,.T.);
#7029=EDGE_CURVE('',#5490,#5502,#3376,.T.);
#7030=EDGE_CURVE('',#5502,#5501,#166,.T.);
#7031=EDGE_CURVE('',#5489,#5503,#3377,.T.);
#7032=EDGE_CURVE('',#5503,#5502,#3378,.T.);
#7033=EDGE_CURVE('',#5488,#5504,#3379,.T.);
#7034=EDGE_CURVE('',#5504,#5503,#167,.T.);
#7035=EDGE_CURVE('',#5487,#5505,#3380,.T.);
#7036=EDGE_CURVE('',#5505,#5504,#3381,.T.);
#7037=EDGE_CURVE('',#5486,#5506,#3382,.T.);
#7038=EDGE_CURVE('',#5506,#5505,#168,.T.);
#7039=EDGE_CURVE('',#5485,#5507,#3383,.T.);
#7040=EDGE_CURVE('',#5507,#5506,#3384,.T.);
#7041=EDGE_CURVE('',#5497,#5507,#3385,.T.);
#7042=EDGE_CURVE('',#5508,#5509,#3386,.T.);
#7043=EDGE_CURVE('',#5510,#5508,#3387,.T.);
#7044=EDGE_CURVE('',#5511,#5510,#3388,.T.);
#7045=EDGE_CURVE('',#5512,#5511,#3389,.T.);
#7046=EDGE_CURVE('',#5513,#5512,#2608,.T.);
#7047=EDGE_CURVE('',#5514,#5513,#3390,.T.);
#7048=EDGE_CURVE('',#5515,#5514,#2609,.T.);
#7049=EDGE_CURVE('',#5516,#5515,#3391,.T.);
#7050=EDGE_CURVE('',#5517,#5516,#2610,.T.);
#7051=EDGE_CURVE('',#5518,#5517,#3392,.T.);
#7052=EDGE_CURVE('',#5519,#5518,#2611,.T.);
#7053=EDGE_CURVE('',#5509,#5519,#3393,.T.);
#7054=EDGE_CURVE('',#5520,#5508,#3394,.T.);
#7055=EDGE_CURVE('',#5520,#5521,#3395,.T.);
#7056=EDGE_CURVE('',#5521,#5510,#3396,.T.);
#7057=EDGE_CURVE('',#5521,#5522,#3397,.T.);
#7058=EDGE_CURVE('',#5522,#5511,#3398,.T.);
#7059=EDGE_CURVE('',#5522,#5523,#3399,.T.);
#7060=EDGE_CURVE('',#5523,#5512,#3400,.T.);
#7061=EDGE_CURVE('',#5523,#5524,#169,.T.);
#7062=EDGE_CURVE('',#5524,#5513,#3401,.T.);
#7063=EDGE_CURVE('',#5524,#5525,#3402,.T.);
#7064=EDGE_CURVE('',#5525,#5514,#3403,.T.);
#7065=EDGE_CURVE('',#5525,#5526,#170,.T.);
#7066=EDGE_CURVE('',#5526,#5515,#3404,.T.);
#7067=EDGE_CURVE('',#5526,#5527,#3405,.T.);
#7068=EDGE_CURVE('',#5527,#5516,#3406,.T.);
#7069=EDGE_CURVE('',#5527,#5528,#171,.T.);
#7070=EDGE_CURVE('',#5528,#5517,#3407,.T.);
#7071=EDGE_CURVE('',#5528,#5529,#3408,.T.);
#7072=EDGE_CURVE('',#5529,#5518,#3409,.T.);
#7073=EDGE_CURVE('',#5529,#5530,#172,.T.);
#7074=EDGE_CURVE('',#5530,#5519,#3410,.T.);
#7075=EDGE_CURVE('',#5530,#5531,#3411,.T.);
#7076=EDGE_CURVE('',#5531,#5509,#3412,.T.);
#7077=EDGE_CURVE('',#5531,#5520,#3413,.T.);
#7078=EDGE_CURVE('',#5532,#5533,#3414,.T.);
#7079=EDGE_CURVE('',#5534,#5533,#3415,.T.);
#7080=EDGE_CURVE('',#5535,#5534,#3416,.T.);
#7081=EDGE_CURVE('',#5535,#5532,#3417,.T.);
#7082=EDGE_CURVE('',#5533,#5536,#3418,.T.);
#7083=EDGE_CURVE('',#5537,#5536,#3419,.T.);
#7084=EDGE_CURVE('',#5534,#5537,#3420,.T.);
#7085=EDGE_CURVE('',#5536,#5538,#2612,.T.);
#7086=EDGE_CURVE('',#5539,#5538,#3421,.T.);
#7087=EDGE_CURVE('',#5537,#5539,#2613,.T.);
#7088=EDGE_CURVE('',#5538,#5540,#3422,.T.);
#7089=EDGE_CURVE('',#5541,#5540,#3423,.T.);
#7090=EDGE_CURVE('',#5539,#5541,#3424,.T.);
#7091=EDGE_CURVE('',#5540,#5542,#2614,.T.);
#7092=EDGE_CURVE('',#5543,#5542,#3425,.T.);
#7093=EDGE_CURVE('',#5541,#5543,#2615,.T.);
#7094=EDGE_CURVE('',#5542,#5544,#3426,.T.);
#7095=EDGE_CURVE('',#5545,#5544,#3427,.T.);
#7096=EDGE_CURVE('',#5543,#5545,#3428,.T.);
#7097=EDGE_CURVE('',#5544,#5546,#2616,.T.);
#7098=EDGE_CURVE('',#5547,#5546,#3429,.T.);
#7099=EDGE_CURVE('',#5545,#5547,#2617,.T.);
#7100=EDGE_CURVE('',#5546,#5548,#3430,.T.);
#7101=EDGE_CURVE('',#5549,#5548,#3431,.T.);
#7102=EDGE_CURVE('',#5547,#5549,#3432,.T.);
#7103=EDGE_CURVE('',#5548,#5532,#3433,.T.);
#7104=EDGE_CURVE('',#5549,#5535,#3434,.T.);
#7105=EDGE_CURVE('',#5550,#5551,#3435,.T.);
#7106=EDGE_CURVE('',#5552,#5551,#3436,.T.);
#7107=EDGE_CURVE('',#5553,#5552,#3437,.T.);
#7108=EDGE_CURVE('',#5553,#5550,#3438,.T.);
#7109=EDGE_CURVE('',#5551,#5554,#3439,.T.);
#7110=EDGE_CURVE('',#5555,#5554,#3440,.T.);
#7111=EDGE_CURVE('',#5552,#5555,#3441,.T.);
#7112=EDGE_CURVE('',#5554,#5556,#2618,.T.);
#7113=EDGE_CURVE('',#5557,#5556,#3442,.T.);
#7114=EDGE_CURVE('',#5555,#5557,#2619,.T.);
#7115=EDGE_CURVE('',#5556,#5558,#3443,.T.);
#7116=EDGE_CURVE('',#5559,#5558,#3444,.T.);
#7117=EDGE_CURVE('',#5557,#5559,#3445,.T.);
#7118=EDGE_CURVE('',#5558,#5560,#2620,.T.);
#7119=EDGE_CURVE('',#5561,#5560,#3446,.T.);
#7120=EDGE_CURVE('',#5559,#5561,#2621,.T.);
#7121=EDGE_CURVE('',#5560,#5562,#3447,.T.);
#7122=EDGE_CURVE('',#5563,#5562,#3448,.T.);
#7123=EDGE_CURVE('',#5561,#5563,#3449,.T.);
#7124=EDGE_CURVE('',#5562,#5564,#2622,.T.);
#7125=EDGE_CURVE('',#5565,#5564,#3450,.T.);
#7126=EDGE_CURVE('',#5563,#5565,#2623,.T.);
#7127=EDGE_CURVE('',#5564,#5566,#3451,.T.);
#7128=EDGE_CURVE('',#5567,#5566,#3452,.T.);
#7129=EDGE_CURVE('',#5565,#5567,#3453,.T.);
#7130=EDGE_CURVE('',#5566,#5550,#3454,.T.);
#7131=EDGE_CURVE('',#5567,#5553,#3455,.T.);
#7132=EDGE_CURVE('',#5568,#5569,#3456,.T.);
#7133=EDGE_CURVE('',#5570,#5568,#3457,.T.);
#7134=EDGE_CURVE('',#5570,#5571,#3458,.T.);
#7135=EDGE_CURVE('',#5571,#5569,#3459,.T.);
#7136=EDGE_CURVE('',#5569,#5572,#3460,.T.);
#7137=EDGE_CURVE('',#5571,#5573,#3461,.T.);
#7138=EDGE_CURVE('',#5573,#5572,#3462,.T.);
#7139=EDGE_CURVE('',#5572,#5574,#2624,.T.);
#7140=EDGE_CURVE('',#5573,#5575,#2625,.T.);
#7141=EDGE_CURVE('',#5575,#5574,#3463,.T.);
#7142=EDGE_CURVE('',#5574,#5576,#3464,.T.);
#7143=EDGE_CURVE('',#5575,#5577,#3465,.T.);
#7144=EDGE_CURVE('',#5577,#5576,#3466,.T.);
#7145=EDGE_CURVE('',#5576,#5578,#2626,.T.);
#7146=EDGE_CURVE('',#5577,#5579,#2627,.T.);
#7147=EDGE_CURVE('',#5579,#5578,#3467,.T.);
#7148=EDGE_CURVE('',#5578,#5580,#3468,.T.);
#7149=EDGE_CURVE('',#5579,#5581,#3469,.T.);
#7150=EDGE_CURVE('',#5581,#5580,#3470,.T.);
#7151=EDGE_CURVE('',#5580,#5582,#2628,.T.);
#7152=EDGE_CURVE('',#5581,#5583,#2629,.T.);
#7153=EDGE_CURVE('',#5583,#5582,#3471,.T.);
#7154=EDGE_CURVE('',#5582,#5584,#3472,.T.);
#7155=EDGE_CURVE('',#5583,#5585,#3473,.T.);
#7156=EDGE_CURVE('',#5585,#5584,#3474,.T.);
#7157=EDGE_CURVE('',#5584,#5568,#3475,.T.);
#7158=EDGE_CURVE('',#5585,#5570,#3476,.T.);
#7159=EDGE_CURVE('',#5586,#5587,#3477,.T.);
#7160=EDGE_CURVE('',#5588,#5586,#3478,.T.);
#7161=EDGE_CURVE('',#5588,#5589,#3479,.T.);
#7162=EDGE_CURVE('',#5589,#5587,#3480,.T.);
#7163=EDGE_CURVE('',#5587,#5590,#3481,.T.);
#7164=EDGE_CURVE('',#5589,#5591,#3482,.T.);
#7165=EDGE_CURVE('',#5591,#5590,#3483,.T.);
#7166=EDGE_CURVE('',#5590,#5592,#2630,.T.);
#7167=EDGE_CURVE('',#5591,#5593,#2631,.T.);
#7168=EDGE_CURVE('',#5593,#5592,#3484,.T.);
#7169=EDGE_CURVE('',#5592,#5594,#3485,.T.);
#7170=EDGE_CURVE('',#5593,#5595,#3486,.T.);
#7171=EDGE_CURVE('',#5595,#5594,#3487,.T.);
#7172=EDGE_CURVE('',#5594,#5596,#2632,.T.);
#7173=EDGE_CURVE('',#5595,#5597,#2633,.T.);
#7174=EDGE_CURVE('',#5597,#5596,#3488,.T.);
#7175=EDGE_CURVE('',#5596,#5598,#3489,.T.);
#7176=EDGE_CURVE('',#5597,#5599,#3490,.T.);
#7177=EDGE_CURVE('',#5599,#5598,#3491,.T.);
#7178=EDGE_CURVE('',#5598,#5600,#2634,.T.);
#7179=EDGE_CURVE('',#5599,#5601,#2635,.T.);
#7180=EDGE_CURVE('',#5601,#5600,#3492,.T.);
#7181=EDGE_CURVE('',#5600,#5602,#3493,.T.);
#7182=EDGE_CURVE('',#5601,#5603,#3494,.T.);
#7183=EDGE_CURVE('',#5603,#5602,#3495,.T.);
#7184=EDGE_CURVE('',#5602,#5586,#3496,.T.);
#7185=EDGE_CURVE('',#5603,#5588,#3497,.T.);
#7186=EDGE_CURVE('',#5604,#5605,#3498,.T.);
#7187=EDGE_CURVE('',#5605,#5606,#3499,.T.);
#7188=EDGE_CURVE('',#5606,#5607,#2636,.T.);
#7189=EDGE_CURVE('',#5607,#5608,#3500,.T.);
#7190=EDGE_CURVE('',#5608,#5609,#2637,.T.);
#7191=EDGE_CURVE('',#5609,#5610,#3501,.T.);
#7192=EDGE_CURVE('',#5610,#5611,#2638,.T.);
#7193=EDGE_CURVE('',#5611,#5612,#3502,.T.);
#7194=EDGE_CURVE('',#5612,#5604,#3503,.T.);
#7195=EDGE_CURVE('',#5612,#5613,#3504,.T.);
#7196=EDGE_CURVE('',#5613,#5614,#3505,.T.);
#7197=EDGE_CURVE('',#5604,#5614,#3506,.T.);
#7198=EDGE_CURVE('',#5611,#5615,#3507,.T.);
#7199=EDGE_CURVE('',#5615,#5613,#3508,.T.);
#7200=EDGE_CURVE('',#5610,#5616,#3509,.T.);
#7201=EDGE_CURVE('',#5616,#5615,#173,.T.);
#7202=EDGE_CURVE('',#5609,#5617,#3510,.T.);
#7203=EDGE_CURVE('',#5617,#5616,#3511,.T.);
#7204=EDGE_CURVE('',#5608,#5618,#3512,.T.);
#7205=EDGE_CURVE('',#5618,#5617,#174,.T.);
#7206=EDGE_CURVE('',#5607,#5619,#3513,.T.);
#7207=EDGE_CURVE('',#5619,#5618,#3514,.T.);
#7208=EDGE_CURVE('',#5606,#5620,#3515,.T.);
#7209=EDGE_CURVE('',#5620,#5619,#175,.T.);
#7210=EDGE_CURVE('',#5605,#5621,#3516,.T.);
#7211=EDGE_CURVE('',#5621,#5620,#3517,.T.);
#7212=EDGE_CURVE('',#5614,#5621,#3518,.T.);
#7213=EDGE_CURVE('',#5622,#5623,#3519,.T.);
#7214=EDGE_CURVE('',#5624,#5622,#3520,.T.);
#7215=EDGE_CURVE('',#5625,#5624,#3521,.T.);
#7216=EDGE_CURVE('',#5625,#5623,#3522,.T.);
#7217=EDGE_CURVE('',#5626,#5622,#3523,.T.);
#7218=EDGE_CURVE('',#5627,#5626,#3524,.T.);
#7219=EDGE_CURVE('',#5624,#5627,#3525,.T.);
#7220=EDGE_CURVE('',#5628,#5626,#176,.T.);
#7221=EDGE_CURVE('',#5629,#5628,#3526,.T.);
#7222=EDGE_CURVE('',#5627,#5629,#177,.T.);
#7223=EDGE_CURVE('',#5630,#5628,#3527,.T.);
#7224=EDGE_CURVE('',#5631,#5630,#3528,.T.);
#7225=EDGE_CURVE('',#5629,#5631,#3529,.T.);
#7226=EDGE_CURVE('',#5632,#5630,#178,.T.);
#7227=EDGE_CURVE('',#5633,#5632,#3530,.T.);
#7228=EDGE_CURVE('',#5631,#5633,#179,.T.);
#7229=EDGE_CURVE('',#5634,#5632,#3531,.T.);
#7230=EDGE_CURVE('',#5635,#5634,#3532,.T.);
#7231=EDGE_CURVE('',#5633,#5635,#3533,.T.);
#7232=EDGE_CURVE('',#5636,#5634,#180,.T.);
#7233=EDGE_CURVE('',#5637,#5636,#3534,.T.);
#7234=EDGE_CURVE('',#5635,#5637,#181,.T.);
#7235=EDGE_CURVE('',#5638,#5636,#3535,.T.);
#7236=EDGE_CURVE('',#5639,#5638,#3536,.T.);
#7237=EDGE_CURVE('',#5637,#5639,#3537,.T.);
#7238=EDGE_CURVE('',#5623,#5638,#3538,.T.);
#7239=EDGE_CURVE('',#5639,#5625,#3539,.T.);
#7240=EDGE_CURVE('',#5640,#5641,#3540,.T.);
#7241=EDGE_CURVE('',#5642,#5640,#3541,.T.);
#7242=EDGE_CURVE('',#5643,#5642,#3542,.T.);
#7243=EDGE_CURVE('',#5644,#5643,#2639,.T.);
#7244=EDGE_CURVE('',#5645,#5644,#3543,.T.);
#7245=EDGE_CURVE('',#5646,#5645,#2640,.T.);
#7246=EDGE_CURVE('',#5647,#5646,#3544,.T.);
#7247=EDGE_CURVE('',#5648,#5647,#2641,.T.);
#7248=EDGE_CURVE('',#5641,#5648,#3545,.T.);
#7249=EDGE_CURVE('',#5649,#5640,#3546,.T.);
#7250=EDGE_CURVE('',#5649,#5650,#3547,.T.);
#7251=EDGE_CURVE('',#5650,#5642,#3548,.T.);
#7252=EDGE_CURVE('',#5650,#5651,#3549,.T.);
#7253=EDGE_CURVE('',#5651,#5643,#3550,.T.);
#7254=EDGE_CURVE('',#5651,#5652,#182,.T.);
#7255=EDGE_CURVE('',#5652,#5644,#3551,.T.);
#7256=EDGE_CURVE('',#5652,#5653,#3552,.T.);
#7257=EDGE_CURVE('',#5653,#5645,#3553,.T.);
#7258=EDGE_CURVE('',#5653,#5654,#183,.T.);
#7259=EDGE_CURVE('',#5654,#5646,#3554,.T.);
#7260=EDGE_CURVE('',#5654,#5655,#3555,.T.);
#7261=EDGE_CURVE('',#5655,#5647,#3556,.T.);
#7262=EDGE_CURVE('',#5655,#5656,#184,.T.);
#7263=EDGE_CURVE('',#5656,#5648,#3557,.T.);
#7264=EDGE_CURVE('',#5656,#5657,#3558,.T.);
#7265=EDGE_CURVE('',#5657,#5641,#3559,.T.);
#7266=EDGE_CURVE('',#5657,#5649,#3560,.T.);
#7267=EDGE_CURVE('',#5658,#5659,#3561,.T.);
#7268=EDGE_CURVE('',#5660,#5658,#3562,.T.);
#7269=EDGE_CURVE('',#5661,#5660,#3563,.T.);
#7270=EDGE_CURVE('',#5662,#5661,#2642,.T.);
#7271=EDGE_CURVE('',#5663,#5662,#3564,.T.);
#7272=EDGE_CURVE('',#5664,#5663,#2643,.T.);
#7273=EDGE_CURVE('',#5665,#5664,#3565,.T.);
#7274=EDGE_CURVE('',#5666,#5665,#2644,.T.);
#7275=EDGE_CURVE('',#5659,#5666,#3566,.T.);
#7276=EDGE_CURVE('',#5667,#5658,#3567,.T.);
#7277=EDGE_CURVE('',#5667,#5668,#3568,.T.);
#7278=EDGE_CURVE('',#5668,#5660,#3569,.T.);
#7279=EDGE_CURVE('',#5668,#5669,#3570,.T.);
#7280=EDGE_CURVE('',#5669,#5661,#3571,.T.);
#7281=EDGE_CURVE('',#5669,#5670,#185,.T.);
#7282=EDGE_CURVE('',#5670,#5662,#3572,.T.);
#7283=EDGE_CURVE('',#5670,#5671,#3573,.T.);
#7284=EDGE_CURVE('',#5671,#5663,#3574,.T.);
#7285=EDGE_CURVE('',#5671,#5672,#186,.T.);
#7286=EDGE_CURVE('',#5672,#5664,#3575,.T.);
#7287=EDGE_CURVE('',#5672,#5673,#3576,.T.);
#7288=EDGE_CURVE('',#5673,#5665,#3577,.T.);
#7289=EDGE_CURVE('',#5673,#5674,#187,.T.);
#7290=EDGE_CURVE('',#5674,#5666,#3578,.T.);
#7291=EDGE_CURVE('',#5674,#5675,#3579,.T.);
#7292=EDGE_CURVE('',#5675,#5659,#3580,.T.);
#7293=EDGE_CURVE('',#5675,#5667,#3581,.T.);
#7294=EDGE_CURVE('',#5676,#5677,#3582,.T.);
#7295=EDGE_CURVE('',#5676,#5678,#3583,.T.);
#7296=EDGE_CURVE('',#5679,#5678,#3584,.T.);
#7297=EDGE_CURVE('',#5677,#5679,#3585,.T.);
#7298=EDGE_CURVE('',#5677,#5680,#3586,.T.);
#7299=EDGE_CURVE('',#5681,#5679,#3587,.T.);
#7300=EDGE_CURVE('',#5680,#5681,#3588,.T.);
#7301=EDGE_CURVE('',#5680,#5682,#188,.T.);
#7302=EDGE_CURVE('',#5683,#5681,#189,.T.);
#7303=EDGE_CURVE('',#5682,#5683,#3589,.T.);
#7304=EDGE_CURVE('',#5682,#5684,#3590,.T.);
#7305=EDGE_CURVE('',#5685,#5683,#3591,.T.);
#7306=EDGE_CURVE('',#5684,#5685,#3592,.T.);
#7307=EDGE_CURVE('',#5684,#5686,#190,.T.);
#7308=EDGE_CURVE('',#5687,#5685,#191,.T.);
#7309=EDGE_CURVE('',#5686,#5687,#3593,.T.);
#7310=EDGE_CURVE('',#5686,#5688,#3594,.T.);
#7311=EDGE_CURVE('',#5689,#5687,#3595,.T.);
#7312=EDGE_CURVE('',#5688,#5689,#3596,.T.);
#7313=EDGE_CURVE('',#5688,#5690,#192,.T.);
#7314=EDGE_CURVE('',#5691,#5689,#193,.T.);
#7315=EDGE_CURVE('',#5690,#5691,#3597,.T.);
#7316=EDGE_CURVE('',#5690,#5692,#3598,.T.);
#7317=EDGE_CURVE('',#5693,#5691,#3599,.T.);
#7318=EDGE_CURVE('',#5692,#5693,#3600,.T.);
#7319=EDGE_CURVE('',#5692,#5676,#3601,.T.);
#7320=EDGE_CURVE('',#5678,#5693,#3602,.T.);
#7321=EDGE_CURVE('',#5694,#5695,#3603,.T.);
#7322=EDGE_CURVE('',#5695,#5696,#3604,.T.);
#7323=EDGE_CURVE('',#5696,#5697,#2645,.T.);
#7324=EDGE_CURVE('',#5697,#5698,#3605,.T.);
#7325=EDGE_CURVE('',#5698,#5699,#2646,.T.);
#7326=EDGE_CURVE('',#5699,#5700,#3606,.T.);
#7327=EDGE_CURVE('',#5700,#5701,#2647,.T.);
#7328=EDGE_CURVE('',#5701,#5702,#3607,.T.);
#7329=EDGE_CURVE('',#5702,#5694,#3608,.T.);
#7330=EDGE_CURVE('',#5702,#5703,#3609,.T.);
#7331=EDGE_CURVE('',#5703,#5704,#3610,.T.);
#7332=EDGE_CURVE('',#5694,#5704,#3611,.T.);
#7333=EDGE_CURVE('',#5701,#5705,#3612,.T.);
#7334=EDGE_CURVE('',#5705,#5703,#3613,.T.);
#7335=EDGE_CURVE('',#5700,#5706,#3614,.T.);
#7336=EDGE_CURVE('',#5706,#5705,#194,.T.);
#7337=EDGE_CURVE('',#5699,#5707,#3615,.T.);
#7338=EDGE_CURVE('',#5707,#5706,#3616,.T.);
#7339=EDGE_CURVE('',#5698,#5708,#3617,.T.);
#7340=EDGE_CURVE('',#5708,#5707,#195,.T.);
#7341=EDGE_CURVE('',#5697,#5709,#3618,.T.);
#7342=EDGE_CURVE('',#5709,#5708,#3619,.T.);
#7343=EDGE_CURVE('',#5696,#5710,#3620,.T.);
#7344=EDGE_CURVE('',#5710,#5709,#196,.T.);
#7345=EDGE_CURVE('',#5695,#5711,#3621,.T.);
#7346=EDGE_CURVE('',#5711,#5710,#3622,.T.);
#7347=EDGE_CURVE('',#5704,#5711,#3623,.T.);
#7348=EDGE_CURVE('',#5712,#5713,#2648,.T.);
#7349=EDGE_CURVE('',#5712,#5714,#3624,.T.);
#7350=EDGE_CURVE('',#5714,#5715,#2649,.T.);
#7351=EDGE_CURVE('',#5713,#5715,#3625,.T.);
#7352=EDGE_CURVE('',#5716,#5717,#2650,.T.);
#7353=EDGE_CURVE('',#5716,#5718,#3626,.T.);
#7354=EDGE_CURVE('',#5718,#5719,#2651,.T.);
#7355=EDGE_CURVE('',#5717,#5719,#3627,.T.);
#7356=EDGE_CURVE('',#5720,#5721,#2652,.T.);
#7357=EDGE_CURVE('',#5720,#5722,#3628,.T.);
#7358=EDGE_CURVE('',#5722,#5723,#2653,.T.);
#7359=EDGE_CURVE('',#5721,#5723,#3629,.T.);
#7360=EDGE_CURVE('',#5724,#5725,#2654,.T.);
#7361=EDGE_CURVE('',#5724,#5726,#3630,.T.);
#7362=EDGE_CURVE('',#5726,#5727,#2655,.T.);
#7363=EDGE_CURVE('',#5725,#5727,#3631,.T.);
#7364=EDGE_CURVE('',#5728,#5729,#3632,.T.);
#7365=EDGE_CURVE('',#5729,#5730,#3633,.T.);
#7366=EDGE_CURVE('',#5731,#5730,#3634,.T.);
#7367=EDGE_CURVE('',#5731,#5728,#3635,.T.);
#7368=EDGE_CURVE('',#5732,#5733,#3636,.T.);
#7369=EDGE_CURVE('',#5732,#5734,#3637,.T.);
#7370=EDGE_CURVE('',#5734,#5735,#3638,.T.);
#7371=EDGE_CURVE('',#5735,#5733,#3639,.T.);
#7372=EDGE_CURVE('',#5736,#5737,#3640,.T.);
#7373=EDGE_CURVE('',#5737,#5738,#3641,.T.);
#7374=EDGE_CURVE('',#5739,#5738,#3642,.T.);
#7375=EDGE_CURVE('',#5739,#5736,#3643,.T.);
#7376=EDGE_CURVE('',#5740,#5741,#3644,.T.);
#7377=EDGE_CURVE('',#5741,#5742,#3645,.T.);
#7378=EDGE_CURVE('',#5743,#5742,#3646,.T.);
#7379=EDGE_CURVE('',#5743,#5740,#3647,.T.);
#7380=EDGE_CURVE('',#5730,#5732,#3648,.T.);
#7381=EDGE_CURVE('',#5733,#5739,#3649,.T.);
#7382=EDGE_CURVE('',#5738,#5743,#3650,.T.);
#7383=EDGE_CURVE('',#5742,#5731,#3651,.T.);
#7384=EDGE_CURVE('',#5715,#5744,#3652,.T.);
#7385=EDGE_CURVE('',#5745,#5714,#3653,.T.);
#7386=EDGE_CURVE('',#5744,#5745,#2656,.T.);
#7387=EDGE_CURVE('',#5719,#5746,#3654,.T.);
#7388=EDGE_CURVE('',#5747,#5718,#3655,.T.);
#7389=EDGE_CURVE('',#5746,#5747,#2657,.T.);
#7390=EDGE_CURVE('',#5723,#5748,#3656,.T.);
#7391=EDGE_CURVE('',#5749,#5722,#3657,.T.);
#7392=EDGE_CURVE('',#5748,#5749,#2658,.T.);
#7393=EDGE_CURVE('',#5727,#5750,#3658,.T.);
#7394=EDGE_CURVE('',#5751,#5726,#3659,.T.);
#7395=EDGE_CURVE('',#5750,#5751,#2659,.T.);
#7396=EDGE_CURVE('',#5734,#5729,#3660,.T.);
#7397=EDGE_CURVE('',#5728,#5741,#3661,.T.);
#7398=EDGE_CURVE('',#5740,#5737,#3662,.T.);
#7399=EDGE_CURVE('',#5736,#5735,#3663,.T.);
#7400=EDGE_CURVE('',#5713,#5752,#3664,.T.);
#7401=EDGE_CURVE('',#5752,#5753,#2660,.T.);
#7402=EDGE_CURVE('',#5753,#5712,#3665,.T.);
#7403=EDGE_CURVE('',#5717,#5754,#3666,.T.);
#7404=EDGE_CURVE('',#5754,#5755,#2661,.T.);
#7405=EDGE_CURVE('',#5755,#5716,#3667,.T.);
#7406=EDGE_CURVE('',#5721,#5756,#3668,.T.);
#7407=EDGE_CURVE('',#5756,#5757,#2662,.T.);
#7408=EDGE_CURVE('',#5757,#5720,#3669,.T.);
#7409=EDGE_CURVE('',#5725,#5758,#3670,.T.);
#7410=EDGE_CURVE('',#5758,#5759,#2663,.T.);
#7411=EDGE_CURVE('',#5759,#5724,#3671,.T.);
#7412=EDGE_CURVE('',#5759,#5751,#3672,.T.);
#7413=EDGE_CURVE('',#5758,#5750,#3673,.T.);
#7414=EDGE_CURVE('',#5757,#5749,#3674,.T.);
#7415=EDGE_CURVE('',#5756,#5748,#3675,.T.);
#7416=EDGE_CURVE('',#5755,#5747,#3676,.T.);
#7417=EDGE_CURVE('',#5754,#5746,#3677,.T.);
#7418=EDGE_CURVE('',#5753,#5745,#3678,.T.);
#7419=EDGE_CURVE('',#5752,#5744,#3679,.T.);
#7420=EDGE_CURVE('',#5760,#5760,#2664,.T.);
#7421=EDGE_CURVE('',#5760,#5761,#3680,.T.);
#7422=EDGE_CURVE('',#5761,#5761,#2665,.T.);
#7423=EDGE_CURVE('',#5762,#5762,#2666,.T.);
#7424=EDGE_CURVE('',#5762,#5763,#3681,.T.);
#7425=EDGE_CURVE('',#5763,#5763,#2667,.T.);
#7426=EDGE_CURVE('',#5764,#5765,#3682,.T.);
#7427=EDGE_CURVE('',#5766,#5764,#3683,.T.);
#7428=EDGE_CURVE('',#5767,#5766,#3684,.T.);
#7429=EDGE_CURVE('',#5767,#5765,#3685,.T.);
#7430=EDGE_CURVE('',#5768,#5764,#3686,.T.);
#7431=EDGE_CURVE('',#5769,#5768,#3687,.T.);
#7432=EDGE_CURVE('',#5766,#5769,#3688,.T.);
#7433=EDGE_CURVE('',#5770,#5768,#197,.T.);
#7434=EDGE_CURVE('',#5771,#5770,#3689,.T.);
#7435=EDGE_CURVE('',#5769,#5771,#198,.T.);
#7436=EDGE_CURVE('',#5772,#5770,#3690,.T.);
#7437=EDGE_CURVE('',#5773,#5772,#3691,.T.);
#7438=EDGE_CURVE('',#5771,#5773,#3692,.T.);
#7439=EDGE_CURVE('',#5774,#5772,#199,.T.);
#7440=EDGE_CURVE('',#5775,#5774,#3693,.T.);
#7441=EDGE_CURVE('',#5773,#5775,#200,.T.);
#7442=EDGE_CURVE('',#5776,#5774,#3694,.T.);
#7443=EDGE_CURVE('',#5777,#5776,#3695,.T.);
#7444=EDGE_CURVE('',#5775,#5777,#3696,.T.);
#7445=EDGE_CURVE('',#5778,#5776,#201,.T.);
#7446=EDGE_CURVE('',#5779,#5778,#3697,.T.);
#7447=EDGE_CURVE('',#5777,#5779,#202,.T.);
#7448=EDGE_CURVE('',#5780,#5778,#3698,.T.);
#7449=EDGE_CURVE('',#5781,#5780,#3699,.T.);
#7450=EDGE_CURVE('',#5779,#5781,#3700,.T.);
#7451=EDGE_CURVE('',#5782,#5780,#203,.T.);
#7452=EDGE_CURVE('',#5783,#5782,#3701,.T.);
#7453=EDGE_CURVE('',#5781,#5783,#204,.T.);
#7454=EDGE_CURVE('',#5784,#5782,#3702,.T.);
#7455=EDGE_CURVE('',#5785,#5784,#3703,.T.);
#7456=EDGE_CURVE('',#5783,#5785,#3704,.T.);
#7457=EDGE_CURVE('',#5786,#5784,#3705,.T.);
#7458=EDGE_CURVE('',#5787,#5786,#3706,.T.);
#7459=EDGE_CURVE('',#5785,#5787,#3707,.T.);
#7460=EDGE_CURVE('',#5765,#5786,#3708,.T.);
#7461=EDGE_CURVE('',#5787,#5767,#3709,.T.);
#7462=EDGE_CURVE('',#5788,#5788,#2668,.T.);
#7463=EDGE_CURVE('',#5788,#5789,#3710,.T.);
#7464=EDGE_CURVE('',#5789,#5789,#2669,.T.);
#7465=EDGE_CURVE('',#5790,#5790,#2670,.T.);
#7466=EDGE_CURVE('',#5790,#5791,#3711,.T.);
#7467=EDGE_CURVE('',#5791,#5791,#2671,.T.);
#7468=EDGE_CURVE('',#5792,#5793,#3712,.T.);
#7469=EDGE_CURVE('',#5794,#5793,#3713,.T.);
#7470=EDGE_CURVE('',#5795,#5794,#3714,.T.);
#7471=EDGE_CURVE('',#5795,#5792,#3715,.T.);
#7472=EDGE_CURVE('',#5793,#5796,#3716,.T.);
#7473=EDGE_CURVE('',#5797,#5796,#3717,.T.);
#7474=EDGE_CURVE('',#5794,#5797,#3718,.T.);
#7475=EDGE_CURVE('',#5796,#5798,#2672,.T.);
#7476=EDGE_CURVE('',#5799,#5798,#3719,.T.);
#7477=EDGE_CURVE('',#5797,#5799,#2673,.T.);
#7478=EDGE_CURVE('',#5798,#5800,#3720,.T.);
#7479=EDGE_CURVE('',#5801,#5800,#3721,.T.);
#7480=EDGE_CURVE('',#5799,#5801,#3722,.T.);
#7481=EDGE_CURVE('',#5800,#5802,#2674,.T.);
#7482=EDGE_CURVE('',#5803,#5802,#3723,.T.);
#7483=EDGE_CURVE('',#5801,#5803,#2675,.T.);
#7484=EDGE_CURVE('',#5802,#5804,#3724,.T.);
#7485=EDGE_CURVE('',#5805,#5804,#3725,.T.);
#7486=EDGE_CURVE('',#5803,#5805,#3726,.T.);
#7487=EDGE_CURVE('',#5804,#5806,#2676,.T.);
#7488=EDGE_CURVE('',#5807,#5806,#3727,.T.);
#7489=EDGE_CURVE('',#5805,#5807,#2677,.T.);
#7490=EDGE_CURVE('',#5806,#5808,#3728,.T.);
#7491=EDGE_CURVE('',#5809,#5808,#3729,.T.);
#7492=EDGE_CURVE('',#5807,#5809,#3730,.T.);
#7493=EDGE_CURVE('',#5808,#5792,#3731,.T.);
#7494=EDGE_CURVE('',#5809,#5795,#3732,.T.);
#7495=EDGE_CURVE('',#5810,#5810,#2678,.T.);
#7496=EDGE_CURVE('',#5810,#5811,#3733,.T.);
#7497=EDGE_CURVE('',#5811,#5811,#2679,.T.);
#7498=EDGE_CURVE('',#5812,#5812,#2680,.T.);
#7499=EDGE_CURVE('',#5812,#5813,#3734,.T.);
#7500=EDGE_CURVE('',#5813,#5813,#2681,.T.);
#7501=EDGE_CURVE('',#5814,#5815,#3735,.T.);
#7502=EDGE_CURVE('',#5816,#5814,#3736,.T.);
#7503=EDGE_CURVE('',#5816,#5817,#3737,.T.);
#7504=EDGE_CURVE('',#5817,#5815,#3738,.T.);
#7505=EDGE_CURVE('',#5815,#5818,#3739,.T.);
#7506=EDGE_CURVE('',#5817,#5819,#3740,.T.);
#7507=EDGE_CURVE('',#5819,#5818,#3741,.T.);
#7508=EDGE_CURVE('',#5818,#5820,#2682,.T.);
#7509=EDGE_CURVE('',#5819,#5821,#2683,.T.);
#7510=EDGE_CURVE('',#5821,#5820,#3742,.T.);
#7511=EDGE_CURVE('',#5820,#5822,#3743,.T.);
#7512=EDGE_CURVE('',#5821,#5823,#3744,.T.);
#7513=EDGE_CURVE('',#5823,#5822,#3745,.T.);
#7514=EDGE_CURVE('',#5822,#5824,#2684,.T.);
#7515=EDGE_CURVE('',#5823,#5825,#2685,.T.);
#7516=EDGE_CURVE('',#5825,#5824,#3746,.T.);
#7517=EDGE_CURVE('',#5824,#5826,#3747,.T.);
#7518=EDGE_CURVE('',#5825,#5827,#3748,.T.);
#7519=EDGE_CURVE('',#5827,#5826,#3749,.T.);
#7520=EDGE_CURVE('',#5826,#5828,#2686,.T.);
#7521=EDGE_CURVE('',#5827,#5829,#2687,.T.);
#7522=EDGE_CURVE('',#5829,#5828,#3750,.T.);
#7523=EDGE_CURVE('',#5828,#5830,#3751,.T.);
#7524=EDGE_CURVE('',#5829,#5831,#3752,.T.);
#7525=EDGE_CURVE('',#5831,#5830,#3753,.T.);
#7526=EDGE_CURVE('',#5830,#5814,#3754,.T.);
#7527=EDGE_CURVE('',#5831,#5816,#3755,.T.);
#9300=ORIENTED_EDGE('',*,*,#6718,.F.);
#9301=ORIENTED_EDGE('',*,*,#6719,.F.);
#9302=ORIENTED_EDGE('',*,*,#6720,.F.);
#9303=ORIENTED_EDGE('',*,*,#6721,.T.);
#9304=ORIENTED_EDGE('',*,*,#6722,.F.);
#9305=ORIENTED_EDGE('',*,*,#6723,.F.);
#9306=ORIENTED_EDGE('',*,*,#6724,.F.);
#9307=ORIENTED_EDGE('',*,*,#6719,.T.);
#9308=ORIENTED_EDGE('',*,*,#6725,.F.);
#9309=ORIENTED_EDGE('',*,*,#6726,.F.);
#9310=ORIENTED_EDGE('',*,*,#6727,.F.);
#9311=ORIENTED_EDGE('',*,*,#6723,.T.);
#9312=ORIENTED_EDGE('',*,*,#6728,.F.);
#9313=ORIENTED_EDGE('',*,*,#6729,.F.);
#9314=ORIENTED_EDGE('',*,*,#6730,.F.);
#9315=ORIENTED_EDGE('',*,*,#6726,.T.);
#9316=ORIENTED_EDGE('',*,*,#6731,.F.);
#9317=ORIENTED_EDGE('',*,*,#6732,.F.);
#9318=ORIENTED_EDGE('',*,*,#6733,.F.);
#9319=ORIENTED_EDGE('',*,*,#6729,.T.);
#9320=ORIENTED_EDGE('',*,*,#6734,.F.);
#9321=ORIENTED_EDGE('',*,*,#6735,.F.);
#9322=ORIENTED_EDGE('',*,*,#6736,.F.);
#9323=ORIENTED_EDGE('',*,*,#6732,.T.);
#9324=ORIENTED_EDGE('',*,*,#6737,.F.);
#9325=ORIENTED_EDGE('',*,*,#6738,.F.);
#9326=ORIENTED_EDGE('',*,*,#6739,.F.);
#9327=ORIENTED_EDGE('',*,*,#6735,.T.);
#9328=ORIENTED_EDGE('',*,*,#6740,.F.);
#9329=ORIENTED_EDGE('',*,*,#6741,.F.);
#9330=ORIENTED_EDGE('',*,*,#6742,.F.);
#9331=ORIENTED_EDGE('',*,*,#6738,.T.);
#9332=ORIENTED_EDGE('',*,*,#6743,.F.);
#9333=ORIENTED_EDGE('',*,*,#6744,.F.);
#9334=ORIENTED_EDGE('',*,*,#6745,.F.);
#9335=ORIENTED_EDGE('',*,*,#6741,.T.);
#9336=ORIENTED_EDGE('',*,*,#6746,.F.);
#9337=ORIENTED_EDGE('',*,*,#6747,.F.);
#9338=ORIENTED_EDGE('',*,*,#6748,.F.);
#9339=ORIENTED_EDGE('',*,*,#6744,.T.);
#9340=ORIENTED_EDGE('',*,*,#6749,.F.);
#9341=ORIENTED_EDGE('',*,*,#6750,.F.);
#9342=ORIENTED_EDGE('',*,*,#6751,.F.);
#9343=ORIENTED_EDGE('',*,*,#6747,.T.);
#9344=ORIENTED_EDGE('',*,*,#6752,.F.);
#9345=ORIENTED_EDGE('',*,*,#6721,.F.);
#9346=ORIENTED_EDGE('',*,*,#6753,.F.);
#9347=ORIENTED_EDGE('',*,*,#6750,.T.);
#9348=ORIENTED_EDGE('',*,*,#6753,.T.);
#9349=ORIENTED_EDGE('',*,*,#6720,.T.);
#9350=ORIENTED_EDGE('',*,*,#6724,.T.);
#9351=ORIENTED_EDGE('',*,*,#6727,.T.);
#9352=ORIENTED_EDGE('',*,*,#6730,.T.);
#9353=ORIENTED_EDGE('',*,*,#6733,.T.);
#9354=ORIENTED_EDGE('',*,*,#6736,.T.);
#9355=ORIENTED_EDGE('',*,*,#6739,.T.);
#9356=ORIENTED_EDGE('',*,*,#6742,.T.);
#9357=ORIENTED_EDGE('',*,*,#6745,.T.);
#9358=ORIENTED_EDGE('',*,*,#6748,.T.);
#9359=ORIENTED_EDGE('',*,*,#6751,.T.);
#9360=ORIENTED_EDGE('',*,*,#6722,.T.);
#9361=ORIENTED_EDGE('',*,*,#6718,.T.);
#9362=ORIENTED_EDGE('',*,*,#6752,.T.);
#9363=ORIENTED_EDGE('',*,*,#6749,.T.);
#9364=ORIENTED_EDGE('',*,*,#6746,.T.);
#9365=ORIENTED_EDGE('',*,*,#6743,.T.);
#9366=ORIENTED_EDGE('',*,*,#6740,.T.);
#9367=ORIENTED_EDGE('',*,*,#6737,.T.);
#9368=ORIENTED_EDGE('',*,*,#6734,.T.);
#9369=ORIENTED_EDGE('',*,*,#6731,.T.);
#9370=ORIENTED_EDGE('',*,*,#6728,.T.);
#9371=ORIENTED_EDGE('',*,*,#6725,.T.);
#9372=ORIENTED_EDGE('',*,*,#6754,.T.);
#9373=ORIENTED_EDGE('',*,*,#6755,.T.);
#9374=ORIENTED_EDGE('',*,*,#6756,.T.);
#9375=ORIENTED_EDGE('',*,*,#6757,.T.);
#9376=ORIENTED_EDGE('',*,*,#6758,.T.);
#9377=ORIENTED_EDGE('',*,*,#6759,.T.);
#9378=ORIENTED_EDGE('',*,*,#6760,.T.);
#9379=ORIENTED_EDGE('',*,*,#6761,.T.);
#9380=ORIENTED_EDGE('',*,*,#6762,.T.);
#9381=ORIENTED_EDGE('',*,*,#6763,.F.);
#9382=ORIENTED_EDGE('',*,*,#6764,.T.);
#9383=ORIENTED_EDGE('',*,*,#6765,.T.);
#9384=ORIENTED_EDGE('',*,*,#6766,.T.);
#9385=ORIENTED_EDGE('',*,*,#6767,.T.);
#9386=ORIENTED_EDGE('',*,*,#6768,.F.);
#9387=ORIENTED_EDGE('',*,*,#6764,.F.);
#9388=ORIENTED_EDGE('',*,*,#6769,.T.);
#9389=ORIENTED_EDGE('',*,*,#6770,.T.);
#9390=ORIENTED_EDGE('',*,*,#6766,.F.);
#9391=ORIENTED_EDGE('',*,*,#6763,.T.);
#9392=ORIENTED_EDGE('',*,*,#6771,.T.);
#9393=ORIENTED_EDGE('',*,*,#6772,.T.);
#9394=ORIENTED_EDGE('',*,*,#6769,.F.);
#9395=ORIENTED_EDGE('',*,*,#6762,.F.);
#9396=ORIENTED_EDGE('',*,*,#6773,.T.);
#9397=ORIENTED_EDGE('',*,*,#6774,.T.);
#9398=ORIENTED_EDGE('',*,*,#6771,.F.);
#9399=ORIENTED_EDGE('',*,*,#6761,.F.);
#9400=ORIENTED_EDGE('',*,*,#6775,.T.);
#9401=ORIENTED_EDGE('',*,*,#6776,.T.);
#9402=ORIENTED_EDGE('',*,*,#6773,.F.);
#9403=ORIENTED_EDGE('',*,*,#6760,.F.);
#9404=ORIENTED_EDGE('',*,*,#6777,.T.);
#9405=ORIENTED_EDGE('',*,*,#6778,.T.);
#9406=ORIENTED_EDGE('',*,*,#6775,.F.);
#9407=ORIENTED_EDGE('',*,*,#6759,.F.);
#9408=ORIENTED_EDGE('',*,*,#6779,.T.);
#9409=ORIENTED_EDGE('',*,*,#6780,.T.);
#9410=ORIENTED_EDGE('',*,*,#6777,.F.);
#9411=ORIENTED_EDGE('',*,*,#6758,.F.);
#9412=ORIENTED_EDGE('',*,*,#6781,.T.);
#9413=ORIENTED_EDGE('',*,*,#6782,.T.);
#9414=ORIENTED_EDGE('',*,*,#6779,.F.);
#9415=ORIENTED_EDGE('',*,*,#6757,.F.);
#9416=ORIENTED_EDGE('',*,*,#6783,.T.);
#9417=ORIENTED_EDGE('',*,*,#6784,.T.);
#9418=ORIENTED_EDGE('',*,*,#6781,.F.);
#9419=ORIENTED_EDGE('',*,*,#6756,.F.);
#9420=ORIENTED_EDGE('',*,*,#6785,.T.);
#9421=ORIENTED_EDGE('',*,*,#6786,.T.);
#9422=ORIENTED_EDGE('',*,*,#6783,.F.);
#9423=ORIENTED_EDGE('',*,*,#6755,.F.);
#9424=ORIENTED_EDGE('',*,*,#6787,.T.);
#9425=ORIENTED_EDGE('',*,*,#6788,.T.);
#9426=ORIENTED_EDGE('',*,*,#6785,.F.);
#9427=ORIENTED_EDGE('',*,*,#6754,.F.);
#9428=ORIENTED_EDGE('',*,*,#6768,.T.);
#9429=ORIENTED_EDGE('',*,*,#6789,.T.);
#9430=ORIENTED_EDGE('',*,*,#6787,.F.);
#9431=ORIENTED_EDGE('',*,*,#6765,.F.);
#9432=ORIENTED_EDGE('',*,*,#6767,.F.);
#9433=ORIENTED_EDGE('',*,*,#6770,.F.);
#9434=ORIENTED_EDGE('',*,*,#6772,.F.);
#9435=ORIENTED_EDGE('',*,*,#6774,.F.);
#9436=ORIENTED_EDGE('',*,*,#6776,.F.);
#9437=ORIENTED_EDGE('',*,*,#6778,.F.);
#9438=ORIENTED_EDGE('',*,*,#6780,.F.);
#9439=ORIENTED_EDGE('',*,*,#6782,.F.);
#9440=ORIENTED_EDGE('',*,*,#6784,.F.);
#9441=ORIENTED_EDGE('',*,*,#6786,.F.);
#9442=ORIENTED_EDGE('',*,*,#6788,.F.);
#9443=ORIENTED_EDGE('',*,*,#6789,.F.);
#9444=ORIENTED_EDGE('',*,*,#6790,.T.);
#9445=ORIENTED_EDGE('',*,*,#6791,.T.);
#9446=ORIENTED_EDGE('',*,*,#6792,.T.);
#9447=ORIENTED_EDGE('',*,*,#6793,.T.);
#9448=ORIENTED_EDGE('',*,*,#6794,.T.);
#9449=ORIENTED_EDGE('',*,*,#6795,.T.);
#9450=ORIENTED_EDGE('',*,*,#6796,.T.);
#9451=ORIENTED_EDGE('',*,*,#6797,.T.);
#9452=ORIENTED_EDGE('',*,*,#6798,.T.);
#9453=ORIENTED_EDGE('',*,*,#6799,.T.);
#9454=ORIENTED_EDGE('',*,*,#6800,.T.);
#9455=ORIENTED_EDGE('',*,*,#6801,.T.);
#9456=ORIENTED_EDGE('',*,*,#6802,.F.);
#9457=ORIENTED_EDGE('',*,*,#6803,.T.);
#9458=ORIENTED_EDGE('',*,*,#6804,.T.);
#9459=ORIENTED_EDGE('',*,*,#6792,.F.);
#9460=ORIENTED_EDGE('',*,*,#6804,.F.);
#9461=ORIENTED_EDGE('',*,*,#6805,.T.);
#9462=ORIENTED_EDGE('',*,*,#6806,.T.);
#9463=ORIENTED_EDGE('',*,*,#6793,.F.);
#9464=ORIENTED_EDGE('',*,*,#6806,.F.);
#9465=ORIENTED_EDGE('',*,*,#6807,.T.);
#9466=ORIENTED_EDGE('',*,*,#6808,.T.);
#9467=ORIENTED_EDGE('',*,*,#6794,.F.);
#9468=ORIENTED_EDGE('',*,*,#6808,.F.);
#9469=ORIENTED_EDGE('',*,*,#6809,.T.);
#9470=ORIENTED_EDGE('',*,*,#6810,.T.);
#9471=ORIENTED_EDGE('',*,*,#6795,.F.);
#9472=ORIENTED_EDGE('',*,*,#6810,.F.);
#9473=ORIENTED_EDGE('',*,*,#6811,.T.);
#9474=ORIENTED_EDGE('',*,*,#6812,.T.);
#9475=ORIENTED_EDGE('',*,*,#6796,.F.);
#9476=ORIENTED_EDGE('',*,*,#6812,.F.);
#9477=ORIENTED_EDGE('',*,*,#6813,.T.);
#9478=ORIENTED_EDGE('',*,*,#6814,.T.);
#9479=ORIENTED_EDGE('',*,*,#6797,.F.);
#9480=ORIENTED_EDGE('',*,*,#6814,.F.);
#9481=ORIENTED_EDGE('',*,*,#6815,.T.);
#9482=ORIENTED_EDGE('',*,*,#6816,.T.);
#9483=ORIENTED_EDGE('',*,*,#6798,.F.);
#9484=ORIENTED_EDGE('',*,*,#6816,.F.);
#9485=ORIENTED_EDGE('',*,*,#6817,.T.);
#9486=ORIENTED_EDGE('',*,*,#6818,.T.);
#9487=ORIENTED_EDGE('',*,*,#6799,.F.);
#9488=ORIENTED_EDGE('',*,*,#6818,.F.);
#9489=ORIENTED_EDGE('',*,*,#6819,.T.);
#9490=ORIENTED_EDGE('',*,*,#6820,.T.);
#9491=ORIENTED_EDGE('',*,*,#6800,.F.);
#9492=ORIENTED_EDGE('',*,*,#6820,.F.);
#9493=ORIENTED_EDGE('',*,*,#6821,.T.);
#9494=ORIENTED_EDGE('',*,*,#6822,.T.);
#9495=ORIENTED_EDGE('',*,*,#6801,.F.);
#9496=ORIENTED_EDGE('',*,*,#6822,.F.);
#9497=ORIENTED_EDGE('',*,*,#6823,.T.);
#9498=ORIENTED_EDGE('',*,*,#6824,.T.);
#9499=ORIENTED_EDGE('',*,*,#6790,.F.);
#9500=ORIENTED_EDGE('',*,*,#6824,.F.);
#9501=ORIENTED_EDGE('',*,*,#6825,.T.);
#9502=ORIENTED_EDGE('',*,*,#6802,.T.);
#9503=ORIENTED_EDGE('',*,*,#6791,.F.);
#9504=ORIENTED_EDGE('',*,*,#6823,.F.);
#9505=ORIENTED_EDGE('',*,*,#6821,.F.);
#9506=ORIENTED_EDGE('',*,*,#6819,.F.);
#9507=ORIENTED_EDGE('',*,*,#6817,.F.);
#9508=ORIENTED_EDGE('',*,*,#6815,.F.);
#9509=ORIENTED_EDGE('',*,*,#6813,.F.);
#9510=ORIENTED_EDGE('',*,*,#6811,.F.);
#9511=ORIENTED_EDGE('',*,*,#6809,.F.);
#9512=ORIENTED_EDGE('',*,*,#6807,.F.);
#9513=ORIENTED_EDGE('',*,*,#6805,.F.);
#9514=ORIENTED_EDGE('',*,*,#6803,.F.);
#9515=ORIENTED_EDGE('',*,*,#6825,.F.);
#9516=ORIENTED_EDGE('',*,*,#6826,.T.);
#9517=ORIENTED_EDGE('',*,*,#6827,.T.);
#9518=ORIENTED_EDGE('',*,*,#6828,.F.);
#9519=ORIENTED_EDGE('',*,*,#6829,.F.);
#9520=ORIENTED_EDGE('',*,*,#6830,.F.);
#9521=ORIENTED_EDGE('',*,*,#6829,.T.);
#9522=ORIENTED_EDGE('',*,*,#6831,.F.);
#9523=ORIENTED_EDGE('',*,*,#6832,.F.);
#9524=ORIENTED_EDGE('',*,*,#6833,.F.);
#9525=ORIENTED_EDGE('',*,*,#6832,.T.);
#9526=ORIENTED_EDGE('',*,*,#6834,.F.);
#9527=ORIENTED_EDGE('',*,*,#6835,.F.);
#9528=ORIENTED_EDGE('',*,*,#6836,.F.);
#9529=ORIENTED_EDGE('',*,*,#6835,.T.);
#9530=ORIENTED_EDGE('',*,*,#6837,.F.);
#9531=ORIENTED_EDGE('',*,*,#6838,.F.);
#9532=ORIENTED_EDGE('',*,*,#6839,.F.);
#9533=ORIENTED_EDGE('',*,*,#6838,.T.);
#9534=ORIENTED_EDGE('',*,*,#6840,.F.);
#9535=ORIENTED_EDGE('',*,*,#6841,.F.);
#9536=ORIENTED_EDGE('',*,*,#6842,.F.);
#9537=ORIENTED_EDGE('',*,*,#6841,.T.);
#9538=ORIENTED_EDGE('',*,*,#6843,.F.);
#9539=ORIENTED_EDGE('',*,*,#6844,.F.);
#9540=ORIENTED_EDGE('',*,*,#6845,.F.);
#9541=ORIENTED_EDGE('',*,*,#6844,.T.);
#9542=ORIENTED_EDGE('',*,*,#6846,.F.);
#9543=ORIENTED_EDGE('',*,*,#6847,.F.);
#9544=ORIENTED_EDGE('',*,*,#6848,.F.);
#9545=ORIENTED_EDGE('',*,*,#6847,.T.);
#9546=ORIENTED_EDGE('',*,*,#6849,.F.);
#9547=ORIENTED_EDGE('',*,*,#6850,.F.);
#9548=ORIENTED_EDGE('',*,*,#6851,.F.);
#9549=ORIENTED_EDGE('',*,*,#6850,.T.);
#9550=ORIENTED_EDGE('',*,*,#6852,.F.);
#9551=ORIENTED_EDGE('',*,*,#6853,.F.);
#9552=ORIENTED_EDGE('',*,*,#6854,.F.);
#9553=ORIENTED_EDGE('',*,*,#6853,.T.);
#9554=ORIENTED_EDGE('',*,*,#6855,.F.);
#9555=ORIENTED_EDGE('',*,*,#6856,.F.);
#9556=ORIENTED_EDGE('',*,*,#6857,.F.);
#9557=ORIENTED_EDGE('',*,*,#6856,.T.);
#9558=ORIENTED_EDGE('',*,*,#6858,.F.);
#9559=ORIENTED_EDGE('',*,*,#6859,.F.);
#9560=ORIENTED_EDGE('',*,*,#6860,.F.);
#9561=ORIENTED_EDGE('',*,*,#6859,.T.);
#9562=ORIENTED_EDGE('',*,*,#6861,.F.);
#9563=ORIENTED_EDGE('',*,*,#6827,.F.);
#9564=ORIENTED_EDGE('',*,*,#6831,.T.);
#9565=ORIENTED_EDGE('',*,*,#6828,.T.);
#9566=ORIENTED_EDGE('',*,*,#6861,.T.);
#9567=ORIENTED_EDGE('',*,*,#6858,.T.);
#9568=ORIENTED_EDGE('',*,*,#6855,.T.);
#9569=ORIENTED_EDGE('',*,*,#6852,.T.);
#9570=ORIENTED_EDGE('',*,*,#6849,.T.);
#9571=ORIENTED_EDGE('',*,*,#6846,.T.);
#9572=ORIENTED_EDGE('',*,*,#6843,.T.);
#9573=ORIENTED_EDGE('',*,*,#6840,.T.);
#9574=ORIENTED_EDGE('',*,*,#6837,.T.);
#9575=ORIENTED_EDGE('',*,*,#6834,.T.);
#9576=ORIENTED_EDGE('',*,*,#6830,.T.);
#9577=ORIENTED_EDGE('',*,*,#6833,.T.);
#9578=ORIENTED_EDGE('',*,*,#6836,.T.);
#9579=ORIENTED_EDGE('',*,*,#6839,.T.);
#9580=ORIENTED_EDGE('',*,*,#6842,.T.);
#9581=ORIENTED_EDGE('',*,*,#6845,.T.);
#9582=ORIENTED_EDGE('',*,*,#6848,.T.);
#9583=ORIENTED_EDGE('',*,*,#6851,.T.);
#9584=ORIENTED_EDGE('',*,*,#6854,.T.);
#9585=ORIENTED_EDGE('',*,*,#6857,.T.);
#9586=ORIENTED_EDGE('',*,*,#6860,.T.);
#9587=ORIENTED_EDGE('',*,*,#6826,.F.);
#9588=ORIENTED_EDGE('',*,*,#6862,.F.);
#9589=ORIENTED_EDGE('',*,*,#6863,.F.);
#9590=ORIENTED_EDGE('',*,*,#6864,.F.);
#9591=ORIENTED_EDGE('',*,*,#6865,.T.);
#9592=ORIENTED_EDGE('',*,*,#6866,.F.);
#9593=ORIENTED_EDGE('',*,*,#6867,.F.);
#9594=ORIENTED_EDGE('',*,*,#6868,.F.);
#9595=ORIENTED_EDGE('',*,*,#6863,.T.);
#9596=ORIENTED_EDGE('',*,*,#6869,.F.);
#9597=ORIENTED_EDGE('',*,*,#6870,.F.);
#9598=ORIENTED_EDGE('',*,*,#6871,.F.);
#9599=ORIENTED_EDGE('',*,*,#6867,.T.);
#9600=ORIENTED_EDGE('',*,*,#6872,.F.);
#9601=ORIENTED_EDGE('',*,*,#6873,.F.);
#9602=ORIENTED_EDGE('',*,*,#6874,.F.);
#9603=ORIENTED_EDGE('',*,*,#6870,.T.);
#9604=ORIENTED_EDGE('',*,*,#6875,.F.);
#9605=ORIENTED_EDGE('',*,*,#6876,.F.);
#9606=ORIENTED_EDGE('',*,*,#6877,.F.);
#9607=ORIENTED_EDGE('',*,*,#6873,.T.);
#9608=ORIENTED_EDGE('',*,*,#6878,.F.);
#9609=ORIENTED_EDGE('',*,*,#6879,.F.);
#9610=ORIENTED_EDGE('',*,*,#6880,.F.);
#9611=ORIENTED_EDGE('',*,*,#6876,.T.);
#9612=ORIENTED_EDGE('',*,*,#6881,.F.);
#9613=ORIENTED_EDGE('',*,*,#6882,.F.);
#9614=ORIENTED_EDGE('',*,*,#6883,.F.);
#9615=ORIENTED_EDGE('',*,*,#6879,.T.);
#9616=ORIENTED_EDGE('',*,*,#6884,.F.);
#9617=ORIENTED_EDGE('',*,*,#6885,.F.);
#9618=ORIENTED_EDGE('',*,*,#6886,.F.);
#9619=ORIENTED_EDGE('',*,*,#6882,.T.);
#9620=ORIENTED_EDGE('',*,*,#6887,.F.);
#9621=ORIENTED_EDGE('',*,*,#6888,.F.);
#9622=ORIENTED_EDGE('',*,*,#6889,.F.);
#9623=ORIENTED_EDGE('',*,*,#6885,.T.);
#9624=ORIENTED_EDGE('',*,*,#6890,.F.);
#9625=ORIENTED_EDGE('',*,*,#6891,.F.);
#9626=ORIENTED_EDGE('',*,*,#6892,.F.);
#9627=ORIENTED_EDGE('',*,*,#6888,.T.);
#9628=ORIENTED_EDGE('',*,*,#6893,.F.);
#9629=ORIENTED_EDGE('',*,*,#6894,.F.);
#9630=ORIENTED_EDGE('',*,*,#6895,.F.);
#9631=ORIENTED_EDGE('',*,*,#6891,.T.);
#9632=ORIENTED_EDGE('',*,*,#6896,.F.);
#9633=ORIENTED_EDGE('',*,*,#6865,.F.);
#9634=ORIENTED_EDGE('',*,*,#6897,.F.);
#9635=ORIENTED_EDGE('',*,*,#6894,.T.);
#9636=ORIENTED_EDGE('',*,*,#6897,.T.);
#9637=ORIENTED_EDGE('',*,*,#6864,.T.);
#9638=ORIENTED_EDGE('',*,*,#6868,.T.);
#9639=ORIENTED_EDGE('',*,*,#6871,.T.);
#9640=ORIENTED_EDGE('',*,*,#6874,.T.);
#9641=ORIENTED_EDGE('',*,*,#6877,.T.);
#9642=ORIENTED_EDGE('',*,*,#6880,.T.);
#9643=ORIENTED_EDGE('',*,*,#6883,.T.);
#9644=ORIENTED_EDGE('',*,*,#6886,.T.);
#9645=ORIENTED_EDGE('',*,*,#6889,.T.);
#9646=ORIENTED_EDGE('',*,*,#6892,.T.);
#9647=ORIENTED_EDGE('',*,*,#6895,.T.);
#9648=ORIENTED_EDGE('',*,*,#6866,.T.);
#9649=ORIENTED_EDGE('',*,*,#6862,.T.);
#9650=ORIENTED_EDGE('',*,*,#6896,.T.);
#9651=ORIENTED_EDGE('',*,*,#6893,.T.);
#9652=ORIENTED_EDGE('',*,*,#6890,.T.);
#9653=ORIENTED_EDGE('',*,*,#6887,.T.);
#9654=ORIENTED_EDGE('',*,*,#6884,.T.);
#9655=ORIENTED_EDGE('',*,*,#6881,.T.);
#9656=ORIENTED_EDGE('',*,*,#6878,.T.);
#9657=ORIENTED_EDGE('',*,*,#6875,.T.);
#9658=ORIENTED_EDGE('',*,*,#6872,.T.);
#9659=ORIENTED_EDGE('',*,*,#6869,.T.);
#9660=ORIENTED_EDGE('',*,*,#6898,.T.);
#9661=ORIENTED_EDGE('',*,*,#6899,.T.);
#9662=ORIENTED_EDGE('',*,*,#6900,.T.);
#9663=ORIENTED_EDGE('',*,*,#6901,.F.);
#9664=ORIENTED_EDGE('',*,*,#6902,.T.);
#9665=ORIENTED_EDGE('',*,*,#6903,.T.);
#9666=ORIENTED_EDGE('',*,*,#6904,.T.);
#9667=ORIENTED_EDGE('',*,*,#6905,.T.);
#9668=ORIENTED_EDGE('',*,*,#6906,.T.);
#9669=ORIENTED_EDGE('',*,*,#6907,.T.);
#9670=ORIENTED_EDGE('',*,*,#6908,.T.);
#9671=ORIENTED_EDGE('',*,*,#6909,.T.);
#9672=ORIENTED_EDGE('',*,*,#6910,.F.);
#9673=ORIENTED_EDGE('',*,*,#6911,.T.);
#9674=ORIENTED_EDGE('',*,*,#6912,.T.);
#9675=ORIENTED_EDGE('',*,*,#6900,.F.);
#9676=ORIENTED_EDGE('',*,*,#6912,.F.);
#9677=ORIENTED_EDGE('',*,*,#6913,.T.);
#9678=ORIENTED_EDGE('',*,*,#6914,.T.);
#9679=ORIENTED_EDGE('',*,*,#6901,.T.);
#9680=ORIENTED_EDGE('',*,*,#6914,.F.);
#9681=ORIENTED_EDGE('',*,*,#6915,.T.);
#9682=ORIENTED_EDGE('',*,*,#6916,.T.);
#9683=ORIENTED_EDGE('',*,*,#6902,.F.);
#9684=ORIENTED_EDGE('',*,*,#6916,.F.);
#9685=ORIENTED_EDGE('',*,*,#6917,.T.);
#9686=ORIENTED_EDGE('',*,*,#6918,.T.);
#9687=ORIENTED_EDGE('',*,*,#6903,.F.);
#9688=ORIENTED_EDGE('',*,*,#6918,.F.);
#9689=ORIENTED_EDGE('',*,*,#6919,.T.);
#9690=ORIENTED_EDGE('',*,*,#6920,.T.);
#9691=ORIENTED_EDGE('',*,*,#6904,.F.);
#9692=ORIENTED_EDGE('',*,*,#6920,.F.);
#9693=ORIENTED_EDGE('',*,*,#6921,.T.);
#9694=ORIENTED_EDGE('',*,*,#6922,.T.);
#9695=ORIENTED_EDGE('',*,*,#6905,.F.);
#9696=ORIENTED_EDGE('',*,*,#6922,.F.);
#9697=ORIENTED_EDGE('',*,*,#6923,.T.);
#9698=ORIENTED_EDGE('',*,*,#6924,.T.);
#9699=ORIENTED_EDGE('',*,*,#6906,.F.);
#9700=ORIENTED_EDGE('',*,*,#6924,.F.);
#9701=ORIENTED_EDGE('',*,*,#6925,.T.);
#9702=ORIENTED_EDGE('',*,*,#6926,.T.);
#9703=ORIENTED_EDGE('',*,*,#6907,.F.);
#9704=ORIENTED_EDGE('',*,*,#6926,.F.);
#9705=ORIENTED_EDGE('',*,*,#6927,.T.);
#9706=ORIENTED_EDGE('',*,*,#6928,.T.);
#9707=ORIENTED_EDGE('',*,*,#6908,.F.);
#9708=ORIENTED_EDGE('',*,*,#6928,.F.);
#9709=ORIENTED_EDGE('',*,*,#6929,.T.);
#9710=ORIENTED_EDGE('',*,*,#6930,.T.);
#9711=ORIENTED_EDGE('',*,*,#6909,.F.);
#9712=ORIENTED_EDGE('',*,*,#6930,.F.);
#9713=ORIENTED_EDGE('',*,*,#6931,.T.);
#9714=ORIENTED_EDGE('',*,*,#6932,.T.);
#9715=ORIENTED_EDGE('',*,*,#6898,.F.);
#9716=ORIENTED_EDGE('',*,*,#6932,.F.);
#9717=ORIENTED_EDGE('',*,*,#6933,.T.);
#9718=ORIENTED_EDGE('',*,*,#6910,.T.);
#9719=ORIENTED_EDGE('',*,*,#6899,.F.);
#9720=ORIENTED_EDGE('',*,*,#6931,.F.);
#9721=ORIENTED_EDGE('',*,*,#6929,.F.);
#9722=ORIENTED_EDGE('',*,*,#6927,.F.);
#9723=ORIENTED_EDGE('',*,*,#6925,.F.);
#9724=ORIENTED_EDGE('',*,*,#6923,.F.);
#9725=ORIENTED_EDGE('',*,*,#6921,.F.);
#9726=ORIENTED_EDGE('',*,*,#6919,.F.);
#9727=ORIENTED_EDGE('',*,*,#6917,.F.);
#9728=ORIENTED_EDGE('',*,*,#6915,.F.);
#9729=ORIENTED_EDGE('',*,*,#6913,.F.);
#9730=ORIENTED_EDGE('',*,*,#6911,.F.);
#9731=ORIENTED_EDGE('',*,*,#6933,.F.);
#9732=ORIENTED_EDGE('',*,*,#6934,.F.);
#9733=ORIENTED_EDGE('',*,*,#6935,.F.);
#9734=ORIENTED_EDGE('',*,*,#6936,.F.);
#9735=ORIENTED_EDGE('',*,*,#6937,.T.);
#9736=ORIENTED_EDGE('',*,*,#6938,.F.);
#9737=ORIENTED_EDGE('',*,*,#6939,.F.);
#9738=ORIENTED_EDGE('',*,*,#6940,.F.);
#9739=ORIENTED_EDGE('',*,*,#6935,.T.);
#9740=ORIENTED_EDGE('',*,*,#6941,.F.);
#9741=ORIENTED_EDGE('',*,*,#6942,.F.);
#9742=ORIENTED_EDGE('',*,*,#6943,.F.);
#9743=ORIENTED_EDGE('',*,*,#6939,.T.);
#9744=ORIENTED_EDGE('',*,*,#6944,.F.);
#9745=ORIENTED_EDGE('',*,*,#6945,.F.);
#9746=ORIENTED_EDGE('',*,*,#6946,.F.);
#9747=ORIENTED_EDGE('',*,*,#6942,.T.);
#9748=ORIENTED_EDGE('',*,*,#6947,.F.);
#9749=ORIENTED_EDGE('',*,*,#6948,.F.);
#9750=ORIENTED_EDGE('',*,*,#6949,.F.);
#9751=ORIENTED_EDGE('',*,*,#6945,.T.);
#9752=ORIENTED_EDGE('',*,*,#6950,.F.);
#9753=ORIENTED_EDGE('',*,*,#6951,.F.);
#9754=ORIENTED_EDGE('',*,*,#6952,.F.);
#9755=ORIENTED_EDGE('',*,*,#6948,.T.);
#9756=ORIENTED_EDGE('',*,*,#6953,.F.);
#9757=ORIENTED_EDGE('',*,*,#6954,.F.);
#9758=ORIENTED_EDGE('',*,*,#6955,.F.);
#9759=ORIENTED_EDGE('',*,*,#6951,.T.);
#9760=ORIENTED_EDGE('',*,*,#6956,.F.);
#9761=ORIENTED_EDGE('',*,*,#6957,.F.);
#9762=ORIENTED_EDGE('',*,*,#6958,.F.);
#9763=ORIENTED_EDGE('',*,*,#6954,.T.);
#9764=ORIENTED_EDGE('',*,*,#6959,.F.);
#9765=ORIENTED_EDGE('',*,*,#6960,.F.);
#9766=ORIENTED_EDGE('',*,*,#6961,.F.);
#9767=ORIENTED_EDGE('',*,*,#6957,.T.);
#9768=ORIENTED_EDGE('',*,*,#6962,.F.);
#9769=ORIENTED_EDGE('',*,*,#6963,.F.);
#9770=ORIENTED_EDGE('',*,*,#6964,.F.);
#9771=ORIENTED_EDGE('',*,*,#6960,.T.);
#9772=ORIENTED_EDGE('',*,*,#6965,.F.);
#9773=ORIENTED_EDGE('',*,*,#6966,.F.);
#9774=ORIENTED_EDGE('',*,*,#6967,.T.);
#9775=ORIENTED_EDGE('',*,*,#6963,.T.);
#9776=ORIENTED_EDGE('',*,*,#6968,.F.);
#9777=ORIENTED_EDGE('',*,*,#6937,.F.);
#9778=ORIENTED_EDGE('',*,*,#6969,.F.);
#9779=ORIENTED_EDGE('',*,*,#6966,.T.);
#9780=ORIENTED_EDGE('',*,*,#6940,.T.);
#9781=ORIENTED_EDGE('',*,*,#6943,.T.);
#9782=ORIENTED_EDGE('',*,*,#6946,.T.);
#9783=ORIENTED_EDGE('',*,*,#6949,.T.);
#9784=ORIENTED_EDGE('',*,*,#6952,.T.);
#9785=ORIENTED_EDGE('',*,*,#6955,.T.);
#9786=ORIENTED_EDGE('',*,*,#6958,.T.);
#9787=ORIENTED_EDGE('',*,*,#6961,.T.);
#9788=ORIENTED_EDGE('',*,*,#6964,.T.);
#9789=ORIENTED_EDGE('',*,*,#6967,.F.);
#9790=ORIENTED_EDGE('',*,*,#6969,.T.);
#9791=ORIENTED_EDGE('',*,*,#6936,.T.);
#9792=ORIENTED_EDGE('',*,*,#6938,.T.);
#9793=ORIENTED_EDGE('',*,*,#6934,.T.);
#9794=ORIENTED_EDGE('',*,*,#6968,.T.);
#9795=ORIENTED_EDGE('',*,*,#6965,.T.);
#9796=ORIENTED_EDGE('',*,*,#6962,.T.);
#9797=ORIENTED_EDGE('',*,*,#6959,.T.);
#9798=ORIENTED_EDGE('',*,*,#6956,.T.);
#9799=ORIENTED_EDGE('',*,*,#6953,.T.);
#9800=ORIENTED_EDGE('',*,*,#6950,.T.);
#9801=ORIENTED_EDGE('',*,*,#6947,.T.);
#9802=ORIENTED_EDGE('',*,*,#6944,.T.);
#9803=ORIENTED_EDGE('',*,*,#6941,.T.);
#9804=ORIENTED_EDGE('',*,*,#6970,.T.);
#9805=ORIENTED_EDGE('',*,*,#6971,.T.);
#9806=ORIENTED_EDGE('',*,*,#6972,.T.);
#9807=ORIENTED_EDGE('',*,*,#6973,.T.);
#9808=ORIENTED_EDGE('',*,*,#6974,.T.);
#9809=ORIENTED_EDGE('',*,*,#6975,.T.);
#9810=ORIENTED_EDGE('',*,*,#6976,.T.);
#9811=ORIENTED_EDGE('',*,*,#6977,.T.);
#9812=ORIENTED_EDGE('',*,*,#6978,.T.);
#9813=ORIENTED_EDGE('',*,*,#6979,.T.);
#9814=ORIENTED_EDGE('',*,*,#6980,.T.);
#9815=ORIENTED_EDGE('',*,*,#6981,.T.);
#9816=ORIENTED_EDGE('',*,*,#6982,.F.);
#9817=ORIENTED_EDGE('',*,*,#6983,.T.);
#9818=ORIENTED_EDGE('',*,*,#6984,.T.);
#9819=ORIENTED_EDGE('',*,*,#6972,.F.);
#9820=ORIENTED_EDGE('',*,*,#6984,.F.);
#9821=ORIENTED_EDGE('',*,*,#6985,.T.);
#9822=ORIENTED_EDGE('',*,*,#6986,.T.);
#9823=ORIENTED_EDGE('',*,*,#6973,.F.);
#9824=ORIENTED_EDGE('',*,*,#6986,.F.);
#9825=ORIENTED_EDGE('',*,*,#6987,.T.);
#9826=ORIENTED_EDGE('',*,*,#6988,.T.);
#9827=ORIENTED_EDGE('',*,*,#6974,.F.);
#9828=ORIENTED_EDGE('',*,*,#6988,.F.);
#9829=ORIENTED_EDGE('',*,*,#6989,.T.);
#9830=ORIENTED_EDGE('',*,*,#6990,.T.);
#9831=ORIENTED_EDGE('',*,*,#6975,.F.);
#9832=ORIENTED_EDGE('',*,*,#6990,.F.);
#9833=ORIENTED_EDGE('',*,*,#6991,.T.);
#9834=ORIENTED_EDGE('',*,*,#6992,.T.);
#9835=ORIENTED_EDGE('',*,*,#6976,.F.);
#9836=ORIENTED_EDGE('',*,*,#6992,.F.);
#9837=ORIENTED_EDGE('',*,*,#6993,.T.);
#9838=ORIENTED_EDGE('',*,*,#6994,.T.);
#9839=ORIENTED_EDGE('',*,*,#6977,.F.);
#9840=ORIENTED_EDGE('',*,*,#6994,.F.);
#9841=ORIENTED_EDGE('',*,*,#6995,.T.);
#9842=ORIENTED_EDGE('',*,*,#6996,.T.);
#9843=ORIENTED_EDGE('',*,*,#6978,.F.);
#9844=ORIENTED_EDGE('',*,*,#6996,.F.);
#9845=ORIENTED_EDGE('',*,*,#6997,.T.);
#9846=ORIENTED_EDGE('',*,*,#6998,.T.);
#9847=ORIENTED_EDGE('',*,*,#6979,.F.);
#9848=ORIENTED_EDGE('',*,*,#6998,.F.);
#9849=ORIENTED_EDGE('',*,*,#6999,.T.);
#9850=ORIENTED_EDGE('',*,*,#7000,.T.);
#9851=ORIENTED_EDGE('',*,*,#6980,.F.);
#9852=ORIENTED_EDGE('',*,*,#7000,.F.);
#9853=ORIENTED_EDGE('',*,*,#7001,.T.);
#9854=ORIENTED_EDGE('',*,*,#7002,.T.);
#9855=ORIENTED_EDGE('',*,*,#6981,.F.);
#9856=ORIENTED_EDGE('',*,*,#7002,.F.);
#9857=ORIENTED_EDGE('',*,*,#7003,.T.);
#9858=ORIENTED_EDGE('',*,*,#7004,.T.);
#9859=ORIENTED_EDGE('',*,*,#6970,.F.);
#9860=ORIENTED_EDGE('',*,*,#7004,.F.);
#9861=ORIENTED_EDGE('',*,*,#7005,.T.);
#9862=ORIENTED_EDGE('',*,*,#6982,.T.);
#9863=ORIENTED_EDGE('',*,*,#6971,.F.);
#9864=ORIENTED_EDGE('',*,*,#7003,.F.);
#9865=ORIENTED_EDGE('',*,*,#7001,.F.);
#9866=ORIENTED_EDGE('',*,*,#6999,.F.);
#9867=ORIENTED_EDGE('',*,*,#6997,.F.);
#9868=ORIENTED_EDGE('',*,*,#6995,.F.);
#9869=ORIENTED_EDGE('',*,*,#6993,.F.);
#9870=ORIENTED_EDGE('',*,*,#6991,.F.);
#9871=ORIENTED_EDGE('',*,*,#6989,.F.);
#9872=ORIENTED_EDGE('',*,*,#6987,.F.);
#9873=ORIENTED_EDGE('',*,*,#6985,.F.);
#9874=ORIENTED_EDGE('',*,*,#6983,.F.);
#9875=ORIENTED_EDGE('',*,*,#7005,.F.);
#9876=ORIENTED_EDGE('',*,*,#7006,.T.);
#9877=ORIENTED_EDGE('',*,*,#7007,.T.);
#9878=ORIENTED_EDGE('',*,*,#7008,.T.);
#9879=ORIENTED_EDGE('',*,*,#7009,.T.);
#9880=ORIENTED_EDGE('',*,*,#7010,.T.);
#9881=ORIENTED_EDGE('',*,*,#7011,.T.);
#9882=ORIENTED_EDGE('',*,*,#7012,.T.);
#9883=ORIENTED_EDGE('',*,*,#7013,.T.);
#9884=ORIENTED_EDGE('',*,*,#7014,.T.);
#9885=ORIENTED_EDGE('',*,*,#7015,.T.);
#9886=ORIENTED_EDGE('',*,*,#7016,.T.);
#9887=ORIENTED_EDGE('',*,*,#7017,.T.);
#9888=ORIENTED_EDGE('',*,*,#7018,.T.);
#9889=ORIENTED_EDGE('',*,*,#7019,.T.);
#9890=ORIENTED_EDGE('',*,*,#7020,.F.);
#9891=ORIENTED_EDGE('',*,*,#7017,.F.);
#9892=ORIENTED_EDGE('',*,*,#7021,.T.);
#9893=ORIENTED_EDGE('',*,*,#7022,.T.);
#9894=ORIENTED_EDGE('',*,*,#7018,.F.);
#9895=ORIENTED_EDGE('',*,*,#7016,.F.);
#9896=ORIENTED_EDGE('',*,*,#7023,.T.);
#9897=ORIENTED_EDGE('',*,*,#7024,.T.);
#9898=ORIENTED_EDGE('',*,*,#7021,.F.);
#9899=ORIENTED_EDGE('',*,*,#7015,.F.);
#9900=ORIENTED_EDGE('',*,*,#7025,.T.);
#9901=ORIENTED_EDGE('',*,*,#7026,.T.);
#9902=ORIENTED_EDGE('',*,*,#7023,.F.);
#9903=ORIENTED_EDGE('',*,*,#7014,.F.);
#9904=ORIENTED_EDGE('',*,*,#7027,.T.);
#9905=ORIENTED_EDGE('',*,*,#7028,.T.);
#9906=ORIENTED_EDGE('',*,*,#7025,.F.);
#9907=ORIENTED_EDGE('',*,*,#7013,.F.);
#9908=ORIENTED_EDGE('',*,*,#7029,.T.);
#9909=ORIENTED_EDGE('',*,*,#7030,.T.);
#9910=ORIENTED_EDGE('',*,*,#7027,.F.);
#9911=ORIENTED_EDGE('',*,*,#7012,.F.);
#9912=ORIENTED_EDGE('',*,*,#7031,.T.);
#9913=ORIENTED_EDGE('',*,*,#7032,.T.);
#9914=ORIENTED_EDGE('',*,*,#7029,.F.);
#9915=ORIENTED_EDGE('',*,*,#7011,.F.);
#9916=ORIENTED_EDGE('',*,*,#7033,.T.);
#9917=ORIENTED_EDGE('',*,*,#7034,.T.);
#9918=ORIENTED_EDGE('',*,*,#7031,.F.);
#9919=ORIENTED_EDGE('',*,*,#7010,.F.);
#9920=ORIENTED_EDGE('',*,*,#7035,.T.);
#9921=ORIENTED_EDGE('',*,*,#7036,.T.);
#9922=ORIENTED_EDGE('',*,*,#7033,.F.);
#9923=ORIENTED_EDGE('',*,*,#7009,.F.);
#9924=ORIENTED_EDGE('',*,*,#7037,.T.);
#9925=ORIENTED_EDGE('',*,*,#7038,.T.);
#9926=ORIENTED_EDGE('',*,*,#7035,.F.);
#9927=ORIENTED_EDGE('',*,*,#7008,.F.);
#9928=ORIENTED_EDGE('',*,*,#7039,.T.);
#9929=ORIENTED_EDGE('',*,*,#7040,.T.);
#9930=ORIENTED_EDGE('',*,*,#7037,.F.);
#9931=ORIENTED_EDGE('',*,*,#7007,.F.);
#9932=ORIENTED_EDGE('',*,*,#7020,.T.);
#9933=ORIENTED_EDGE('',*,*,#7041,.T.);
#9934=ORIENTED_EDGE('',*,*,#7039,.F.);
#9935=ORIENTED_EDGE('',*,*,#7006,.F.);
#9936=ORIENTED_EDGE('',*,*,#7019,.F.);
#9937=ORIENTED_EDGE('',*,*,#7022,.F.);
#9938=ORIENTED_EDGE('',*,*,#7024,.F.);
#9939=ORIENTED_EDGE('',*,*,#7026,.F.);
#9940=ORIENTED_EDGE('',*,*,#7028,.F.);
#9941=ORIENTED_EDGE('',*,*,#7030,.F.);
#9942=ORIENTED_EDGE('',*,*,#7032,.F.);
#9943=ORIENTED_EDGE('',*,*,#7034,.F.);
#9944=ORIENTED_EDGE('',*,*,#7036,.F.);
#9945=ORIENTED_EDGE('',*,*,#7038,.F.);
#9946=ORIENTED_EDGE('',*,*,#7040,.F.);
#9947=ORIENTED_EDGE('',*,*,#7041,.F.);
#9948=ORIENTED_EDGE('',*,*,#7042,.F.);
#9949=ORIENTED_EDGE('',*,*,#7043,.F.);
#9950=ORIENTED_EDGE('',*,*,#7044,.F.);
#9951=ORIENTED_EDGE('',*,*,#7045,.F.);
#9952=ORIENTED_EDGE('',*,*,#7046,.F.);
#9953=ORIENTED_EDGE('',*,*,#7047,.F.);
#9954=ORIENTED_EDGE('',*,*,#7048,.F.);
#9955=ORIENTED_EDGE('',*,*,#7049,.F.);
#9956=ORIENTED_EDGE('',*,*,#7050,.F.);
#9957=ORIENTED_EDGE('',*,*,#7051,.F.);
#9958=ORIENTED_EDGE('',*,*,#7052,.F.);
#9959=ORIENTED_EDGE('',*,*,#7053,.F.);
#9960=ORIENTED_EDGE('',*,*,#7054,.F.);
#9961=ORIENTED_EDGE('',*,*,#7055,.T.);
#9962=ORIENTED_EDGE('',*,*,#7056,.T.);
#9963=ORIENTED_EDGE('',*,*,#7043,.T.);
#9964=ORIENTED_EDGE('',*,*,#7056,.F.);
#9965=ORIENTED_EDGE('',*,*,#7057,.T.);
#9966=ORIENTED_EDGE('',*,*,#7058,.T.);
#9967=ORIENTED_EDGE('',*,*,#7044,.T.);
#9968=ORIENTED_EDGE('',*,*,#7058,.F.);
#9969=ORIENTED_EDGE('',*,*,#7059,.T.);
#9970=ORIENTED_EDGE('',*,*,#7060,.T.);
#9971=ORIENTED_EDGE('',*,*,#7045,.T.);
#9972=ORIENTED_EDGE('',*,*,#7060,.F.);
#9973=ORIENTED_EDGE('',*,*,#7061,.T.);
#9974=ORIENTED_EDGE('',*,*,#7062,.T.);
#9975=ORIENTED_EDGE('',*,*,#7046,.T.);
#9976=ORIENTED_EDGE('',*,*,#7062,.F.);
#9977=ORIENTED_EDGE('',*,*,#7063,.T.);
#9978=ORIENTED_EDGE('',*,*,#7064,.T.);
#9979=ORIENTED_EDGE('',*,*,#7047,.T.);
#9980=ORIENTED_EDGE('',*,*,#7064,.F.);
#9981=ORIENTED_EDGE('',*,*,#7065,.T.);
#9982=ORIENTED_EDGE('',*,*,#7066,.T.);
#9983=ORIENTED_EDGE('',*,*,#7048,.T.);
#9984=ORIENTED_EDGE('',*,*,#7066,.F.);
#9985=ORIENTED_EDGE('',*,*,#7067,.T.);
#9986=ORIENTED_EDGE('',*,*,#7068,.T.);
#9987=ORIENTED_EDGE('',*,*,#7049,.T.);
#9988=ORIENTED_EDGE('',*,*,#7068,.F.);
#9989=ORIENTED_EDGE('',*,*,#7069,.T.);
#9990=ORIENTED_EDGE('',*,*,#7070,.T.);
#9991=ORIENTED_EDGE('',*,*,#7050,.T.);
#9992=ORIENTED_EDGE('',*,*,#7070,.F.);
#9993=ORIENTED_EDGE('',*,*,#7071,.T.);
#9994=ORIENTED_EDGE('',*,*,#7072,.T.);
#9995=ORIENTED_EDGE('',*,*,#7051,.T.);
#9996=ORIENTED_EDGE('',*,*,#7072,.F.);
#9997=ORIENTED_EDGE('',*,*,#7073,.T.);
#9998=ORIENTED_EDGE('',*,*,#7074,.T.);
#9999=ORIENTED_EDGE('',*,*,#7052,.T.);
#10000=ORIENTED_EDGE('',*,*,#7074,.F.);
#10001=ORIENTED_EDGE('',*,*,#7075,.T.);
#10002=ORIENTED_EDGE('',*,*,#7076,.T.);
#10003=ORIENTED_EDGE('',*,*,#7053,.T.);
#10004=ORIENTED_EDGE('',*,*,#7076,.F.);
#10005=ORIENTED_EDGE('',*,*,#7077,.T.);
#10006=ORIENTED_EDGE('',*,*,#7054,.T.);
#10007=ORIENTED_EDGE('',*,*,#7042,.T.);
#10008=ORIENTED_EDGE('',*,*,#7075,.F.);
#10009=ORIENTED_EDGE('',*,*,#7073,.F.);
#10010=ORIENTED_EDGE('',*,*,#7071,.F.);
#10011=ORIENTED_EDGE('',*,*,#7069,.F.);
#10012=ORIENTED_EDGE('',*,*,#7067,.F.);
#10013=ORIENTED_EDGE('',*,*,#7065,.F.);
#10014=ORIENTED_EDGE('',*,*,#7063,.F.);
#10015=ORIENTED_EDGE('',*,*,#7061,.F.);
#10016=ORIENTED_EDGE('',*,*,#7059,.F.);
#10017=ORIENTED_EDGE('',*,*,#7057,.F.);
#10018=ORIENTED_EDGE('',*,*,#7055,.F.);
#10019=ORIENTED_EDGE('',*,*,#7077,.F.);
#10020=ORIENTED_EDGE('',*,*,#7078,.T.);
#10021=ORIENTED_EDGE('',*,*,#7079,.F.);
#10022=ORIENTED_EDGE('',*,*,#7080,.F.);
#10023=ORIENTED_EDGE('',*,*,#7081,.T.);
#10024=ORIENTED_EDGE('',*,*,#7082,.T.);
#10025=ORIENTED_EDGE('',*,*,#7083,.F.);
#10026=ORIENTED_EDGE('',*,*,#7084,.F.);
#10027=ORIENTED_EDGE('',*,*,#7079,.T.);
#10028=ORIENTED_EDGE('',*,*,#7085,.T.);
#10029=ORIENTED_EDGE('',*,*,#7086,.F.);
#10030=ORIENTED_EDGE('',*,*,#7087,.F.);
#10031=ORIENTED_EDGE('',*,*,#7083,.T.);
#10032=ORIENTED_EDGE('',*,*,#7088,.T.);
#10033=ORIENTED_EDGE('',*,*,#7089,.F.);
#10034=ORIENTED_EDGE('',*,*,#7090,.F.);
#10035=ORIENTED_EDGE('',*,*,#7086,.T.);
#10036=ORIENTED_EDGE('',*,*,#7091,.T.);
#10037=ORIENTED_EDGE('',*,*,#7092,.F.);
#10038=ORIENTED_EDGE('',*,*,#7093,.F.);
#10039=ORIENTED_EDGE('',*,*,#7089,.T.);
#10040=ORIENTED_EDGE('',*,*,#7094,.T.);
#10041=ORIENTED_EDGE('',*,*,#7095,.F.);
#10042=ORIENTED_EDGE('',*,*,#7096,.F.);
#10043=ORIENTED_EDGE('',*,*,#7092,.T.);
#10044=ORIENTED_EDGE('',*,*,#7097,.T.);
#10045=ORIENTED_EDGE('',*,*,#7098,.F.);
#10046=ORIENTED_EDGE('',*,*,#7099,.F.);
#10047=ORIENTED_EDGE('',*,*,#7095,.T.);
#10048=ORIENTED_EDGE('',*,*,#7100,.T.);
#10049=ORIENTED_EDGE('',*,*,#7101,.F.);
#10050=ORIENTED_EDGE('',*,*,#7102,.F.);
#10051=ORIENTED_EDGE('',*,*,#7098,.T.);
#10052=ORIENTED_EDGE('',*,*,#7103,.T.);
#10053=ORIENTED_EDGE('',*,*,#7081,.F.);
#10054=ORIENTED_EDGE('',*,*,#7104,.F.);
#10055=ORIENTED_EDGE('',*,*,#7101,.T.);
#10056=ORIENTED_EDGE('',*,*,#7080,.T.);
#10057=ORIENTED_EDGE('',*,*,#7084,.T.);
#10058=ORIENTED_EDGE('',*,*,#7087,.T.);
#10059=ORIENTED_EDGE('',*,*,#7090,.T.);
#10060=ORIENTED_EDGE('',*,*,#7093,.T.);
#10061=ORIENTED_EDGE('',*,*,#7096,.T.);
#10062=ORIENTED_EDGE('',*,*,#7099,.T.);
#10063=ORIENTED_EDGE('',*,*,#7102,.T.);
#10064=ORIENTED_EDGE('',*,*,#7104,.T.);
#10065=ORIENTED_EDGE('',*,*,#7078,.F.);
#10066=ORIENTED_EDGE('',*,*,#7103,.F.);
#10067=ORIENTED_EDGE('',*,*,#7100,.F.);
#10068=ORIENTED_EDGE('',*,*,#7097,.F.);
#10069=ORIENTED_EDGE('',*,*,#7094,.F.);
#10070=ORIENTED_EDGE('',*,*,#7091,.F.);
#10071=ORIENTED_EDGE('',*,*,#7088,.F.);
#10072=ORIENTED_EDGE('',*,*,#7085,.F.);
#10073=ORIENTED_EDGE('',*,*,#7082,.F.);
#10074=ORIENTED_EDGE('',*,*,#7105,.T.);
#10075=ORIENTED_EDGE('',*,*,#7106,.F.);
#10076=ORIENTED_EDGE('',*,*,#7107,.F.);
#10077=ORIENTED_EDGE('',*,*,#7108,.T.);
#10078=ORIENTED_EDGE('',*,*,#7109,.T.);
#10079=ORIENTED_EDGE('',*,*,#7110,.F.);
#10080=ORIENTED_EDGE('',*,*,#7111,.F.);
#10081=ORIENTED_EDGE('',*,*,#7106,.T.);
#10082=ORIENTED_EDGE('',*,*,#7112,.T.);
#10083=ORIENTED_EDGE('',*,*,#7113,.F.);
#10084=ORIENTED_EDGE('',*,*,#7114,.F.);
#10085=ORIENTED_EDGE('',*,*,#7110,.T.);
#10086=ORIENTED_EDGE('',*,*,#7115,.T.);
#10087=ORIENTED_EDGE('',*,*,#7116,.F.);
#10088=ORIENTED_EDGE('',*,*,#7117,.F.);
#10089=ORIENTED_EDGE('',*,*,#7113,.T.);
#10090=ORIENTED_EDGE('',*,*,#7118,.T.);
#10091=ORIENTED_EDGE('',*,*,#7119,.F.);
#10092=ORIENTED_EDGE('',*,*,#7120,.F.);
#10093=ORIENTED_EDGE('',*,*,#7116,.T.);
#10094=ORIENTED_EDGE('',*,*,#7121,.T.);
#10095=ORIENTED_EDGE('',*,*,#7122,.F.);
#10096=ORIENTED_EDGE('',*,*,#7123,.F.);
#10097=ORIENTED_EDGE('',*,*,#7119,.T.);
#10098=ORIENTED_EDGE('',*,*,#7124,.T.);
#10099=ORIENTED_EDGE('',*,*,#7125,.F.);
#10100=ORIENTED_EDGE('',*,*,#7126,.F.);
#10101=ORIENTED_EDGE('',*,*,#7122,.T.);
#10102=ORIENTED_EDGE('',*,*,#7127,.T.);
#10103=ORIENTED_EDGE('',*,*,#7128,.F.);
#10104=ORIENTED_EDGE('',*,*,#7129,.F.);
#10105=ORIENTED_EDGE('',*,*,#7125,.T.);
#10106=ORIENTED_EDGE('',*,*,#7130,.T.);
#10107=ORIENTED_EDGE('',*,*,#7108,.F.);
#10108=ORIENTED_EDGE('',*,*,#7131,.F.);
#10109=ORIENTED_EDGE('',*,*,#7128,.T.);
#10110=ORIENTED_EDGE('',*,*,#7107,.T.);
#10111=ORIENTED_EDGE('',*,*,#7111,.T.);
#10112=ORIENTED_EDGE('',*,*,#7114,.T.);
#10113=ORIENTED_EDGE('',*,*,#7117,.T.);
#10114=ORIENTED_EDGE('',*,*,#7120,.T.);
#10115=ORIENTED_EDGE('',*,*,#7123,.T.);
#10116=ORIENTED_EDGE('',*,*,#7126,.T.);
#10117=ORIENTED_EDGE('',*,*,#7129,.T.);
#10118=ORIENTED_EDGE('',*,*,#7131,.T.);
#10119=ORIENTED_EDGE('',*,*,#7105,.F.);
#10120=ORIENTED_EDGE('',*,*,#7130,.F.);
#10121=ORIENTED_EDGE('',*,*,#7127,.F.);
#10122=ORIENTED_EDGE('',*,*,#7124,.F.);
#10123=ORIENTED_EDGE('',*,*,#7121,.F.);
#10124=ORIENTED_EDGE('',*,*,#7118,.F.);
#10125=ORIENTED_EDGE('',*,*,#7115,.F.);
#10126=ORIENTED_EDGE('',*,*,#7112,.F.);
#10127=ORIENTED_EDGE('',*,*,#7109,.F.);
#10128=ORIENTED_EDGE('',*,*,#7132,.F.);
#10129=ORIENTED_EDGE('',*,*,#7133,.F.);
#10130=ORIENTED_EDGE('',*,*,#7134,.T.);
#10131=ORIENTED_EDGE('',*,*,#7135,.T.);
#10132=ORIENTED_EDGE('',*,*,#7136,.F.);
#10133=ORIENTED_EDGE('',*,*,#7135,.F.);
#10134=ORIENTED_EDGE('',*,*,#7137,.T.);
#10135=ORIENTED_EDGE('',*,*,#7138,.T.);
#10136=ORIENTED_EDGE('',*,*,#7139,.F.);
#10137=ORIENTED_EDGE('',*,*,#7138,.F.);
#10138=ORIENTED_EDGE('',*,*,#7140,.T.);
#10139=ORIENTED_EDGE('',*,*,#7141,.T.);
#10140=ORIENTED_EDGE('',*,*,#7142,.F.);
#10141=ORIENTED_EDGE('',*,*,#7141,.F.);
#10142=ORIENTED_EDGE('',*,*,#7143,.T.);
#10143=ORIENTED_EDGE('',*,*,#7144,.T.);
#10144=ORIENTED_EDGE('',*,*,#7145,.F.);
#10145=ORIENTED_EDGE('',*,*,#7144,.F.);
#10146=ORIENTED_EDGE('',*,*,#7146,.T.);
#10147=ORIENTED_EDGE('',*,*,#7147,.T.);
#10148=ORIENTED_EDGE('',*,*,#7148,.F.);
#10149=ORIENTED_EDGE('',*,*,#7147,.F.);
#10150=ORIENTED_EDGE('',*,*,#7149,.T.);
#10151=ORIENTED_EDGE('',*,*,#7150,.T.);
#10152=ORIENTED_EDGE('',*,*,#7151,.F.);
#10153=ORIENTED_EDGE('',*,*,#7150,.F.);
#10154=ORIENTED_EDGE('',*,*,#7152,.T.);
#10155=ORIENTED_EDGE('',*,*,#7153,.T.);
#10156=ORIENTED_EDGE('',*,*,#7154,.F.);
#10157=ORIENTED_EDGE('',*,*,#7153,.F.);
#10158=ORIENTED_EDGE('',*,*,#7155,.T.);
#10159=ORIENTED_EDGE('',*,*,#7156,.T.);
#10160=ORIENTED_EDGE('',*,*,#7157,.F.);
#10161=ORIENTED_EDGE('',*,*,#7156,.F.);
#10162=ORIENTED_EDGE('',*,*,#7158,.T.);
#10163=ORIENTED_EDGE('',*,*,#7133,.T.);
#10164=ORIENTED_EDGE('',*,*,#7134,.F.);
#10165=ORIENTED_EDGE('',*,*,#7158,.F.);
#10166=ORIENTED_EDGE('',*,*,#7155,.F.);
#10167=ORIENTED_EDGE('',*,*,#7152,.F.);
#10168=ORIENTED_EDGE('',*,*,#7149,.F.);
#10169=ORIENTED_EDGE('',*,*,#7146,.F.);
#10170=ORIENTED_EDGE('',*,*,#7143,.F.);
#10171=ORIENTED_EDGE('',*,*,#7140,.F.);
#10172=ORIENTED_EDGE('',*,*,#7137,.F.);
#10173=ORIENTED_EDGE('',*,*,#7132,.T.);
#10174=ORIENTED_EDGE('',*,*,#7136,.T.);
#10175=ORIENTED_EDGE('',*,*,#7139,.T.);
#10176=ORIENTED_EDGE('',*,*,#7142,.T.);
#10177=ORIENTED_EDGE('',*,*,#7145,.T.);
#10178=ORIENTED_EDGE('',*,*,#7148,.T.);
#10179=ORIENTED_EDGE('',*,*,#7151,.T.);
#10180=ORIENTED_EDGE('',*,*,#7154,.T.);
#10181=ORIENTED_EDGE('',*,*,#7157,.T.);
#10182=ORIENTED_EDGE('',*,*,#7159,.F.);
#10183=ORIENTED_EDGE('',*,*,#7160,.F.);
#10184=ORIENTED_EDGE('',*,*,#7161,.T.);
#10185=ORIENTED_EDGE('',*,*,#7162,.T.);
#10186=ORIENTED_EDGE('',*,*,#7163,.F.);
#10187=ORIENTED_EDGE('',*,*,#7162,.F.);
#10188=ORIENTED_EDGE('',*,*,#7164,.T.);
#10189=ORIENTED_EDGE('',*,*,#7165,.T.);
#10190=ORIENTED_EDGE('',*,*,#7166,.F.);
#10191=ORIENTED_EDGE('',*,*,#7165,.F.);
#10192=ORIENTED_EDGE('',*,*,#7167,.T.);
#10193=ORIENTED_EDGE('',*,*,#7168,.T.);
#10194=ORIENTED_EDGE('',*,*,#7169,.F.);
#10195=ORIENTED_EDGE('',*,*,#7168,.F.);
#10196=ORIENTED_EDGE('',*,*,#7170,.T.);
#10197=ORIENTED_EDGE('',*,*,#7171,.T.);
#10198=ORIENTED_EDGE('',*,*,#7172,.F.);
#10199=ORIENTED_EDGE('',*,*,#7171,.F.);
#10200=ORIENTED_EDGE('',*,*,#7173,.T.);
#10201=ORIENTED_EDGE('',*,*,#7174,.T.);
#10202=ORIENTED_EDGE('',*,*,#7175,.F.);
#10203=ORIENTED_EDGE('',*,*,#7174,.F.);
#10204=ORIENTED_EDGE('',*,*,#7176,.T.);
#10205=ORIENTED_EDGE('',*,*,#7177,.T.);
#10206=ORIENTED_EDGE('',*,*,#7178,.F.);
#10207=ORIENTED_EDGE('',*,*,#7177,.F.);
#10208=ORIENTED_EDGE('',*,*,#7179,.T.);
#10209=ORIENTED_EDGE('',*,*,#7180,.T.);
#10210=ORIENTED_EDGE('',*,*,#7181,.F.);
#10211=ORIENTED_EDGE('',*,*,#7180,.F.);
#10212=ORIENTED_EDGE('',*,*,#7182,.T.);
#10213=ORIENTED_EDGE('',*,*,#7183,.T.);
#10214=ORIENTED_EDGE('',*,*,#7184,.F.);
#10215=ORIENTED_EDGE('',*,*,#7183,.F.);
#10216=ORIENTED_EDGE('',*,*,#7185,.T.);
#10217=ORIENTED_EDGE('',*,*,#7160,.T.);
#10218=ORIENTED_EDGE('',*,*,#7161,.F.);
#10219=ORIENTED_EDGE('',*,*,#7185,.F.);
#10220=ORIENTED_EDGE('',*,*,#7182,.F.);
#10221=ORIENTED_EDGE('',*,*,#7179,.F.);
#10222=ORIENTED_EDGE('',*,*,#7176,.F.);
#10223=ORIENTED_EDGE('',*,*,#7173,.F.);
#10224=ORIENTED_EDGE('',*,*,#7170,.F.);
#10225=ORIENTED_EDGE('',*,*,#7167,.F.);
#10226=ORIENTED_EDGE('',*,*,#7164,.F.);
#10227=ORIENTED_EDGE('',*,*,#7159,.T.);
#10228=ORIENTED_EDGE('',*,*,#7163,.T.);
#10229=ORIENTED_EDGE('',*,*,#7166,.T.);
#10230=ORIENTED_EDGE('',*,*,#7169,.T.);
#10231=ORIENTED_EDGE('',*,*,#7172,.T.);
#10232=ORIENTED_EDGE('',*,*,#7175,.T.);
#10233=ORIENTED_EDGE('',*,*,#7178,.T.);
#10234=ORIENTED_EDGE('',*,*,#7181,.T.);
#10235=ORIENTED_EDGE('',*,*,#7184,.T.);
#10236=ORIENTED_EDGE('',*,*,#7186,.T.);
#10237=ORIENTED_EDGE('',*,*,#7187,.T.);
#10238=ORIENTED_EDGE('',*,*,#7188,.T.);
#10239=ORIENTED_EDGE('',*,*,#7189,.T.);
#10240=ORIENTED_EDGE('',*,*,#7190,.T.);
#10241=ORIENTED_EDGE('',*,*,#7191,.T.);
#10242=ORIENTED_EDGE('',*,*,#7192,.T.);
#10243=ORIENTED_EDGE('',*,*,#7193,.T.);
#10244=ORIENTED_EDGE('',*,*,#7194,.T.);
#10245=ORIENTED_EDGE('',*,*,#7195,.T.);
#10246=ORIENTED_EDGE('',*,*,#7196,.T.);
#10247=ORIENTED_EDGE('',*,*,#7197,.F.);
#10248=ORIENTED_EDGE('',*,*,#7194,.F.);
#10249=ORIENTED_EDGE('',*,*,#7198,.T.);
#10250=ORIENTED_EDGE('',*,*,#7199,.T.);
#10251=ORIENTED_EDGE('',*,*,#7195,.F.);
#10252=ORIENTED_EDGE('',*,*,#7193,.F.);
#10253=ORIENTED_EDGE('',*,*,#7200,.T.);
#10254=ORIENTED_EDGE('',*,*,#7201,.T.);
#10255=ORIENTED_EDGE('',*,*,#7198,.F.);
#10256=ORIENTED_EDGE('',*,*,#7192,.F.);
#10257=ORIENTED_EDGE('',*,*,#7202,.T.);
#10258=ORIENTED_EDGE('',*,*,#7203,.T.);
#10259=ORIENTED_EDGE('',*,*,#7200,.F.);
#10260=ORIENTED_EDGE('',*,*,#7191,.F.);
#10261=ORIENTED_EDGE('',*,*,#7204,.T.);
#10262=ORIENTED_EDGE('',*,*,#7205,.T.);
#10263=ORIENTED_EDGE('',*,*,#7202,.F.);
#10264=ORIENTED_EDGE('',*,*,#7190,.F.);
#10265=ORIENTED_EDGE('',*,*,#7206,.T.);
#10266=ORIENTED_EDGE('',*,*,#7207,.T.);
#10267=ORIENTED_EDGE('',*,*,#7204,.F.);
#10268=ORIENTED_EDGE('',*,*,#7189,.F.);
#10269=ORIENTED_EDGE('',*,*,#7208,.T.);
#10270=ORIENTED_EDGE('',*,*,#7209,.T.);
#10271=ORIENTED_EDGE('',*,*,#7206,.F.);
#10272=ORIENTED_EDGE('',*,*,#7188,.F.);
#10273=ORIENTED_EDGE('',*,*,#7210,.T.);
#10274=ORIENTED_EDGE('',*,*,#7211,.T.);
#10275=ORIENTED_EDGE('',*,*,#7208,.F.);
#10276=ORIENTED_EDGE('',*,*,#7187,.F.);
#10277=ORIENTED_EDGE('',*,*,#7197,.T.);
#10278=ORIENTED_EDGE('',*,*,#7212,.T.);
#10279=ORIENTED_EDGE('',*,*,#7210,.F.);
#10280=ORIENTED_EDGE('',*,*,#7186,.F.);
#10281=ORIENTED_EDGE('',*,*,#7196,.F.);
#10282=ORIENTED_EDGE('',*,*,#7199,.F.);
#10283=ORIENTED_EDGE('',*,*,#7201,.F.);
#10284=ORIENTED_EDGE('',*,*,#7203,.F.);
#10285=ORIENTED_EDGE('',*,*,#7205,.F.);
#10286=ORIENTED_EDGE('',*,*,#7207,.F.);
#10287=ORIENTED_EDGE('',*,*,#7209,.F.);
#10288=ORIENTED_EDGE('',*,*,#7211,.F.);
#10289=ORIENTED_EDGE('',*,*,#7212,.F.);
#10290=ORIENTED_EDGE('',*,*,#7213,.F.);
#10291=ORIENTED_EDGE('',*,*,#7214,.F.);
#10292=ORIENTED_EDGE('',*,*,#7215,.F.);
#10293=ORIENTED_EDGE('',*,*,#7216,.T.);
#10294=ORIENTED_EDGE('',*,*,#7217,.F.);
#10295=ORIENTED_EDGE('',*,*,#7218,.F.);
#10296=ORIENTED_EDGE('',*,*,#7219,.F.);
#10297=ORIENTED_EDGE('',*,*,#7214,.T.);
#10298=ORIENTED_EDGE('',*,*,#7220,.F.);
#10299=ORIENTED_EDGE('',*,*,#7221,.F.);
#10300=ORIENTED_EDGE('',*,*,#7222,.F.);
#10301=ORIENTED_EDGE('',*,*,#7218,.T.);
#10302=ORIENTED_EDGE('',*,*,#7223,.F.);
#10303=ORIENTED_EDGE('',*,*,#7224,.F.);
#10304=ORIENTED_EDGE('',*,*,#7225,.F.);
#10305=ORIENTED_EDGE('',*,*,#7221,.T.);
#10306=ORIENTED_EDGE('',*,*,#7226,.F.);
#10307=ORIENTED_EDGE('',*,*,#7227,.F.);
#10308=ORIENTED_EDGE('',*,*,#7228,.F.);
#10309=ORIENTED_EDGE('',*,*,#7224,.T.);
#10310=ORIENTED_EDGE('',*,*,#7229,.F.);
#10311=ORIENTED_EDGE('',*,*,#7230,.F.);
#10312=ORIENTED_EDGE('',*,*,#7231,.F.);
#10313=ORIENTED_EDGE('',*,*,#7227,.T.);
#10314=ORIENTED_EDGE('',*,*,#7232,.F.);
#10315=ORIENTED_EDGE('',*,*,#7233,.F.);
#10316=ORIENTED_EDGE('',*,*,#7234,.F.);
#10317=ORIENTED_EDGE('',*,*,#7230,.T.);
#10318=ORIENTED_EDGE('',*,*,#7235,.F.);
#10319=ORIENTED_EDGE('',*,*,#7236,.F.);
#10320=ORIENTED_EDGE('',*,*,#7237,.F.);
#10321=ORIENTED_EDGE('',*,*,#7233,.T.);
#10322=ORIENTED_EDGE('',*,*,#7238,.F.);
#10323=ORIENTED_EDGE('',*,*,#7216,.F.);
#10324=ORIENTED_EDGE('',*,*,#7239,.F.);
#10325=ORIENTED_EDGE('',*,*,#7236,.T.);
#10326=ORIENTED_EDGE('',*,*,#7239,.T.);
#10327=ORIENTED_EDGE('',*,*,#7215,.T.);
#10328=ORIENTED_EDGE('',*,*,#7219,.T.);
#10329=ORIENTED_EDGE('',*,*,#7222,.T.);
#10330=ORIENTED_EDGE('',*,*,#7225,.T.);
#10331=ORIENTED_EDGE('',*,*,#7228,.T.);
#10332=ORIENTED_EDGE('',*,*,#7231,.T.);
#10333=ORIENTED_EDGE('',*,*,#7234,.T.);
#10334=ORIENTED_EDGE('',*,*,#7237,.T.);
#10335=ORIENTED_EDGE('',*,*,#7217,.T.);
#10336=ORIENTED_EDGE('',*,*,#7213,.T.);
#10337=ORIENTED_EDGE('',*,*,#7238,.T.);
#10338=ORIENTED_EDGE('',*,*,#7235,.T.);
#10339=ORIENTED_EDGE('',*,*,#7232,.T.);
#10340=ORIENTED_EDGE('',*,*,#7229,.T.);
#10341=ORIENTED_EDGE('',*,*,#7226,.T.);
#10342=ORIENTED_EDGE('',*,*,#7223,.T.);
#10343=ORIENTED_EDGE('',*,*,#7220,.T.);
#10344=ORIENTED_EDGE('',*,*,#7240,.F.);
#10345=ORIENTED_EDGE('',*,*,#7241,.F.);
#10346=ORIENTED_EDGE('',*,*,#7242,.F.);
#10347=ORIENTED_EDGE('',*,*,#7243,.F.);
#10348=ORIENTED_EDGE('',*,*,#7244,.F.);
#10349=ORIENTED_EDGE('',*,*,#7245,.F.);
#10350=ORIENTED_EDGE('',*,*,#7246,.F.);
#10351=ORIENTED_EDGE('',*,*,#7247,.F.);
#10352=ORIENTED_EDGE('',*,*,#7248,.F.);
#10353=ORIENTED_EDGE('',*,*,#7249,.F.);
#10354=ORIENTED_EDGE('',*,*,#7250,.T.);
#10355=ORIENTED_EDGE('',*,*,#7251,.T.);
#10356=ORIENTED_EDGE('',*,*,#7241,.T.);
#10357=ORIENTED_EDGE('',*,*,#7251,.F.);
#10358=ORIENTED_EDGE('',*,*,#7252,.T.);
#10359=ORIENTED_EDGE('',*,*,#7253,.T.);
#10360=ORIENTED_EDGE('',*,*,#7242,.T.);
#10361=ORIENTED_EDGE('',*,*,#7253,.F.);
#10362=ORIENTED_EDGE('',*,*,#7254,.T.);
#10363=ORIENTED_EDGE('',*,*,#7255,.T.);
#10364=ORIENTED_EDGE('',*,*,#7243,.T.);
#10365=ORIENTED_EDGE('',*,*,#7255,.F.);
#10366=ORIENTED_EDGE('',*,*,#7256,.T.);
#10367=ORIENTED_EDGE('',*,*,#7257,.T.);
#10368=ORIENTED_EDGE('',*,*,#7244,.T.);
#10369=ORIENTED_EDGE('',*,*,#7257,.F.);
#10370=ORIENTED_EDGE('',*,*,#7258,.T.);
#10371=ORIENTED_EDGE('',*,*,#7259,.T.);
#10372=ORIENTED_EDGE('',*,*,#7245,.T.);
#10373=ORIENTED_EDGE('',*,*,#7259,.F.);
#10374=ORIENTED_EDGE('',*,*,#7260,.T.);
#10375=ORIENTED_EDGE('',*,*,#7261,.T.);
#10376=ORIENTED_EDGE('',*,*,#7246,.T.);
#10377=ORIENTED_EDGE('',*,*,#7261,.F.);
#10378=ORIENTED_EDGE('',*,*,#7262,.T.);
#10379=ORIENTED_EDGE('',*,*,#7263,.T.);
#10380=ORIENTED_EDGE('',*,*,#7247,.T.);
#10381=ORIENTED_EDGE('',*,*,#7263,.F.);
#10382=ORIENTED_EDGE('',*,*,#7264,.T.);
#10383=ORIENTED_EDGE('',*,*,#7265,.T.);
#10384=ORIENTED_EDGE('',*,*,#7248,.T.);
#10385=ORIENTED_EDGE('',*,*,#7265,.F.);
#10386=ORIENTED_EDGE('',*,*,#7266,.T.);
#10387=ORIENTED_EDGE('',*,*,#7249,.T.);
#10388=ORIENTED_EDGE('',*,*,#7240,.T.);
#10389=ORIENTED_EDGE('',*,*,#7264,.F.);
#10390=ORIENTED_EDGE('',*,*,#7262,.F.);
#10391=ORIENTED_EDGE('',*,*,#7260,.F.);
#10392=ORIENTED_EDGE('',*,*,#7258,.F.);
#10393=ORIENTED_EDGE('',*,*,#7256,.F.);
#10394=ORIENTED_EDGE('',*,*,#7254,.F.);
#10395=ORIENTED_EDGE('',*,*,#7252,.F.);
#10396=ORIENTED_EDGE('',*,*,#7250,.F.);
#10397=ORIENTED_EDGE('',*,*,#7266,.F.);
#10398=ORIENTED_EDGE('',*,*,#7267,.F.);
#10399=ORIENTED_EDGE('',*,*,#7268,.F.);
#10400=ORIENTED_EDGE('',*,*,#7269,.F.);
#10401=ORIENTED_EDGE('',*,*,#7270,.F.);
#10402=ORIENTED_EDGE('',*,*,#7271,.F.);
#10403=ORIENTED_EDGE('',*,*,#7272,.F.);
#10404=ORIENTED_EDGE('',*,*,#7273,.F.);
#10405=ORIENTED_EDGE('',*,*,#7274,.F.);
#10406=ORIENTED_EDGE('',*,*,#7275,.F.);
#10407=ORIENTED_EDGE('',*,*,#7276,.F.);
#10408=ORIENTED_EDGE('',*,*,#7277,.T.);
#10409=ORIENTED_EDGE('',*,*,#7278,.T.);
#10410=ORIENTED_EDGE('',*,*,#7268,.T.);
#10411=ORIENTED_EDGE('',*,*,#7278,.F.);
#10412=ORIENTED_EDGE('',*,*,#7279,.T.);
#10413=ORIENTED_EDGE('',*,*,#7280,.T.);
#10414=ORIENTED_EDGE('',*,*,#7269,.T.);
#10415=ORIENTED_EDGE('',*,*,#7280,.F.);
#10416=ORIENTED_EDGE('',*,*,#7281,.T.);
#10417=ORIENTED_EDGE('',*,*,#7282,.T.);
#10418=ORIENTED_EDGE('',*,*,#7270,.T.);
#10419=ORIENTED_EDGE('',*,*,#7282,.F.);
#10420=ORIENTED_EDGE('',*,*,#7283,.T.);
#10421=ORIENTED_EDGE('',*,*,#7284,.T.);
#10422=ORIENTED_EDGE('',*,*,#7271,.T.);
#10423=ORIENTED_EDGE('',*,*,#7284,.F.);
#10424=ORIENTED_EDGE('',*,*,#7285,.T.);
#10425=ORIENTED_EDGE('',*,*,#7286,.T.);
#10426=ORIENTED_EDGE('',*,*,#7272,.T.);
#10427=ORIENTED_EDGE('',*,*,#7286,.F.);
#10428=ORIENTED_EDGE('',*,*,#7287,.T.);
#10429=ORIENTED_EDGE('',*,*,#7288,.T.);
#10430=ORIENTED_EDGE('',*,*,#7273,.T.);
#10431=ORIENTED_EDGE('',*,*,#7288,.F.);
#10432=ORIENTED_EDGE('',*,*,#7289,.T.);
#10433=ORIENTED_EDGE('',*,*,#7290,.T.);
#10434=ORIENTED_EDGE('',*,*,#7274,.T.);
#10435=ORIENTED_EDGE('',*,*,#7290,.F.);
#10436=ORIENTED_EDGE('',*,*,#7291,.T.);
#10437=ORIENTED_EDGE('',*,*,#7292,.T.);
#10438=ORIENTED_EDGE('',*,*,#7275,.T.);
#10439=ORIENTED_EDGE('',*,*,#7292,.F.);
#10440=ORIENTED_EDGE('',*,*,#7293,.T.);
#10441=ORIENTED_EDGE('',*,*,#7276,.T.);
#10442=ORIENTED_EDGE('',*,*,#7267,.T.);
#10443=ORIENTED_EDGE('',*,*,#7291,.F.);
#10444=ORIENTED_EDGE('',*,*,#7289,.F.);
#10445=ORIENTED_EDGE('',*,*,#7287,.F.);
#10446=ORIENTED_EDGE('',*,*,#7285,.F.);
#10447=ORIENTED_EDGE('',*,*,#7283,.F.);
#10448=ORIENTED_EDGE('',*,*,#7281,.F.);
#10449=ORIENTED_EDGE('',*,*,#7279,.F.);
#10450=ORIENTED_EDGE('',*,*,#7277,.F.);
#10451=ORIENTED_EDGE('',*,*,#7293,.F.);
#10452=ORIENTED_EDGE('',*,*,#7294,.F.);
#10453=ORIENTED_EDGE('',*,*,#7295,.T.);
#10454=ORIENTED_EDGE('',*,*,#7296,.F.);
#10455=ORIENTED_EDGE('',*,*,#7297,.F.);
#10456=ORIENTED_EDGE('',*,*,#7298,.F.);
#10457=ORIENTED_EDGE('',*,*,#7297,.T.);
#10458=ORIENTED_EDGE('',*,*,#7299,.F.);
#10459=ORIENTED_EDGE('',*,*,#7300,.F.);
#10460=ORIENTED_EDGE('',*,*,#7301,.F.);
#10461=ORIENTED_EDGE('',*,*,#7300,.T.);
#10462=ORIENTED_EDGE('',*,*,#7302,.F.);
#10463=ORIENTED_EDGE('',*,*,#7303,.F.);
#10464=ORIENTED_EDGE('',*,*,#7304,.F.);
#10465=ORIENTED_EDGE('',*,*,#7303,.T.);
#10466=ORIENTED_EDGE('',*,*,#7305,.F.);
#10467=ORIENTED_EDGE('',*,*,#7306,.F.);
#10468=ORIENTED_EDGE('',*,*,#7307,.F.);
#10469=ORIENTED_EDGE('',*,*,#7306,.T.);
#10470=ORIENTED_EDGE('',*,*,#7308,.F.);
#10471=ORIENTED_EDGE('',*,*,#7309,.F.);
#10472=ORIENTED_EDGE('',*,*,#7310,.F.);
#10473=ORIENTED_EDGE('',*,*,#7309,.T.);
#10474=ORIENTED_EDGE('',*,*,#7311,.F.);
#10475=ORIENTED_EDGE('',*,*,#7312,.F.);
#10476=ORIENTED_EDGE('',*,*,#7313,.F.);
#10477=ORIENTED_EDGE('',*,*,#7312,.T.);
#10478=ORIENTED_EDGE('',*,*,#7314,.F.);
#10479=ORIENTED_EDGE('',*,*,#7315,.F.);
#10480=ORIENTED_EDGE('',*,*,#7316,.F.);
#10481=ORIENTED_EDGE('',*,*,#7315,.T.);
#10482=ORIENTED_EDGE('',*,*,#7317,.F.);
#10483=ORIENTED_EDGE('',*,*,#7318,.F.);
#10484=ORIENTED_EDGE('',*,*,#7319,.F.);
#10485=ORIENTED_EDGE('',*,*,#7318,.T.);
#10486=ORIENTED_EDGE('',*,*,#7320,.F.);
#10487=ORIENTED_EDGE('',*,*,#7295,.F.);
#10488=ORIENTED_EDGE('',*,*,#7299,.T.);
#10489=ORIENTED_EDGE('',*,*,#7296,.T.);
#10490=ORIENTED_EDGE('',*,*,#7320,.T.);
#10491=ORIENTED_EDGE('',*,*,#7317,.T.);
#10492=ORIENTED_EDGE('',*,*,#7314,.T.);
#10493=ORIENTED_EDGE('',*,*,#7311,.T.);
#10494=ORIENTED_EDGE('',*,*,#7308,.T.);
#10495=ORIENTED_EDGE('',*,*,#7305,.T.);
#10496=ORIENTED_EDGE('',*,*,#7302,.T.);
#10497=ORIENTED_EDGE('',*,*,#7319,.T.);
#10498=ORIENTED_EDGE('',*,*,#7294,.T.);
#10499=ORIENTED_EDGE('',*,*,#7298,.T.);
#10500=ORIENTED_EDGE('',*,*,#7301,.T.);
#10501=ORIENTED_EDGE('',*,*,#7304,.T.);
#10502=ORIENTED_EDGE('',*,*,#7307,.T.);
#10503=ORIENTED_EDGE('',*,*,#7310,.T.);
#10504=ORIENTED_EDGE('',*,*,#7313,.T.);
#10505=ORIENTED_EDGE('',*,*,#7316,.T.);
#10506=ORIENTED_EDGE('',*,*,#7321,.T.);
#10507=ORIENTED_EDGE('',*,*,#7322,.T.);
#10508=ORIENTED_EDGE('',*,*,#7323,.T.);
#10509=ORIENTED_EDGE('',*,*,#7324,.T.);
#10510=ORIENTED_EDGE('',*,*,#7325,.T.);
#10511=ORIENTED_EDGE('',*,*,#7326,.T.);
#10512=ORIENTED_EDGE('',*,*,#7327,.T.);
#10513=ORIENTED_EDGE('',*,*,#7328,.T.);
#10514=ORIENTED_EDGE('',*,*,#7329,.T.);
#10515=ORIENTED_EDGE('',*,*,#7330,.T.);
#10516=ORIENTED_EDGE('',*,*,#7331,.T.);
#10517=ORIENTED_EDGE('',*,*,#7332,.F.);
#10518=ORIENTED_EDGE('',*,*,#7329,.F.);
#10519=ORIENTED_EDGE('',*,*,#7333,.T.);
#10520=ORIENTED_EDGE('',*,*,#7334,.T.);
#10521=ORIENTED_EDGE('',*,*,#7330,.F.);
#10522=ORIENTED_EDGE('',*,*,#7328,.F.);
#10523=ORIENTED_EDGE('',*,*,#7335,.T.);
#10524=ORIENTED_EDGE('',*,*,#7336,.T.);
#10525=ORIENTED_EDGE('',*,*,#7333,.F.);
#10526=ORIENTED_EDGE('',*,*,#7327,.F.);
#10527=ORIENTED_EDGE('',*,*,#7337,.T.);
#10528=ORIENTED_EDGE('',*,*,#7338,.T.);
#10529=ORIENTED_EDGE('',*,*,#7335,.F.);
#10530=ORIENTED_EDGE('',*,*,#7326,.F.);
#10531=ORIENTED_EDGE('',*,*,#7339,.T.);
#10532=ORIENTED_EDGE('',*,*,#7340,.T.);
#10533=ORIENTED_EDGE('',*,*,#7337,.F.);
#10534=ORIENTED_EDGE('',*,*,#7325,.F.);
#10535=ORIENTED_EDGE('',*,*,#7341,.T.);
#10536=ORIENTED_EDGE('',*,*,#7342,.T.);
#10537=ORIENTED_EDGE('',*,*,#7339,.F.);
#10538=ORIENTED_EDGE('',*,*,#7324,.F.);
#10539=ORIENTED_EDGE('',*,*,#7343,.T.);
#10540=ORIENTED_EDGE('',*,*,#7344,.T.);
#10541=ORIENTED_EDGE('',*,*,#7341,.F.);
#10542=ORIENTED_EDGE('',*,*,#7323,.F.);
#10543=ORIENTED_EDGE('',*,*,#7345,.T.);
#10544=ORIENTED_EDGE('',*,*,#7346,.T.);
#10545=ORIENTED_EDGE('',*,*,#7343,.F.);
#10546=ORIENTED_EDGE('',*,*,#7322,.F.);
#10547=ORIENTED_EDGE('',*,*,#7332,.T.);
#10548=ORIENTED_EDGE('',*,*,#7347,.T.);
#10549=ORIENTED_EDGE('',*,*,#7345,.F.);
#10550=ORIENTED_EDGE('',*,*,#7321,.F.);
#10551=ORIENTED_EDGE('',*,*,#7331,.F.);
#10552=ORIENTED_EDGE('',*,*,#7334,.F.);
#10553=ORIENTED_EDGE('',*,*,#7336,.F.);
#10554=ORIENTED_EDGE('',*,*,#7338,.F.);
#10555=ORIENTED_EDGE('',*,*,#7340,.F.);
#10556=ORIENTED_EDGE('',*,*,#7342,.F.);
#10557=ORIENTED_EDGE('',*,*,#7344,.F.);
#10558=ORIENTED_EDGE('',*,*,#7346,.F.);
#10559=ORIENTED_EDGE('',*,*,#7347,.F.);
#10560=ORIENTED_EDGE('',*,*,#7348,.F.);
#10561=ORIENTED_EDGE('',*,*,#7349,.T.);
#10562=ORIENTED_EDGE('',*,*,#7350,.T.);
#10563=ORIENTED_EDGE('',*,*,#7351,.F.);
#10564=ORIENTED_EDGE('',*,*,#7352,.F.);
#10565=ORIENTED_EDGE('',*,*,#7353,.T.);
#10566=ORIENTED_EDGE('',*,*,#7354,.T.);
#10567=ORIENTED_EDGE('',*,*,#7355,.F.);
#10568=ORIENTED_EDGE('',*,*,#7356,.F.);
#10569=ORIENTED_EDGE('',*,*,#7357,.T.);
#10570=ORIENTED_EDGE('',*,*,#7358,.T.);
#10571=ORIENTED_EDGE('',*,*,#7359,.F.);
#10572=ORIENTED_EDGE('',*,*,#7360,.F.);
#10573=ORIENTED_EDGE('',*,*,#7361,.T.);
#10574=ORIENTED_EDGE('',*,*,#7362,.T.);
#10575=ORIENTED_EDGE('',*,*,#7363,.F.);
#10576=ORIENTED_EDGE('',*,*,#7364,.T.);
#10577=ORIENTED_EDGE('',*,*,#7365,.T.);
#10578=ORIENTED_EDGE('',*,*,#7366,.F.);
#10579=ORIENTED_EDGE('',*,*,#7367,.T.);
#10580=ORIENTED_EDGE('',*,*,#7368,.F.);
#10581=ORIENTED_EDGE('',*,*,#7369,.T.);
#10582=ORIENTED_EDGE('',*,*,#7370,.T.);
#10583=ORIENTED_EDGE('',*,*,#7371,.T.);
#10584=ORIENTED_EDGE('',*,*,#7372,.T.);
#10585=ORIENTED_EDGE('',*,*,#7373,.T.);
#10586=ORIENTED_EDGE('',*,*,#7374,.F.);
#10587=ORIENTED_EDGE('',*,*,#7375,.T.);
#10588=ORIENTED_EDGE('',*,*,#7376,.T.);
#10589=ORIENTED_EDGE('',*,*,#7377,.T.);
#10590=ORIENTED_EDGE('',*,*,#7378,.F.);
#10591=ORIENTED_EDGE('',*,*,#7379,.T.);
#10592=ORIENTED_EDGE('',*,*,#7366,.T.);
#10593=ORIENTED_EDGE('',*,*,#7380,.T.);
#10594=ORIENTED_EDGE('',*,*,#7368,.T.);
#10595=ORIENTED_EDGE('',*,*,#7381,.T.);
#10596=ORIENTED_EDGE('',*,*,#7374,.T.);
#10597=ORIENTED_EDGE('',*,*,#7382,.T.);
#10598=ORIENTED_EDGE('',*,*,#7378,.T.);
#10599=ORIENTED_EDGE('',*,*,#7383,.T.);
#10600=ORIENTED_EDGE('',*,*,#7384,.F.);
#10601=ORIENTED_EDGE('',*,*,#7350,.F.);
#10602=ORIENTED_EDGE('',*,*,#7385,.F.);
#10603=ORIENTED_EDGE('',*,*,#7386,.F.);
#10604=ORIENTED_EDGE('',*,*,#7387,.F.);
#10605=ORIENTED_EDGE('',*,*,#7354,.F.);
#10606=ORIENTED_EDGE('',*,*,#7388,.F.);
#10607=ORIENTED_EDGE('',*,*,#7389,.F.);
#10608=ORIENTED_EDGE('',*,*,#7390,.F.);
#10609=ORIENTED_EDGE('',*,*,#7358,.F.);
#10610=ORIENTED_EDGE('',*,*,#7391,.F.);
#10611=ORIENTED_EDGE('',*,*,#7392,.F.);
#10612=ORIENTED_EDGE('',*,*,#7393,.F.);
#10613=ORIENTED_EDGE('',*,*,#7362,.F.);
#10614=ORIENTED_EDGE('',*,*,#7394,.F.);
#10615=ORIENTED_EDGE('',*,*,#7395,.F.);
#10616=ORIENTED_EDGE('',*,*,#7370,.F.);
#10617=ORIENTED_EDGE('',*,*,#7396,.T.);
#10618=ORIENTED_EDGE('',*,*,#7364,.F.);
#10619=ORIENTED_EDGE('',*,*,#7397,.T.);
#10620=ORIENTED_EDGE('',*,*,#7376,.F.);
#10621=ORIENTED_EDGE('',*,*,#7398,.T.);
#10622=ORIENTED_EDGE('',*,*,#7372,.F.);
#10623=ORIENTED_EDGE('',*,*,#7399,.T.);
#10624=ORIENTED_EDGE('',*,*,#7348,.T.);
#10625=ORIENTED_EDGE('',*,*,#7400,.T.);
#10626=ORIENTED_EDGE('',*,*,#7401,.T.);
#10627=ORIENTED_EDGE('',*,*,#7402,.T.);
#10628=ORIENTED_EDGE('',*,*,#7352,.T.);
#10629=ORIENTED_EDGE('',*,*,#7403,.T.);
#10630=ORIENTED_EDGE('',*,*,#7404,.T.);
#10631=ORIENTED_EDGE('',*,*,#7405,.T.);
#10632=ORIENTED_EDGE('',*,*,#7356,.T.);
#10633=ORIENTED_EDGE('',*,*,#7406,.T.);
#10634=ORIENTED_EDGE('',*,*,#7407,.T.);
#10635=ORIENTED_EDGE('',*,*,#7408,.T.);
#10636=ORIENTED_EDGE('',*,*,#7360,.T.);
#10637=ORIENTED_EDGE('',*,*,#7409,.T.);
#10638=ORIENTED_EDGE('',*,*,#7410,.T.);
#10639=ORIENTED_EDGE('',*,*,#7411,.T.);
#10640=ORIENTED_EDGE('',*,*,#7394,.T.);
#10641=ORIENTED_EDGE('',*,*,#7361,.F.);
#10642=ORIENTED_EDGE('',*,*,#7411,.F.);
#10643=ORIENTED_EDGE('',*,*,#7412,.T.);
#10644=ORIENTED_EDGE('',*,*,#7395,.T.);
#10645=ORIENTED_EDGE('',*,*,#7412,.F.);
#10646=ORIENTED_EDGE('',*,*,#7410,.F.);
#10647=ORIENTED_EDGE('',*,*,#7413,.T.);
#10648=ORIENTED_EDGE('',*,*,#7393,.T.);
#10649=ORIENTED_EDGE('',*,*,#7413,.F.);
#10650=ORIENTED_EDGE('',*,*,#7409,.F.);
#10651=ORIENTED_EDGE('',*,*,#7363,.T.);
#10652=ORIENTED_EDGE('',*,*,#7391,.T.);
#10653=ORIENTED_EDGE('',*,*,#7357,.F.);
#10654=ORIENTED_EDGE('',*,*,#7408,.F.);
#10655=ORIENTED_EDGE('',*,*,#7414,.T.);
#10656=ORIENTED_EDGE('',*,*,#7392,.T.);
#10657=ORIENTED_EDGE('',*,*,#7414,.F.);
#10658=ORIENTED_EDGE('',*,*,#7407,.F.);
#10659=ORIENTED_EDGE('',*,*,#7415,.T.);
#10660=ORIENTED_EDGE('',*,*,#7390,.T.);
#10661=ORIENTED_EDGE('',*,*,#7415,.F.);
#10662=ORIENTED_EDGE('',*,*,#7406,.F.);
#10663=ORIENTED_EDGE('',*,*,#7359,.T.);
#10664=ORIENTED_EDGE('',*,*,#7388,.T.);
#10665=ORIENTED_EDGE('',*,*,#7353,.F.);
#10666=ORIENTED_EDGE('',*,*,#7405,.F.);
#10667=ORIENTED_EDGE('',*,*,#7416,.T.);
#10668=ORIENTED_EDGE('',*,*,#7389,.T.);
#10669=ORIENTED_EDGE('',*,*,#7416,.F.);
#10670=ORIENTED_EDGE('',*,*,#7404,.F.);
#10671=ORIENTED_EDGE('',*,*,#7417,.T.);
#10672=ORIENTED_EDGE('',*,*,#7387,.T.);
#10673=ORIENTED_EDGE('',*,*,#7417,.F.);
#10674=ORIENTED_EDGE('',*,*,#7403,.F.);
#10675=ORIENTED_EDGE('',*,*,#7355,.T.);
#10676=ORIENTED_EDGE('',*,*,#7385,.T.);
#10677=ORIENTED_EDGE('',*,*,#7349,.F.);
#10678=ORIENTED_EDGE('',*,*,#7402,.F.);
#10679=ORIENTED_EDGE('',*,*,#7418,.T.);
#10680=ORIENTED_EDGE('',*,*,#7386,.T.);
#10681=ORIENTED_EDGE('',*,*,#7418,.F.);
#10682=ORIENTED_EDGE('',*,*,#7401,.F.);
#10683=ORIENTED_EDGE('',*,*,#7419,.T.);
#10684=ORIENTED_EDGE('',*,*,#7384,.T.);
#10685=ORIENTED_EDGE('',*,*,#7419,.F.);
#10686=ORIENTED_EDGE('',*,*,#7400,.F.);
#10687=ORIENTED_EDGE('',*,*,#7351,.T.);
#10688=ORIENTED_EDGE('',*,*,#7380,.F.);
#10689=ORIENTED_EDGE('',*,*,#7365,.F.);
#10690=ORIENTED_EDGE('',*,*,#7396,.F.);
#10691=ORIENTED_EDGE('',*,*,#7369,.F.);
#10692=ORIENTED_EDGE('',*,*,#7383,.F.);
#10693=ORIENTED_EDGE('',*,*,#7377,.F.);
#10694=ORIENTED_EDGE('',*,*,#7397,.F.);
#10695=ORIENTED_EDGE('',*,*,#7367,.F.);
#10696=ORIENTED_EDGE('',*,*,#7382,.F.);
#10697=ORIENTED_EDGE('',*,*,#7373,.F.);
#10698=ORIENTED_EDGE('',*,*,#7398,.F.);
#10699=ORIENTED_EDGE('',*,*,#7379,.F.);
#10700=ORIENTED_EDGE('',*,*,#7381,.F.);
#10701=ORIENTED_EDGE('',*,*,#7371,.F.);
#10702=ORIENTED_EDGE('',*,*,#7399,.F.);
#10703=ORIENTED_EDGE('',*,*,#7375,.F.);
#10704=ORIENTED_EDGE('',*,*,#7420,.F.);
#10705=ORIENTED_EDGE('',*,*,#7421,.T.);
#10706=ORIENTED_EDGE('',*,*,#7422,.T.);
#10707=ORIENTED_EDGE('',*,*,#7421,.F.);
#10708=ORIENTED_EDGE('',*,*,#7423,.F.);
#10709=ORIENTED_EDGE('',*,*,#7424,.T.);
#10710=ORIENTED_EDGE('',*,*,#7425,.T.);
#10711=ORIENTED_EDGE('',*,*,#7424,.F.);
#10712=ORIENTED_EDGE('',*,*,#7426,.F.);
#10713=ORIENTED_EDGE('',*,*,#7427,.F.);
#10714=ORIENTED_EDGE('',*,*,#7428,.F.);
#10715=ORIENTED_EDGE('',*,*,#7429,.T.);
#10716=ORIENTED_EDGE('',*,*,#7430,.F.);
#10717=ORIENTED_EDGE('',*,*,#7431,.F.);
#10718=ORIENTED_EDGE('',*,*,#7432,.F.);
#10719=ORIENTED_EDGE('',*,*,#7427,.T.);
#10720=ORIENTED_EDGE('',*,*,#7433,.F.);
#10721=ORIENTED_EDGE('',*,*,#7434,.F.);
#10722=ORIENTED_EDGE('',*,*,#7435,.F.);
#10723=ORIENTED_EDGE('',*,*,#7431,.T.);
#10724=ORIENTED_EDGE('',*,*,#7436,.F.);
#10725=ORIENTED_EDGE('',*,*,#7437,.F.);
#10726=ORIENTED_EDGE('',*,*,#7438,.F.);
#10727=ORIENTED_EDGE('',*,*,#7434,.T.);
#10728=ORIENTED_EDGE('',*,*,#7439,.F.);
#10729=ORIENTED_EDGE('',*,*,#7440,.F.);
#10730=ORIENTED_EDGE('',*,*,#7441,.F.);
#10731=ORIENTED_EDGE('',*,*,#7437,.T.);
#10732=ORIENTED_EDGE('',*,*,#7442,.F.);
#10733=ORIENTED_EDGE('',*,*,#7443,.F.);
#10734=ORIENTED_EDGE('',*,*,#7444,.F.);
#10735=ORIENTED_EDGE('',*,*,#7440,.T.);
#10736=ORIENTED_EDGE('',*,*,#7420,.T.);
#10737=ORIENTED_EDGE('',*,*,#7423,.T.);
#10738=ORIENTED_EDGE('',*,*,#7445,.F.);
#10739=ORIENTED_EDGE('',*,*,#7446,.F.);
#10740=ORIENTED_EDGE('',*,*,#7447,.F.);
#10741=ORIENTED_EDGE('',*,*,#7443,.T.);
#10742=ORIENTED_EDGE('',*,*,#7448,.F.);
#10743=ORIENTED_EDGE('',*,*,#7449,.F.);
#10744=ORIENTED_EDGE('',*,*,#7450,.F.);
#10745=ORIENTED_EDGE('',*,*,#7446,.T.);
#10746=ORIENTED_EDGE('',*,*,#7451,.F.);
#10747=ORIENTED_EDGE('',*,*,#7452,.F.);
#10748=ORIENTED_EDGE('',*,*,#7453,.F.);
#10749=ORIENTED_EDGE('',*,*,#7449,.T.);
#10750=ORIENTED_EDGE('',*,*,#7454,.F.);
#10751=ORIENTED_EDGE('',*,*,#7455,.F.);
#10752=ORIENTED_EDGE('',*,*,#7456,.F.);
#10753=ORIENTED_EDGE('',*,*,#7452,.T.);
#10754=ORIENTED_EDGE('',*,*,#7457,.F.);
#10755=ORIENTED_EDGE('',*,*,#7458,.F.);
#10756=ORIENTED_EDGE('',*,*,#7459,.F.);
#10757=ORIENTED_EDGE('',*,*,#7455,.T.);
#10758=ORIENTED_EDGE('',*,*,#7460,.F.);
#10759=ORIENTED_EDGE('',*,*,#7429,.F.);
#10760=ORIENTED_EDGE('',*,*,#7461,.F.);
#10761=ORIENTED_EDGE('',*,*,#7458,.T.);
#10762=ORIENTED_EDGE('',*,*,#7422,.F.);
#10763=ORIENTED_EDGE('',*,*,#7425,.F.);
#10764=ORIENTED_EDGE('',*,*,#7461,.T.);
#10765=ORIENTED_EDGE('',*,*,#7428,.T.);
#10766=ORIENTED_EDGE('',*,*,#7432,.T.);
#10767=ORIENTED_EDGE('',*,*,#7435,.T.);
#10768=ORIENTED_EDGE('',*,*,#7438,.T.);
#10769=ORIENTED_EDGE('',*,*,#7441,.T.);
#10770=ORIENTED_EDGE('',*,*,#7444,.T.);
#10771=ORIENTED_EDGE('',*,*,#7447,.T.);
#10772=ORIENTED_EDGE('',*,*,#7450,.T.);
#10773=ORIENTED_EDGE('',*,*,#7453,.T.);
#10774=ORIENTED_EDGE('',*,*,#7456,.T.);
#10775=ORIENTED_EDGE('',*,*,#7459,.T.);
#10776=ORIENTED_EDGE('',*,*,#7430,.T.);
#10777=ORIENTED_EDGE('',*,*,#7426,.T.);
#10778=ORIENTED_EDGE('',*,*,#7460,.T.);
#10779=ORIENTED_EDGE('',*,*,#7457,.T.);
#10780=ORIENTED_EDGE('',*,*,#7454,.T.);
#10781=ORIENTED_EDGE('',*,*,#7451,.T.);
#10782=ORIENTED_EDGE('',*,*,#7448,.T.);
#10783=ORIENTED_EDGE('',*,*,#7445,.T.);
#10784=ORIENTED_EDGE('',*,*,#7442,.T.);
#10785=ORIENTED_EDGE('',*,*,#7439,.T.);
#10786=ORIENTED_EDGE('',*,*,#7436,.T.);
#10787=ORIENTED_EDGE('',*,*,#7433,.T.);
#10788=ORIENTED_EDGE('',*,*,#7462,.F.);
#10789=ORIENTED_EDGE('',*,*,#7463,.T.);
#10790=ORIENTED_EDGE('',*,*,#7464,.T.);
#10791=ORIENTED_EDGE('',*,*,#7463,.F.);
#10792=ORIENTED_EDGE('',*,*,#7465,.F.);
#10793=ORIENTED_EDGE('',*,*,#7466,.T.);
#10794=ORIENTED_EDGE('',*,*,#7467,.T.);
#10795=ORIENTED_EDGE('',*,*,#7466,.F.);
#10796=ORIENTED_EDGE('',*,*,#7468,.T.);
#10797=ORIENTED_EDGE('',*,*,#7469,.F.);
#10798=ORIENTED_EDGE('',*,*,#7470,.F.);
#10799=ORIENTED_EDGE('',*,*,#7471,.T.);
#10800=ORIENTED_EDGE('',*,*,#7464,.F.);
#10801=ORIENTED_EDGE('',*,*,#7467,.F.);
#10802=ORIENTED_EDGE('',*,*,#7472,.T.);
#10803=ORIENTED_EDGE('',*,*,#7473,.F.);
#10804=ORIENTED_EDGE('',*,*,#7474,.F.);
#10805=ORIENTED_EDGE('',*,*,#7469,.T.);
#10806=ORIENTED_EDGE('',*,*,#7475,.T.);
#10807=ORIENTED_EDGE('',*,*,#7476,.F.);
#10808=ORIENTED_EDGE('',*,*,#7477,.F.);
#10809=ORIENTED_EDGE('',*,*,#7473,.T.);
#10810=ORIENTED_EDGE('',*,*,#7478,.T.);
#10811=ORIENTED_EDGE('',*,*,#7479,.F.);
#10812=ORIENTED_EDGE('',*,*,#7480,.F.);
#10813=ORIENTED_EDGE('',*,*,#7476,.T.);
#10814=ORIENTED_EDGE('',*,*,#7462,.T.);
#10815=ORIENTED_EDGE('',*,*,#7465,.T.);
#10816=ORIENTED_EDGE('',*,*,#7481,.T.);
#10817=ORIENTED_EDGE('',*,*,#7482,.F.);
#10818=ORIENTED_EDGE('',*,*,#7483,.F.);
#10819=ORIENTED_EDGE('',*,*,#7479,.T.);
#10820=ORIENTED_EDGE('',*,*,#7484,.T.);
#10821=ORIENTED_EDGE('',*,*,#7485,.F.);
#10822=ORIENTED_EDGE('',*,*,#7486,.F.);
#10823=ORIENTED_EDGE('',*,*,#7482,.T.);
#10824=ORIENTED_EDGE('',*,*,#7487,.T.);
#10825=ORIENTED_EDGE('',*,*,#7488,.F.);
#10826=ORIENTED_EDGE('',*,*,#7489,.F.);
#10827=ORIENTED_EDGE('',*,*,#7485,.T.);
#10828=ORIENTED_EDGE('',*,*,#7490,.T.);
#10829=ORIENTED_EDGE('',*,*,#7491,.F.);
#10830=ORIENTED_EDGE('',*,*,#7492,.F.);
#10831=ORIENTED_EDGE('',*,*,#7488,.T.);
#10832=ORIENTED_EDGE('',*,*,#7493,.T.);
#10833=ORIENTED_EDGE('',*,*,#7471,.F.);
#10834=ORIENTED_EDGE('',*,*,#7494,.F.);
#10835=ORIENTED_EDGE('',*,*,#7491,.T.);
#10836=ORIENTED_EDGE('',*,*,#7470,.T.);
#10837=ORIENTED_EDGE('',*,*,#7474,.T.);
#10838=ORIENTED_EDGE('',*,*,#7477,.T.);
#10839=ORIENTED_EDGE('',*,*,#7480,.T.);
#10840=ORIENTED_EDGE('',*,*,#7483,.T.);
#10841=ORIENTED_EDGE('',*,*,#7486,.T.);
#10842=ORIENTED_EDGE('',*,*,#7489,.T.);
#10843=ORIENTED_EDGE('',*,*,#7492,.T.);
#10844=ORIENTED_EDGE('',*,*,#7494,.T.);
#10845=ORIENTED_EDGE('',*,*,#7468,.F.);
#10846=ORIENTED_EDGE('',*,*,#7493,.F.);
#10847=ORIENTED_EDGE('',*,*,#7490,.F.);
#10848=ORIENTED_EDGE('',*,*,#7487,.F.);
#10849=ORIENTED_EDGE('',*,*,#7484,.F.);
#10850=ORIENTED_EDGE('',*,*,#7481,.F.);
#10851=ORIENTED_EDGE('',*,*,#7478,.F.);
#10852=ORIENTED_EDGE('',*,*,#7475,.F.);
#10853=ORIENTED_EDGE('',*,*,#7472,.F.);
#10854=ORIENTED_EDGE('',*,*,#7495,.F.);
#10855=ORIENTED_EDGE('',*,*,#7496,.T.);
#10856=ORIENTED_EDGE('',*,*,#7497,.T.);
#10857=ORIENTED_EDGE('',*,*,#7496,.F.);
#10858=ORIENTED_EDGE('',*,*,#7498,.F.);
#10859=ORIENTED_EDGE('',*,*,#7499,.T.);
#10860=ORIENTED_EDGE('',*,*,#7500,.T.);
#10861=ORIENTED_EDGE('',*,*,#7499,.F.);
#10862=ORIENTED_EDGE('',*,*,#7501,.F.);
#10863=ORIENTED_EDGE('',*,*,#7502,.F.);
#10864=ORIENTED_EDGE('',*,*,#7503,.T.);
#10865=ORIENTED_EDGE('',*,*,#7504,.T.);
#10866=ORIENTED_EDGE('',*,*,#7497,.F.);
#10867=ORIENTED_EDGE('',*,*,#7500,.F.);
#10868=ORIENTED_EDGE('',*,*,#7505,.F.);
#10869=ORIENTED_EDGE('',*,*,#7504,.F.);
#10870=ORIENTED_EDGE('',*,*,#7506,.T.);
#10871=ORIENTED_EDGE('',*,*,#7507,.T.);
#10872=ORIENTED_EDGE('',*,*,#7508,.F.);
#10873=ORIENTED_EDGE('',*,*,#7507,.F.);
#10874=ORIENTED_EDGE('',*,*,#7509,.T.);
#10875=ORIENTED_EDGE('',*,*,#7510,.T.);
#10876=ORIENTED_EDGE('',*,*,#7511,.F.);
#10877=ORIENTED_EDGE('',*,*,#7510,.F.);
#10878=ORIENTED_EDGE('',*,*,#7512,.T.);
#10879=ORIENTED_EDGE('',*,*,#7513,.T.);
#10880=ORIENTED_EDGE('',*,*,#7495,.T.);
#10881=ORIENTED_EDGE('',*,*,#7498,.T.);
#10882=ORIENTED_EDGE('',*,*,#7514,.F.);
#10883=ORIENTED_EDGE('',*,*,#7513,.F.);
#10884=ORIENTED_EDGE('',*,*,#7515,.T.);
#10885=ORIENTED_EDGE('',*,*,#7516,.T.);
#10886=ORIENTED_EDGE('',*,*,#7517,.F.);
#10887=ORIENTED_EDGE('',*,*,#7516,.F.);
#10888=ORIENTED_EDGE('',*,*,#7518,.T.);
#10889=ORIENTED_EDGE('',*,*,#7519,.T.);
#10890=ORIENTED_EDGE('',*,*,#7520,.F.);
#10891=ORIENTED_EDGE('',*,*,#7519,.F.);
#10892=ORIENTED_EDGE('',*,*,#7521,.T.);
#10893=ORIENTED_EDGE('',*,*,#7522,.T.);
#10894=ORIENTED_EDGE('',*,*,#7523,.F.);
#10895=ORIENTED_EDGE('',*,*,#7522,.F.);
#10896=ORIENTED_EDGE('',*,*,#7524,.T.);
#10897=ORIENTED_EDGE('',*,*,#7525,.T.);
#10898=ORIENTED_EDGE('',*,*,#7526,.F.);
#10899=ORIENTED_EDGE('',*,*,#7525,.F.);
#10900=ORIENTED_EDGE('',*,*,#7527,.T.);
#10901=ORIENTED_EDGE('',*,*,#7502,.T.);
#10902=ORIENTED_EDGE('',*,*,#7503,.F.);
#10903=ORIENTED_EDGE('',*,*,#7527,.F.);
#10904=ORIENTED_EDGE('',*,*,#7524,.F.);
#10905=ORIENTED_EDGE('',*,*,#7521,.F.);
#10906=ORIENTED_EDGE('',*,*,#7518,.F.);
#10907=ORIENTED_EDGE('',*,*,#7515,.F.);
#10908=ORIENTED_EDGE('',*,*,#7512,.F.);
#10909=ORIENTED_EDGE('',*,*,#7509,.F.);
#10910=ORIENTED_EDGE('',*,*,#7506,.F.);
#10911=ORIENTED_EDGE('',*,*,#7501,.T.);
#10912=ORIENTED_EDGE('',*,*,#7505,.T.);
#10913=ORIENTED_EDGE('',*,*,#7508,.T.);
#10914=ORIENTED_EDGE('',*,*,#7511,.T.);
#10915=ORIENTED_EDGE('',*,*,#7514,.T.);
#10916=ORIENTED_EDGE('',*,*,#7517,.T.);
#10917=ORIENTED_EDGE('',*,*,#7520,.T.);
#10918=ORIENTED_EDGE('',*,*,#7523,.T.);
#10919=ORIENTED_EDGE('',*,*,#7526,.T.);
#11048=CYLINDRICAL_SURFACE('',#12669,2.54);
#11049=CYLINDRICAL_SURFACE('',#12673,6.85800000000002);
#11050=CYLINDRICAL_SURFACE('',#12677,6.85800000000002);
#11051=CYLINDRICAL_SURFACE('',#12681,2.54);
#11052=CYLINDRICAL_SURFACE('',#12697,2.53999999999999);
#11053=CYLINDRICAL_SURFACE('',#12700,6.85800000000003);
#11054=CYLINDRICAL_SURFACE('',#12703,6.85800000000003);
#11055=CYLINDRICAL_SURFACE('',#12706,2.53999999999999);
#11056=CYLINDRICAL_SURFACE('',#12719,2.53999999999998);
#11057=CYLINDRICAL_SURFACE('',#12722,6.85800000000001);
#11058=CYLINDRICAL_SURFACE('',#12725,6.858);
#11059=CYLINDRICAL_SURFACE('',#12728,2.53999999999998);
#11060=CYLINDRICAL_SURFACE('',#12735,2.53999999999999);
#11061=CYLINDRICAL_SURFACE('',#12739,6.858);
#11062=CYLINDRICAL_SURFACE('',#12743,6.85800000000002);
#11063=CYLINDRICAL_SURFACE('',#12747,2.53999999999999);
#11064=CYLINDRICAL_SURFACE('',#12757,2.53999999999999);
#11065=CYLINDRICAL_SURFACE('',#12761,6.85799999999992);
#11066=CYLINDRICAL_SURFACE('',#12765,6.85799999999992);
#11067=CYLINDRICAL_SURFACE('',#12769,2.53999999999999);
#11068=CYLINDRICAL_SURFACE('',#12785,2.53999999999999);
#11069=CYLINDRICAL_SURFACE('',#12788,6.85800000000003);
#11070=CYLINDRICAL_SURFACE('',#12791,6.85800000000003);
#11071=CYLINDRICAL_SURFACE('',#12794,2.53999999999999);
#11072=CYLINDRICAL_SURFACE('',#12801,2.53999999999999);
#11073=CYLINDRICAL_SURFACE('',#12805,6.85800000000003);
#11074=CYLINDRICAL_SURFACE('',#12809,6.85800000000003);
#11075=CYLINDRICAL_SURFACE('',#12813,2.53999999999999);
#11076=CYLINDRICAL_SURFACE('',#12829,2.53999999999998);
#11077=CYLINDRICAL_SURFACE('',#12832,6.85800000000003);
#11078=CYLINDRICAL_SURFACE('',#12835,6.85800000000003);
#11079=CYLINDRICAL_SURFACE('',#12838,2.53999999999998);
#11080=CYLINDRICAL_SURFACE('',#12851,2.53999999999999);
#11081=CYLINDRICAL_SURFACE('',#12854,6.858);
#11082=CYLINDRICAL_SURFACE('',#12857,6.85800000000003);
#11083=CYLINDRICAL_SURFACE('',#12860,2.53999999999999);
#11084=CYLINDRICAL_SURFACE('',#12873,2.53999999999999);
#11085=CYLINDRICAL_SURFACE('',#12876,6.858);
#11086=CYLINDRICAL_SURFACE('',#12879,6.85800000000003);
#11087=CYLINDRICAL_SURFACE('',#12882,2.53999999999999);
#11088=CYLINDRICAL_SURFACE('',#12889,3.16991999999999);
#11089=CYLINDRICAL_SURFACE('',#12893,4.7625);
#11090=CYLINDRICAL_SURFACE('',#12897,3.16991999999999);
#11091=CYLINDRICAL_SURFACE('',#12906,3.16991999999999);
#11092=CYLINDRICAL_SURFACE('',#12910,4.7625);
#11093=CYLINDRICAL_SURFACE('',#12914,3.16991999999999);
#11094=CYLINDRICAL_SURFACE('',#12923,3.16991999999999);
#11095=CYLINDRICAL_SURFACE('',#12927,4.7625);
#11096=CYLINDRICAL_SURFACE('',#12931,3.16991999999999);
#11097=CYLINDRICAL_SURFACE('',#12940,3.16991999999999);
#11098=CYLINDRICAL_SURFACE('',#12944,4.7625);
#11099=CYLINDRICAL_SURFACE('',#12948,3.16991999999999);
#11100=CYLINDRICAL_SURFACE('',#12961,3.16991999999998);
#11101=CYLINDRICAL_SURFACE('',#12964,4.7625);
#11102=CYLINDRICAL_SURFACE('',#12967,3.16991999999999);
#11103=CYLINDRICAL_SURFACE('',#12974,3.16991999999999);
#11104=CYLINDRICAL_SURFACE('',#12978,4.7625);
#11105=CYLINDRICAL_SURFACE('',#12982,3.16991999999999);
#11106=CYLINDRICAL_SURFACE('',#12995,3.16991999999996);
#11107=CYLINDRICAL_SURFACE('',#12998,4.7625);
#11108=CYLINDRICAL_SURFACE('',#13001,3.16991999999999);
#11109=CYLINDRICAL_SURFACE('',#13012,3.16991999999996);
#11110=CYLINDRICAL_SURFACE('',#13015,4.7625);
#11111=CYLINDRICAL_SURFACE('',#13018,3.16991999999999);
#11112=CYLINDRICAL_SURFACE('',#13025,3.16992000000005);
#11113=CYLINDRICAL_SURFACE('',#13029,4.7625);
#11114=CYLINDRICAL_SURFACE('',#13033,3.16991999999994);
#11115=CYLINDRICAL_SURFACE('',#13046,3.16991999999994);
#11116=CYLINDRICAL_SURFACE('',#13049,4.7625);
#11117=CYLINDRICAL_SURFACE('',#13052,3.16992000000005);
#11118=CYLINDRICAL_SURFACE('',#13057,4.50000000000006);
#11119=CYLINDRICAL_SURFACE('',#13060,4.49999999999995);
#11120=CYLINDRICAL_SURFACE('',#13063,4.49999999999995);
#11121=CYLINDRICAL_SURFACE('',#13066,4.49999999999995);
#11122=CYLINDRICAL_SURFACE('',#13084,4.49999999999995);
#11123=CYLINDRICAL_SURFACE('',#13087,4.49999999999995);
#11124=CYLINDRICAL_SURFACE('',#13090,4.49999999999995);
#11125=CYLINDRICAL_SURFACE('',#13093,4.50000000000006);
#11126=CYLINDRICAL_SURFACE('',#13099,8.74999999999998);
#11127=CYLINDRICAL_SURFACE('',#13102,8.74999999999998);
#11128=CYLINDRICAL_SURFACE('',#13107,2.53999999999999);
#11129=CYLINDRICAL_SURFACE('',#13111,6.85800000000003);
#11130=CYLINDRICAL_SURFACE('',#13115,6.85799999999998);
#11131=CYLINDRICAL_SURFACE('',#13119,2.53999999999999);
#11132=CYLINDRICAL_SURFACE('',#13127,4.5);
#11133=CYLINDRICAL_SURFACE('',#13130,4.5);
#11134=CYLINDRICAL_SURFACE('',#13135,3.16991999999999);
#11135=CYLINDRICAL_SURFACE('',#13139,4.7625);
#11136=CYLINDRICAL_SURFACE('',#13143,3.16991999999999);
#11137=CYLINDRICAL_SURFACE('',#13150,4.5);
#11138=CYLINDRICAL_SURFACE('',#13153,4.5);
#11139=CYLINDRICAL_SURFACE('',#13158,3.16991999999999);
#11140=CYLINDRICAL_SURFACE('',#13162,4.7625);
#11141=CYLINDRICAL_SURFACE('',#13166,3.16991999999999);
#11505=ADVANCED_FACE('',(#1066),#318,.F.);
#11506=ADVANCED_FACE('',(#1067),#319,.F.);
#11507=ADVANCED_FACE('',(#1068),#11048,.T.);
#11508=ADVANCED_FACE('',(#1069),#320,.F.);
#11509=ADVANCED_FACE('',(#1070),#11049,.F.);
#11510=ADVANCED_FACE('',(#1071),#321,.F.);
#11511=ADVANCED_FACE('',(#1072),#11050,.F.);
#11512=ADVANCED_FACE('',(#1073),#322,.F.);
#11513=ADVANCED_FACE('',(#1074),#11051,.T.);
#11514=ADVANCED_FACE('',(#1075),#323,.F.);
#11515=ADVANCED_FACE('',(#1076),#324,.F.);
#11516=ADVANCED_FACE('',(#1077),#325,.F.);
#11517=ADVANCED_FACE('',(#1078),#326,.T.);
#11518=ADVANCED_FACE('',(#1079),#327,.T.);
#11519=ADVANCED_FACE('',(#1080),#328,.T.);
#11520=ADVANCED_FACE('',(#1081),#329,.F.);
#11521=ADVANCED_FACE('',(#1082),#330,.F.);
#11522=ADVANCED_FACE('',(#1083),#331,.F.);
#11523=ADVANCED_FACE('',(#1084),#11052,.T.);
#11524=ADVANCED_FACE('',(#1085),#332,.F.);
#11525=ADVANCED_FACE('',(#1086),#11053,.F.);
#11526=ADVANCED_FACE('',(#1087),#333,.F.);
#11527=ADVANCED_FACE('',(#1088),#11054,.F.);
#11528=ADVANCED_FACE('',(#1089),#334,.F.);
#11529=ADVANCED_FACE('',(#1090),#11055,.T.);
#11530=ADVANCED_FACE('',(#1091),#335,.F.);
#11531=ADVANCED_FACE('',(#1092),#336,.F.);
#11532=ADVANCED_FACE('',(#1093),#337,.F.);
#11533=ADVANCED_FACE('',(#1094),#338,.T.);
#11534=ADVANCED_FACE('',(#1095),#339,.F.);
#11535=ADVANCED_FACE('',(#1096),#340,.F.);
#11536=ADVANCED_FACE('',(#1097),#341,.F.);
#11537=ADVANCED_FACE('',(#1098),#11056,.T.);
#11538=ADVANCED_FACE('',(#1099),#342,.F.);
#11539=ADVANCED_FACE('',(#1100),#11057,.F.);
#11540=ADVANCED_FACE('',(#1101),#343,.F.);
#11541=ADVANCED_FACE('',(#1102),#11058,.F.);
#11542=ADVANCED_FACE('',(#1103),#344,.F.);
#11543=ADVANCED_FACE('',(#1104),#11059,.T.);
#11544=ADVANCED_FACE('',(#1105),#345,.F.);
#11545=ADVANCED_FACE('',(#1106),#346,.F.);
#11546=ADVANCED_FACE('',(#1107),#347,.F.);
#11547=ADVANCED_FACE('',(#1108),#348,.F.);
#11548=ADVANCED_FACE('',(#1109),#349,.F.);
#11549=ADVANCED_FACE('',(#1110),#11060,.T.);
#11550=ADVANCED_FACE('',(#1111),#350,.F.);
#11551=ADVANCED_FACE('',(#1112),#11061,.F.);
#11552=ADVANCED_FACE('',(#1113),#351,.F.);
#11553=ADVANCED_FACE('',(#1114),#11062,.F.);
#11554=ADVANCED_FACE('',(#1115),#352,.F.);
#11555=ADVANCED_FACE('',(#1116),#11063,.T.);
#11556=ADVANCED_FACE('',(#1117),#353,.F.);
#11557=ADVANCED_FACE('',(#1118),#354,.F.);
#11558=ADVANCED_FACE('',(#1119),#355,.F.);
#11559=ADVANCED_FACE('',(#1120),#356,.T.);
#11560=ADVANCED_FACE('',(#1121),#357,.T.);
#11561=ADVANCED_FACE('',(#1122),#358,.F.);
#11562=ADVANCED_FACE('',(#1123),#359,.F.);
#11563=ADVANCED_FACE('',(#1124),#11064,.T.);
#11564=ADVANCED_FACE('',(#1125),#360,.F.);
#11565=ADVANCED_FACE('',(#1126),#11065,.F.);
#11566=ADVANCED_FACE('',(#1127),#361,.F.);
#11567=ADVANCED_FACE('',(#1128),#11066,.F.);
#11568=ADVANCED_FACE('',(#1129),#362,.F.);
#11569=ADVANCED_FACE('',(#1130),#11067,.T.);
#11570=ADVANCED_FACE('',(#1131),#363,.F.);
#11571=ADVANCED_FACE('',(#1132),#364,.F.);
#11572=ADVANCED_FACE('',(#1133),#365,.F.);
#11573=ADVANCED_FACE('',(#1134),#366,.T.);
#11574=ADVANCED_FACE('',(#1135),#367,.T.);
#11575=ADVANCED_FACE('',(#1136),#368,.T.);
#11576=ADVANCED_FACE('',(#1137),#369,.F.);
#11577=ADVANCED_FACE('',(#1138),#370,.F.);
#11578=ADVANCED_FACE('',(#1139),#371,.F.);
#11579=ADVANCED_FACE('',(#1140),#11068,.T.);
#11580=ADVANCED_FACE('',(#1141),#372,.F.);
#11581=ADVANCED_FACE('',(#1142),#11069,.F.);
#11582=ADVANCED_FACE('',(#1143),#373,.F.);
#11583=ADVANCED_FACE('',(#1144),#11070,.F.);
#11584=ADVANCED_FACE('',(#1145),#374,.F.);
#11585=ADVANCED_FACE('',(#1146),#11071,.T.);
#11586=ADVANCED_FACE('',(#1147),#375,.F.);
#11587=ADVANCED_FACE('',(#1148),#376,.F.);
#11588=ADVANCED_FACE('',(#1149),#377,.F.);
#11589=ADVANCED_FACE('',(#1150),#378,.F.);
#11590=ADVANCED_FACE('',(#1151),#379,.F.);
#11591=ADVANCED_FACE('',(#1152),#11072,.T.);
#11592=ADVANCED_FACE('',(#1153),#380,.F.);
#11593=ADVANCED_FACE('',(#1154),#11073,.F.);
#11594=ADVANCED_FACE('',(#1155),#381,.F.);
#11595=ADVANCED_FACE('',(#1156),#11074,.F.);
#11596=ADVANCED_FACE('',(#1157),#382,.F.);
#11597=ADVANCED_FACE('',(#1158),#11075,.T.);
#11598=ADVANCED_FACE('',(#1159),#383,.F.);
#11599=ADVANCED_FACE('',(#1160),#384,.F.);
#11600=ADVANCED_FACE('',(#1161),#385,.F.);
#11601=ADVANCED_FACE('',(#1162),#386,.T.);
#11602=ADVANCED_FACE('',(#1163),#387,.T.);
#11603=ADVANCED_FACE('',(#1164),#388,.T.);
#11604=ADVANCED_FACE('',(#1165),#389,.F.);
#11605=ADVANCED_FACE('',(#1166),#390,.F.);
#11606=ADVANCED_FACE('',(#1167),#391,.F.);
#11607=ADVANCED_FACE('',(#1168),#11076,.T.);
#11608=ADVANCED_FACE('',(#1169),#392,.F.);
#11609=ADVANCED_FACE('',(#1170),#11077,.F.);
#11610=ADVANCED_FACE('',(#1171),#393,.F.);
#11611=ADVANCED_FACE('',(#1172),#11078,.F.);
#11612=ADVANCED_FACE('',(#1173),#394,.F.);
#11613=ADVANCED_FACE('',(#1174),#11079,.T.);
#11614=ADVANCED_FACE('',(#1175),#395,.F.);
#11615=ADVANCED_FACE('',(#1176),#396,.F.);
#11616=ADVANCED_FACE('',(#1177),#397,.F.);
#11617=ADVANCED_FACE('',(#1178),#398,.T.);
#11618=ADVANCED_FACE('',(#1179),#399,.F.);
#11619=ADVANCED_FACE('',(#1180),#400,.F.);
#11620=ADVANCED_FACE('',(#1181),#401,.F.);
#11621=ADVANCED_FACE('',(#1182),#11080,.T.);
#11622=ADVANCED_FACE('',(#1183),#402,.F.);
#11623=ADVANCED_FACE('',(#1184),#11081,.F.);
#11624=ADVANCED_FACE('',(#1185),#403,.F.);
#11625=ADVANCED_FACE('',(#1186),#11082,.F.);
#11626=ADVANCED_FACE('',(#1187),#404,.F.);
#11627=ADVANCED_FACE('',(#1188),#11083,.T.);
#11628=ADVANCED_FACE('',(#1189),#405,.F.);
#11629=ADVANCED_FACE('',(#1190),#406,.F.);
#11630=ADVANCED_FACE('',(#1191),#407,.F.);
#11631=ADVANCED_FACE('',(#1192),#408,.F.);
#11632=ADVANCED_FACE('',(#1193),#409,.F.);
#11633=ADVANCED_FACE('',(#1194),#410,.F.);
#11634=ADVANCED_FACE('',(#1195),#411,.F.);
#11635=ADVANCED_FACE('',(#1196),#11084,.T.);
#11636=ADVANCED_FACE('',(#1197),#412,.F.);
#11637=ADVANCED_FACE('',(#1198),#11085,.F.);
#11638=ADVANCED_FACE('',(#1199),#413,.F.);
#11639=ADVANCED_FACE('',(#1200),#11086,.F.);
#11640=ADVANCED_FACE('',(#1201),#414,.F.);
#11641=ADVANCED_FACE('',(#1202),#11087,.T.);
#11642=ADVANCED_FACE('',(#1203),#415,.F.);
#11643=ADVANCED_FACE('',(#1204),#416,.F.);
#11644=ADVANCED_FACE('',(#1205),#417,.F.);
#11645=ADVANCED_FACE('',(#1206),#418,.F.);
#11646=ADVANCED_FACE('',(#1207),#419,.F.);
#11647=ADVANCED_FACE('',(#1208),#11088,.T.);
#11648=ADVANCED_FACE('',(#1209),#420,.F.);
#11649=ADVANCED_FACE('',(#1210),#11089,.F.);
#11650=ADVANCED_FACE('',(#1211),#421,.F.);
#11651=ADVANCED_FACE('',(#1212),#11090,.T.);
#11652=ADVANCED_FACE('',(#1213),#422,.F.);
#11653=ADVANCED_FACE('',(#1214),#423,.F.);
#11654=ADVANCED_FACE('',(#1215),#424,.F.);
#11655=ADVANCED_FACE('',(#1216),#425,.T.);
#11656=ADVANCED_FACE('',(#1217),#426,.F.);
#11657=ADVANCED_FACE('',(#1218),#427,.F.);
#11658=ADVANCED_FACE('',(#1219),#11091,.T.);
#11659=ADVANCED_FACE('',(#1220),#428,.F.);
#11660=ADVANCED_FACE('',(#1221),#11092,.F.);
#11661=ADVANCED_FACE('',(#1222),#429,.F.);
#11662=ADVANCED_FACE('',(#1223),#11093,.T.);
#11663=ADVANCED_FACE('',(#1224),#430,.F.);
#11664=ADVANCED_FACE('',(#1225),#431,.F.);
#11665=ADVANCED_FACE('',(#1226),#432,.F.);
#11666=ADVANCED_FACE('',(#1227),#433,.T.);
#11667=ADVANCED_FACE('',(#1228),#434,.F.);
#11668=ADVANCED_FACE('',(#1229),#435,.F.);
#11669=ADVANCED_FACE('',(#1230),#11094,.T.);
#11670=ADVANCED_FACE('',(#1231),#436,.F.);
#11671=ADVANCED_FACE('',(#1232),#11095,.F.);
#11672=ADVANCED_FACE('',(#1233),#437,.F.);
#11673=ADVANCED_FACE('',(#1234),#11096,.T.);
#11674=ADVANCED_FACE('',(#1235),#438,.F.);
#11675=ADVANCED_FACE('',(#1236),#439,.F.);
#11676=ADVANCED_FACE('',(#1237),#440,.F.);
#11677=ADVANCED_FACE('',(#1238),#441,.T.);
#11678=ADVANCED_FACE('',(#1239),#442,.F.);
#11679=ADVANCED_FACE('',(#1240),#443,.F.);
#11680=ADVANCED_FACE('',(#1241),#11097,.T.);
#11681=ADVANCED_FACE('',(#1242),#444,.F.);
#11682=ADVANCED_FACE('',(#1243),#11098,.F.);
#11683=ADVANCED_FACE('',(#1244),#445,.F.);
#11684=ADVANCED_FACE('',(#1245),#11099,.T.);
#11685=ADVANCED_FACE('',(#1246),#446,.F.);
#11686=ADVANCED_FACE('',(#1247),#447,.F.);
#11687=ADVANCED_FACE('',(#1248),#448,.F.);
#11688=ADVANCED_FACE('',(#1249),#449,.T.);
#11689=ADVANCED_FACE('',(#1250),#450,.F.);
#11690=ADVANCED_FACE('',(#1251),#451,.F.);
#11691=ADVANCED_FACE('',(#1252),#452,.F.);
#11692=ADVANCED_FACE('',(#1253),#11100,.T.);
#11693=ADVANCED_FACE('',(#1254),#453,.F.);
#11694=ADVANCED_FACE('',(#1255),#11101,.F.);
#11695=ADVANCED_FACE('',(#1256),#454,.F.);
#11696=ADVANCED_FACE('',(#1257),#11102,.T.);
#11697=ADVANCED_FACE('',(#1258),#455,.F.);
#11698=ADVANCED_FACE('',(#1259),#456,.F.);
#11699=ADVANCED_FACE('',(#1260),#457,.F.);
#11700=ADVANCED_FACE('',(#1261),#458,.F.);
#11701=ADVANCED_FACE('',(#1262),#459,.F.);
#11702=ADVANCED_FACE('',(#1263),#11103,.T.);
#11703=ADVANCED_FACE('',(#1264),#460,.F.);
#11704=ADVANCED_FACE('',(#1265),#11104,.F.);
#11705=ADVANCED_FACE('',(#1266),#461,.F.);
#11706=ADVANCED_FACE('',(#1267),#11105,.T.);
#11707=ADVANCED_FACE('',(#1268),#462,.F.);
#11708=ADVANCED_FACE('',(#1269),#463,.F.);
#11709=ADVANCED_FACE('',(#1270),#464,.T.);
#11710=ADVANCED_FACE('',(#1271),#465,.T.);
#11711=ADVANCED_FACE('',(#1272),#466,.T.);
#11712=ADVANCED_FACE('',(#1273),#467,.F.);
#11713=ADVANCED_FACE('',(#1274),#468,.F.);
#11714=ADVANCED_FACE('',(#1275),#11106,.T.);
#11715=ADVANCED_FACE('',(#1276),#469,.F.);
#11716=ADVANCED_FACE('',(#1277),#11107,.F.);
#11717=ADVANCED_FACE('',(#1278),#470,.F.);
#11718=ADVANCED_FACE('',(#1279),#11108,.T.);
#11719=ADVANCED_FACE('',(#1280),#471,.F.);
#11720=ADVANCED_FACE('',(#1281),#472,.F.);
#11721=ADVANCED_FACE('',(#1282),#473,.F.);
#11722=ADVANCED_FACE('',(#1283),#474,.T.);
#11723=ADVANCED_FACE('',(#1284),#475,.F.);
#11724=ADVANCED_FACE('',(#1285),#476,.F.);
#11725=ADVANCED_FACE('',(#1286),#11109,.T.);
#11726=ADVANCED_FACE('',(#1287),#477,.F.);
#11727=ADVANCED_FACE('',(#1288),#11110,.F.);
#11728=ADVANCED_FACE('',(#1289),#478,.F.);
#11729=ADVANCED_FACE('',(#1290),#11111,.T.);
#11730=ADVANCED_FACE('',(#1291),#479,.F.);
#11731=ADVANCED_FACE('',(#1292),#480,.F.);
#11732=ADVANCED_FACE('',(#1293),#481,.F.);
#11733=ADVANCED_FACE('',(#1294),#482,.F.);
#11734=ADVANCED_FACE('',(#1295),#483,.F.);
#11735=ADVANCED_FACE('',(#1296),#11112,.T.);
#11736=ADVANCED_FACE('',(#1297),#484,.F.);
#11737=ADVANCED_FACE('',(#1298),#11113,.F.);
#11738=ADVANCED_FACE('',(#1299),#485,.F.);
#11739=ADVANCED_FACE('',(#1300),#11114,.T.);
#11740=ADVANCED_FACE('',(#1301),#486,.F.);
#11741=ADVANCED_FACE('',(#1302),#487,.F.);
#11742=ADVANCED_FACE('',(#1303),#488,.T.);
#11743=ADVANCED_FACE('',(#1304),#489,.T.);
#11744=ADVANCED_FACE('',(#1305),#490,.F.);
#11745=ADVANCED_FACE('',(#1306),#491,.F.);
#11746=ADVANCED_FACE('',(#1307),#492,.F.);
#11747=ADVANCED_FACE('',(#1308),#11115,.T.);
#11748=ADVANCED_FACE('',(#1309),#493,.F.);
#11749=ADVANCED_FACE('',(#1310),#11116,.F.);
#11750=ADVANCED_FACE('',(#1311),#494,.F.);
#11751=ADVANCED_FACE('',(#1312),#11117,.T.);
#11752=ADVANCED_FACE('',(#1313),#495,.F.);
#11753=ADVANCED_FACE('',(#1314),#496,.F.);
#11754=ADVANCED_FACE('',(#1315),#497,.F.);
#11755=ADVANCED_FACE('',(#1316),#11118,.F.);
#11756=ADVANCED_FACE('',(#1317),#11119,.F.);
#11757=ADVANCED_FACE('',(#1318),#11120,.F.);
#11758=ADVANCED_FACE('',(#1319),#11121,.F.);
#11759=ADVANCED_FACE('',(#1320),#498,.F.);
#11760=ADVANCED_FACE('',(#1321),#499,.F.);
#11761=ADVANCED_FACE('',(#1322),#500,.F.);
#11762=ADVANCED_FACE('',(#1323),#501,.F.);
#11763=ADVANCED_FACE('',(#1324,#597,#598,#599,#600),#502,.F.);
#11764=ADVANCED_FACE('',(#1325,#601,#602,#603,#604),#503,.T.);
#11765=ADVANCED_FACE('',(#1326),#504,.F.);
#11766=ADVANCED_FACE('',(#1327),#11122,.F.);
#11767=ADVANCED_FACE('',(#1328),#505,.F.);
#11768=ADVANCED_FACE('',(#1329),#506,.F.);
#11769=ADVANCED_FACE('',(#1330),#11123,.F.);
#11770=ADVANCED_FACE('',(#1331),#507,.F.);
#11771=ADVANCED_FACE('',(#1332),#508,.F.);
#11772=ADVANCED_FACE('',(#1333),#11124,.F.);
#11773=ADVANCED_FACE('',(#1334),#509,.F.);
#11774=ADVANCED_FACE('',(#1335),#510,.F.);
#11775=ADVANCED_FACE('',(#1336),#11125,.F.);
#11776=ADVANCED_FACE('',(#1337),#511,.F.);
#11777=ADVANCED_FACE('',(#1338),#512,.F.);
#11778=ADVANCED_FACE('',(#1339),#513,.F.);
#11779=ADVANCED_FACE('',(#1340),#514,.F.);
#11780=ADVANCED_FACE('',(#1341),#515,.F.);
#11781=ADVANCED_FACE('',(#1342),#11126,.F.);
#11782=ADVANCED_FACE('',(#1343),#11127,.F.);
#11783=ADVANCED_FACE('',(#1344),#516,.F.);
#11784=ADVANCED_FACE('',(#1345),#517,.F.);
#11785=ADVANCED_FACE('',(#1346),#11128,.T.);
#11786=ADVANCED_FACE('',(#1347),#518,.F.);
#11787=ADVANCED_FACE('',(#1348),#11129,.F.);
#11788=ADVANCED_FACE('',(#1349,#605,#606),#519,.F.);
#11789=ADVANCED_FACE('',(#1350),#11130,.F.);
#11790=ADVANCED_FACE('',(#1351),#520,.F.);
#11791=ADVANCED_FACE('',(#1352),#11131,.T.);
#11792=ADVANCED_FACE('',(#1353),#521,.F.);
#11793=ADVANCED_FACE('',(#1354),#522,.F.);
#11794=ADVANCED_FACE('',(#1355,#607,#608),#523,.F.);
#11795=ADVANCED_FACE('',(#1356),#524,.T.);
#11796=ADVANCED_FACE('',(#1357),#525,.T.);
#11797=ADVANCED_FACE('',(#1358),#11132,.F.);
#11798=ADVANCED_FACE('',(#1359),#11133,.F.);
#11799=ADVANCED_FACE('',(#1360,#609,#610),#526,.F.);
#11800=ADVANCED_FACE('',(#1361),#527,.F.);
#11801=ADVANCED_FACE('',(#1362),#11134,.T.);
#11802=ADVANCED_FACE('',(#1363,#611,#612),#528,.F.);
#11803=ADVANCED_FACE('',(#1364),#11135,.F.);
#11804=ADVANCED_FACE('',(#1365),#529,.F.);
#11805=ADVANCED_FACE('',(#1366),#11136,.T.);
#11806=ADVANCED_FACE('',(#1367),#530,.F.);
#11807=ADVANCED_FACE('',(#1368),#531,.F.);
#11808=ADVANCED_FACE('',(#1369),#532,.F.);
#11809=ADVANCED_FACE('',(#1370),#533,.T.);
#11810=ADVANCED_FACE('',(#1371),#11137,.F.);
#11811=ADVANCED_FACE('',(#1372),#11138,.F.);
#11812=ADVANCED_FACE('',(#1373,#613,#614),#534,.F.);
#11813=ADVANCED_FACE('',(#1374),#535,.F.);
#11814=ADVANCED_FACE('',(#1375),#11139,.T.);
#11815=ADVANCED_FACE('',(#1376,#615,#616),#536,.F.);
#11816=ADVANCED_FACE('',(#1377),#11140,.F.);
#11817=ADVANCED_FACE('',(#1378),#537,.F.);
#11818=ADVANCED_FACE('',(#1379),#11141,.T.);
#11819=ADVANCED_FACE('',(#1380),#538,.F.);
#11820=ADVANCED_FACE('',(#1381),#539,.F.);
#11821=ADVANCED_FACE('',(#1382),#540,.F.);
#11822=ADVANCED_FACE('',(#1383),#541,.T.);
#11826=CLOSED_SHELL('',(#11505,#11506,#11507,#11508,#11509,#11510,#11511,
#11512,#11513,#11514,#11515,#11516,#11517,#11518));
#11827=CLOSED_SHELL('',(#11519,#11520,#11521,#11522,#11523,#11524,#11525,
#11526,#11527,#11528,#11529,#11530,#11531,#11532));
#11828=CLOSED_SHELL('',(#11533,#11534,#11535,#11536,#11537,#11538,#11539,
#11540,#11541,#11542,#11543,#11544,#11545,#11546));
#11829=CLOSED_SHELL('',(#11547,#11548,#11549,#11550,#11551,#11552,#11553,
#11554,#11555,#11556,#11557,#11558,#11559,#11560));
#11830=CLOSED_SHELL('',(#11561,#11562,#11563,#11564,#11565,#11566,#11567,
#11568,#11569,#11570,#11571,#11572,#11573,#11574));
#11831=CLOSED_SHELL('',(#11575,#11576,#11577,#11578,#11579,#11580,#11581,
#11582,#11583,#11584,#11585,#11586,#11587,#11588));
#11832=CLOSED_SHELL('',(#11589,#11590,#11591,#11592,#11593,#11594,#11595,
#11596,#11597,#11598,#11599,#11600,#11601,#11602));
#11833=CLOSED_SHELL('',(#11603,#11604,#11605,#11606,#11607,#11608,#11609,
#11610,#11611,#11612,#11613,#11614,#11615,#11616));
#11834=CLOSED_SHELL('',(#11617,#11618,#11619,#11620,#11621,#11622,#11623,
#11624,#11625,#11626,#11627,#11628,#11629,#11630));
#11835=CLOSED_SHELL('',(#11631,#11632,#11633,#11634,#11635,#11636,#11637,
#11638,#11639,#11640,#11641,#11642,#11643,#11644));
#11836=CLOSED_SHELL('',(#11645,#11646,#11647,#11648,#11649,#11650,#11651,
#11652,#11653,#11654,#11655));
#11837=CLOSED_SHELL('',(#11656,#11657,#11658,#11659,#11660,#11661,#11662,
#11663,#11664,#11665,#11666));
#11838=CLOSED_SHELL('',(#11667,#11668,#11669,#11670,#11671,#11672,#11673,
#11674,#11675,#11676,#11677));
#11839=CLOSED_SHELL('',(#11678,#11679,#11680,#11681,#11682,#11683,#11684,
#11685,#11686,#11687,#11688));
#11840=CLOSED_SHELL('',(#11689,#11690,#11691,#11692,#11693,#11694,#11695,
#11696,#11697,#11698,#11699));
#11841=CLOSED_SHELL('',(#11700,#11701,#11702,#11703,#11704,#11705,#11706,
#11707,#11708,#11709,#11710));
#11842=CLOSED_SHELL('',(#11711,#11712,#11713,#11714,#11715,#11716,#11717,
#11718,#11719,#11720,#11721));
#11843=CLOSED_SHELL('',(#11722,#11723,#11724,#11725,#11726,#11727,#11728,
#11729,#11730,#11731,#11732));
#11844=CLOSED_SHELL('',(#11733,#11734,#11735,#11736,#11737,#11738,#11739,
#11740,#11741,#11742,#11743));
#11845=CLOSED_SHELL('',(#11744,#11745,#11746,#11747,#11748,#11749,#11750,
#11751,#11752,#11753,#11754));
#11846=CLOSED_SHELL('',(#11755,#11756,#11757,#11758,#11759,#11760,#11761,
#11762,#11763,#11764,#11765,#11766,#11767,#11768,#11769,#11770,#11771,#11772,
#11773,#11774,#11775,#11776,#11777,#11778,#11779,#11780));
#11847=CLOSED_SHELL('',(#11781,#11782,#11783,#11784,#11785,#11786,#11787,
#11788,#11789,#11790,#11791,#11792,#11793,#11794,#11795,#11796));
#11848=CLOSED_SHELL('',(#11797,#11798,#11799,#11800,#11801,#11802,#11803,
#11804,#11805,#11806,#11807,#11808,#11809));
#11849=CLOSED_SHELL('',(#11810,#11811,#11812,#11813,#11814,#11815,#11816,
#11817,#11818,#11819,#11820,#11821,#11822));
#12666=AXIS2_PLACEMENT_3D('',#25857,#15109,#15110);
#12667=AXIS2_PLACEMENT_3D('',#25858,#15111,#15112);
#12668=AXIS2_PLACEMENT_3D('',#25867,#15117,#15118);
#12669=AXIS2_PLACEMENT_3D('',#25873,#15122,#15123);
#12670=AXIS2_PLACEMENT_3D('',#25875,#15124,#15125);
#12671=AXIS2_PLACEMENT_3D('',#25878,#15127,#15128);
#12672=AXIS2_PLACEMENT_3D('',#25879,#15129,#15130);
#12673=AXIS2_PLACEMENT_3D('',#25885,#15134,#15135);
#12674=AXIS2_PLACEMENT_3D('',#25887,#15136,#15137);
#12675=AXIS2_PLACEMENT_3D('',#25890,#15139,#15140);
#12676=AXIS2_PLACEMENT_3D('',#25891,#15141,#15142);
#12677=AXIS2_PLACEMENT_3D('',#25897,#15146,#15147);
#12678=AXIS2_PLACEMENT_3D('',#25899,#15148,#15149);
#12679=AXIS2_PLACEMENT_3D('',#25902,#15151,#15152);
#12680=AXIS2_PLACEMENT_3D('',#25903,#15153,#15154);
#12681=AXIS2_PLACEMENT_3D('',#25909,#15158,#15159);
#12682=AXIS2_PLACEMENT_3D('',#25911,#15160,#15161);
#12683=AXIS2_PLACEMENT_3D('',#25914,#15163,#15164);
#12684=AXIS2_PLACEMENT_3D('',#25915,#15165,#15166);
#12685=AXIS2_PLACEMENT_3D('',#25921,#15170,#15171);
#12686=AXIS2_PLACEMENT_3D('',#25927,#15175,#15176);
#12687=AXIS2_PLACEMENT_3D('',#25930,#15179,#15180);
#12688=AXIS2_PLACEMENT_3D('',#25931,#15181,#15182);
#12689=AXIS2_PLACEMENT_3D('',#25932,#15183,#15184);
#12690=AXIS2_PLACEMENT_3D('',#25937,#15186,#15187);
#12691=AXIS2_PLACEMENT_3D('',#25941,#15189,#15190);
#12692=AXIS2_PLACEMENT_3D('',#25945,#15192,#15193);
#12693=AXIS2_PLACEMENT_3D('',#25949,#15195,#15196);
#12694=AXIS2_PLACEMENT_3D('',#25957,#15201,#15202);
#12695=AXIS2_PLACEMENT_3D('',#25963,#15206,#15207);
#12696=AXIS2_PLACEMENT_3D('',#25967,#15210,#15211);
#12697=AXIS2_PLACEMENT_3D('',#25971,#15214,#15215);
#12698=AXIS2_PLACEMENT_3D('',#25974,#15217,#15218);
#12699=AXIS2_PLACEMENT_3D('',#25975,#15219,#15220);
#12700=AXIS2_PLACEMENT_3D('',#25979,#15223,#15224);
#12701=AXIS2_PLACEMENT_3D('',#25982,#15226,#15227);
#12702=AXIS2_PLACEMENT_3D('',#25983,#15228,#15229);
#12703=AXIS2_PLACEMENT_3D('',#25987,#15232,#15233);
#12704=AXIS2_PLACEMENT_3D('',#25990,#15235,#15236);
#12705=AXIS2_PLACEMENT_3D('',#25991,#15237,#15238);
#12706=AXIS2_PLACEMENT_3D('',#25995,#15241,#15242);
#12707=AXIS2_PLACEMENT_3D('',#25998,#15244,#15245);
#12708=AXIS2_PLACEMENT_3D('',#25999,#15246,#15247);
#12709=AXIS2_PLACEMENT_3D('',#26003,#15250,#15251);
#12710=AXIS2_PLACEMENT_3D('',#26005,#15253,#15254);
#12711=AXIS2_PLACEMENT_3D('',#26006,#15255,#15256);
#12712=AXIS2_PLACEMENT_3D('',#26019,#15262,#15263);
#12713=AXIS2_PLACEMENT_3D('',#26023,#15265,#15266);
#12714=AXIS2_PLACEMENT_3D('',#26027,#15268,#15269);
#12715=AXIS2_PLACEMENT_3D('',#26030,#15271,#15272);
#12716=AXIS2_PLACEMENT_3D('',#26031,#15273,#15274);
#12717=AXIS2_PLACEMENT_3D('',#26037,#15278,#15279);
#12718=AXIS2_PLACEMENT_3D('',#26041,#15282,#15283);
#12719=AXIS2_PLACEMENT_3D('',#26045,#15286,#15287);
#12720=AXIS2_PLACEMENT_3D('',#26047,#15288,#15289);
#12721=AXIS2_PLACEMENT_3D('',#26049,#15291,#15292);
#12722=AXIS2_PLACEMENT_3D('',#26053,#15295,#15296);
#12723=AXIS2_PLACEMENT_3D('',#26055,#15297,#15298);
#12724=AXIS2_PLACEMENT_3D('',#26057,#15300,#15301);
#12725=AXIS2_PLACEMENT_3D('',#26061,#15304,#15305);
#12726=AXIS2_PLACEMENT_3D('',#26063,#15306,#15307);
#12727=AXIS2_PLACEMENT_3D('',#26065,#15309,#15310);
#12728=AXIS2_PLACEMENT_3D('',#26069,#15313,#15314);
#12729=AXIS2_PLACEMENT_3D('',#26071,#15315,#15316);
#12730=AXIS2_PLACEMENT_3D('',#26073,#15318,#15319);
#12731=AXIS2_PLACEMENT_3D('',#26077,#15322,#15323);
#12732=AXIS2_PLACEMENT_3D('',#26079,#15325,#15326);
#12733=AXIS2_PLACEMENT_3D('',#26080,#15327,#15328);
#12734=AXIS2_PLACEMENT_3D('',#26089,#15333,#15334);
#12735=AXIS2_PLACEMENT_3D('',#26095,#15338,#15339);
#12736=AXIS2_PLACEMENT_3D('',#26097,#15340,#15341);
#12737=AXIS2_PLACEMENT_3D('',#26099,#15342,#15343);
#12738=AXIS2_PLACEMENT_3D('',#26101,#15345,#15346);
#12739=AXIS2_PLACEMENT_3D('',#26107,#15350,#15351);
#12740=AXIS2_PLACEMENT_3D('',#26109,#15352,#15353);
#12741=AXIS2_PLACEMENT_3D('',#26111,#15354,#15355);
#12742=AXIS2_PLACEMENT_3D('',#26113,#15357,#15358);
#12743=AXIS2_PLACEMENT_3D('',#26119,#15362,#15363);
#12744=AXIS2_PLACEMENT_3D('',#26121,#15364,#15365);
#12745=AXIS2_PLACEMENT_3D('',#26123,#15366,#15367);
#12746=AXIS2_PLACEMENT_3D('',#26125,#15369,#15370);
#12747=AXIS2_PLACEMENT_3D('',#26131,#15374,#15375);
#12748=AXIS2_PLACEMENT_3D('',#26133,#15376,#15377);
#12749=AXIS2_PLACEMENT_3D('',#26135,#15378,#15379);
#12750=AXIS2_PLACEMENT_3D('',#26137,#15381,#15382);
#12751=AXIS2_PLACEMENT_3D('',#26143,#15386,#15387);
#12752=AXIS2_PLACEMENT_3D('',#26149,#15391,#15392);
#12753=AXIS2_PLACEMENT_3D('',#26152,#15395,#15396);
#12754=AXIS2_PLACEMENT_3D('',#26153,#15397,#15398);
#12755=AXIS2_PLACEMENT_3D('',#26154,#15399,#15400);
#12756=AXIS2_PLACEMENT_3D('',#26163,#15405,#15406);
#12757=AXIS2_PLACEMENT_3D('',#26169,#15410,#15411);
#12758=AXIS2_PLACEMENT_3D('',#26171,#15412,#15413);
#12759=AXIS2_PLACEMENT_3D('',#26174,#15415,#15416);
#12760=AXIS2_PLACEMENT_3D('',#26175,#15417,#15418);
#12761=AXIS2_PLACEMENT_3D('',#26181,#15422,#15423);
#12762=AXIS2_PLACEMENT_3D('',#26183,#15424,#15425);
#12763=AXIS2_PLACEMENT_3D('',#26186,#15427,#15428);
#12764=AXIS2_PLACEMENT_3D('',#26187,#15429,#15430);
#12765=AXIS2_PLACEMENT_3D('',#26193,#15434,#15435);
#12766=AXIS2_PLACEMENT_3D('',#26195,#15436,#15437);
#12767=AXIS2_PLACEMENT_3D('',#26198,#15439,#15440);
#12768=AXIS2_PLACEMENT_3D('',#26199,#15441,#15442);
#12769=AXIS2_PLACEMENT_3D('',#26205,#15446,#15447);
#12770=AXIS2_PLACEMENT_3D('',#26207,#15448,#15449);
#12771=AXIS2_PLACEMENT_3D('',#26210,#15451,#15452);
#12772=AXIS2_PLACEMENT_3D('',#26211,#15453,#15454);
#12773=AXIS2_PLACEMENT_3D('',#26217,#15458,#15459);
#12774=AXIS2_PLACEMENT_3D('',#26223,#15463,#15464);
#12775=AXIS2_PLACEMENT_3D('',#26226,#15467,#15468);
#12776=AXIS2_PLACEMENT_3D('',#26227,#15469,#15470);
#12777=AXIS2_PLACEMENT_3D('',#26228,#15471,#15472);
#12778=AXIS2_PLACEMENT_3D('',#26241,#15478,#15479);
#12779=AXIS2_PLACEMENT_3D('',#26245,#15481,#15482);
#12780=AXIS2_PLACEMENT_3D('',#26249,#15484,#15485);
#12781=AXIS2_PLACEMENT_3D('',#26252,#15487,#15488);
#12782=AXIS2_PLACEMENT_3D('',#26253,#15489,#15490);
#12783=AXIS2_PLACEMENT_3D('',#26259,#15494,#15495);
#12784=AXIS2_PLACEMENT_3D('',#26263,#15498,#15499);
#12785=AXIS2_PLACEMENT_3D('',#26267,#15502,#15503);
#12786=AXIS2_PLACEMENT_3D('',#26269,#15504,#15505);
#12787=AXIS2_PLACEMENT_3D('',#26271,#15507,#15508);
#12788=AXIS2_PLACEMENT_3D('',#26275,#15511,#15512);
#12789=AXIS2_PLACEMENT_3D('',#26277,#15513,#15514);
#12790=AXIS2_PLACEMENT_3D('',#26279,#15516,#15517);
#12791=AXIS2_PLACEMENT_3D('',#26283,#15520,#15521);
#12792=AXIS2_PLACEMENT_3D('',#26285,#15522,#15523);
#12793=AXIS2_PLACEMENT_3D('',#26287,#15525,#15526);
#12794=AXIS2_PLACEMENT_3D('',#26291,#15529,#15530);
#12795=AXIS2_PLACEMENT_3D('',#26293,#15531,#15532);
#12796=AXIS2_PLACEMENT_3D('',#26295,#15534,#15535);
#12797=AXIS2_PLACEMENT_3D('',#26299,#15538,#15539);
#12798=AXIS2_PLACEMENT_3D('',#26301,#15541,#15542);
#12799=AXIS2_PLACEMENT_3D('',#26302,#15543,#15544);
#12800=AXIS2_PLACEMENT_3D('',#26311,#15549,#15550);
#12801=AXIS2_PLACEMENT_3D('',#26317,#15554,#15555);
#12802=AXIS2_PLACEMENT_3D('',#26319,#15556,#15557);
#12803=AXIS2_PLACEMENT_3D('',#26322,#15559,#15560);
#12804=AXIS2_PLACEMENT_3D('',#26323,#15561,#15562);
#12805=AXIS2_PLACEMENT_3D('',#26329,#15566,#15567);
#12806=AXIS2_PLACEMENT_3D('',#26331,#15568,#15569);
#12807=AXIS2_PLACEMENT_3D('',#26334,#15571,#15572);
#12808=AXIS2_PLACEMENT_3D('',#26335,#15573,#15574);
#12809=AXIS2_PLACEMENT_3D('',#26341,#15578,#15579);
#12810=AXIS2_PLACEMENT_3D('',#26343,#15580,#15581);
#12811=AXIS2_PLACEMENT_3D('',#26346,#15583,#15584);
#12812=AXIS2_PLACEMENT_3D('',#26347,#15585,#15586);
#12813=AXIS2_PLACEMENT_3D('',#26353,#15590,#15591);
#12814=AXIS2_PLACEMENT_3D('',#26355,#15592,#15593);
#12815=AXIS2_PLACEMENT_3D('',#26358,#15595,#15596);
#12816=AXIS2_PLACEMENT_3D('',#26359,#15597,#15598);
#12817=AXIS2_PLACEMENT_3D('',#26365,#15602,#15603);
#12818=AXIS2_PLACEMENT_3D('',#26371,#15607,#15608);
#12819=AXIS2_PLACEMENT_3D('',#26374,#15611,#15612);
#12820=AXIS2_PLACEMENT_3D('',#26375,#15613,#15614);
#12821=AXIS2_PLACEMENT_3D('',#26376,#15615,#15616);
#12822=AXIS2_PLACEMENT_3D('',#26389,#15622,#15623);
#12823=AXIS2_PLACEMENT_3D('',#26393,#15625,#15626);
#12824=AXIS2_PLACEMENT_3D('',#26397,#15628,#15629);
#12825=AXIS2_PLACEMENT_3D('',#26400,#15631,#15632);
#12826=AXIS2_PLACEMENT_3D('',#26401,#15633,#15634);
#12827=AXIS2_PLACEMENT_3D('',#26407,#15638,#15639);
#12828=AXIS2_PLACEMENT_3D('',#26411,#15642,#15643);
#12829=AXIS2_PLACEMENT_3D('',#26415,#15646,#15647);
#12830=AXIS2_PLACEMENT_3D('',#26417,#15648,#15649);
#12831=AXIS2_PLACEMENT_3D('',#26419,#15651,#15652);
#12832=AXIS2_PLACEMENT_3D('',#26423,#15655,#15656);
#12833=AXIS2_PLACEMENT_3D('',#26425,#15657,#15658);
#12834=AXIS2_PLACEMENT_3D('',#26427,#15660,#15661);
#12835=AXIS2_PLACEMENT_3D('',#26431,#15664,#15665);
#12836=AXIS2_PLACEMENT_3D('',#26433,#15666,#15667);
#12837=AXIS2_PLACEMENT_3D('',#26435,#15669,#15670);
#12838=AXIS2_PLACEMENT_3D('',#26439,#15673,#15674);
#12839=AXIS2_PLACEMENT_3D('',#26441,#15675,#15676);
#12840=AXIS2_PLACEMENT_3D('',#26443,#15678,#15679);
#12841=AXIS2_PLACEMENT_3D('',#26447,#15682,#15683);
#12842=AXIS2_PLACEMENT_3D('',#26449,#15685,#15686);
#12843=AXIS2_PLACEMENT_3D('',#26450,#15687,#15688);
#12844=AXIS2_PLACEMENT_3D('',#26457,#15691,#15692);
#12845=AXIS2_PLACEMENT_3D('',#26461,#15694,#15695);
#12846=AXIS2_PLACEMENT_3D('',#26465,#15697,#15698);
#12847=AXIS2_PLACEMENT_3D('',#26469,#15700,#15701);
#12848=AXIS2_PLACEMENT_3D('',#26475,#15705,#15706);
#12849=AXIS2_PLACEMENT_3D('',#26481,#15710,#15711);
#12850=AXIS2_PLACEMENT_3D('',#26485,#15714,#15715);
#12851=AXIS2_PLACEMENT_3D('',#26489,#15718,#15719);
#12852=AXIS2_PLACEMENT_3D('',#26492,#15721,#15722);
#12853=AXIS2_PLACEMENT_3D('',#26493,#15723,#15724);
#12854=AXIS2_PLACEMENT_3D('',#26497,#15727,#15728);
#12855=AXIS2_PLACEMENT_3D('',#26500,#15730,#15731);
#12856=AXIS2_PLACEMENT_3D('',#26501,#15732,#15733);
#12857=AXIS2_PLACEMENT_3D('',#26505,#15736,#15737);
#12858=AXIS2_PLACEMENT_3D('',#26508,#15739,#15740);
#12859=AXIS2_PLACEMENT_3D('',#26509,#15741,#15742);
#12860=AXIS2_PLACEMENT_3D('',#26513,#15745,#15746);
#12861=AXIS2_PLACEMENT_3D('',#26516,#15748,#15749);
#12862=AXIS2_PLACEMENT_3D('',#26517,#15750,#15751);
#12863=AXIS2_PLACEMENT_3D('',#26521,#15754,#15755);
#12864=AXIS2_PLACEMENT_3D('',#26523,#15757,#15758);
#12865=AXIS2_PLACEMENT_3D('',#26524,#15759,#15760);
#12866=AXIS2_PLACEMENT_3D('',#26535,#15765,#15766);
#12867=AXIS2_PLACEMENT_3D('',#26539,#15768,#15769);
#12868=AXIS2_PLACEMENT_3D('',#26543,#15771,#15772);
#12869=AXIS2_PLACEMENT_3D('',#26547,#15774,#15775);
#12870=AXIS2_PLACEMENT_3D('',#26549,#15777,#15778);
#12871=AXIS2_PLACEMENT_3D('',#26555,#15782,#15783);
#12872=AXIS2_PLACEMENT_3D('',#26559,#15786,#15787);
#12873=AXIS2_PLACEMENT_3D('',#26563,#15790,#15791);
#12874=AXIS2_PLACEMENT_3D('',#26565,#15792,#15793);
#12875=AXIS2_PLACEMENT_3D('',#26567,#15795,#15796);
#12876=AXIS2_PLACEMENT_3D('',#26571,#15799,#15800);
#12877=AXIS2_PLACEMENT_3D('',#26573,#15801,#15802);
#12878=AXIS2_PLACEMENT_3D('',#26575,#15804,#15805);
#12879=AXIS2_PLACEMENT_3D('',#26579,#15808,#15809);
#12880=AXIS2_PLACEMENT_3D('',#26581,#15810,#15811);
#12881=AXIS2_PLACEMENT_3D('',#26583,#15813,#15814);
#12882=AXIS2_PLACEMENT_3D('',#26587,#15817,#15818);
#12883=AXIS2_PLACEMENT_3D('',#26589,#15819,#15820);
#12884=AXIS2_PLACEMENT_3D('',#26591,#15822,#15823);
#12885=AXIS2_PLACEMENT_3D('',#26595,#15826,#15827);
#12886=AXIS2_PLACEMENT_3D('',#26597,#15829,#15830);
#12887=AXIS2_PLACEMENT_3D('',#26598,#15831,#15832);
#12888=AXIS2_PLACEMENT_3D('',#26607,#15837,#15838);
#12889=AXIS2_PLACEMENT_3D('',#26613,#15842,#15843);
#12890=AXIS2_PLACEMENT_3D('',#26615,#15844,#15845);
#12891=AXIS2_PLACEMENT_3D('',#26618,#15847,#15848);
#12892=AXIS2_PLACEMENT_3D('',#26619,#15849,#15850);
#12893=AXIS2_PLACEMENT_3D('',#26625,#15854,#15855);
#12894=AXIS2_PLACEMENT_3D('',#26627,#15856,#15857);
#12895=AXIS2_PLACEMENT_3D('',#26630,#15859,#15860);
#12896=AXIS2_PLACEMENT_3D('',#26631,#15861,#15862);
#12897=AXIS2_PLACEMENT_3D('',#26637,#15866,#15867);
#12898=AXIS2_PLACEMENT_3D('',#26639,#15868,#15869);
#12899=AXIS2_PLACEMENT_3D('',#26642,#15871,#15872);
#12900=AXIS2_PLACEMENT_3D('',#26643,#15873,#15874);
#12901=AXIS2_PLACEMENT_3D('',#26649,#15878,#15879);
#12902=AXIS2_PLACEMENT_3D('',#26652,#15882,#15883);
#12903=AXIS2_PLACEMENT_3D('',#26653,#15884,#15885);
#12904=AXIS2_PLACEMENT_3D('',#26654,#15886,#15887);
#12905=AXIS2_PLACEMENT_3D('',#26663,#15892,#15893);
#12906=AXIS2_PLACEMENT_3D('',#26669,#15897,#15898);
#12907=AXIS2_PLACEMENT_3D('',#26671,#15899,#15900);
#12908=AXIS2_PLACEMENT_3D('',#26674,#15902,#15903);
#12909=AXIS2_PLACEMENT_3D('',#26675,#15904,#15905);
#12910=AXIS2_PLACEMENT_3D('',#26681,#15909,#15910);
#12911=AXIS2_PLACEMENT_3D('',#26683,#15911,#15912);
#12912=AXIS2_PLACEMENT_3D('',#26686,#15914,#15915);
#12913=AXIS2_PLACEMENT_3D('',#26687,#15916,#15917);
#12914=AXIS2_PLACEMENT_3D('',#26693,#15921,#15922);
#12915=AXIS2_PLACEMENT_3D('',#26695,#15923,#15924);
#12916=AXIS2_PLACEMENT_3D('',#26698,#15926,#15927);
#12917=AXIS2_PLACEMENT_3D('',#26699,#15928,#15929);
#12918=AXIS2_PLACEMENT_3D('',#26705,#15933,#15934);
#12919=AXIS2_PLACEMENT_3D('',#26708,#15937,#15938);
#12920=AXIS2_PLACEMENT_3D('',#26709,#15939,#15940);
#12921=AXIS2_PLACEMENT_3D('',#26710,#15941,#15942);
#12922=AXIS2_PLACEMENT_3D('',#26719,#15947,#15948);
#12923=AXIS2_PLACEMENT_3D('',#26725,#15952,#15953);
#12924=AXIS2_PLACEMENT_3D('',#26727,#15954,#15955);
#12925=AXIS2_PLACEMENT_3D('',#26729,#15956,#15957);
#12926=AXIS2_PLACEMENT_3D('',#26731,#15959,#15960);
#12927=AXIS2_PLACEMENT_3D('',#26737,#15964,#15965);
#12928=AXIS2_PLACEMENT_3D('',#26739,#15966,#15967);
#12929=AXIS2_PLACEMENT_3D('',#26741,#15968,#15969);
#12930=AXIS2_PLACEMENT_3D('',#26743,#15971,#15972);
#12931=AXIS2_PLACEMENT_3D('',#26749,#15976,#15977);
#12932=AXIS2_PLACEMENT_3D('',#26751,#15978,#15979);
#12933=AXIS2_PLACEMENT_3D('',#26753,#15980,#15981);
#12934=AXIS2_PLACEMENT_3D('',#26755,#15983,#15984);
#12935=AXIS2_PLACEMENT_3D('',#26761,#15988,#15989);
#12936=AXIS2_PLACEMENT_3D('',#26764,#15992,#15993);
#12937=AXIS2_PLACEMENT_3D('',#26765,#15994,#15995);
#12938=AXIS2_PLACEMENT_3D('',#26766,#15996,#15997);
#12939=AXIS2_PLACEMENT_3D('',#26775,#16002,#16003);
#12940=AXIS2_PLACEMENT_3D('',#26781,#16007,#16008);
#12941=AXIS2_PLACEMENT_3D('',#26783,#16009,#16010);
#12942=AXIS2_PLACEMENT_3D('',#26785,#16011,#16012);
#12943=AXIS2_PLACEMENT_3D('',#26787,#16014,#16015);
#12944=AXIS2_PLACEMENT_3D('',#26793,#16019,#16020);
#12945=AXIS2_PLACEMENT_3D('',#26795,#16021,#16022);
#12946=AXIS2_PLACEMENT_3D('',#26797,#16023,#16024);
#12947=AXIS2_PLACEMENT_3D('',#26799,#16026,#16027);
#12948=AXIS2_PLACEMENT_3D('',#26805,#16031,#16032);
#12949=AXIS2_PLACEMENT_3D('',#26807,#16033,#16034);
#12950=AXIS2_PLACEMENT_3D('',#26809,#16035,#16036);
#12951=AXIS2_PLACEMENT_3D('',#26811,#16038,#16039);
#12952=AXIS2_PLACEMENT_3D('',#26817,#16043,#16044);
#12953=AXIS2_PLACEMENT_3D('',#26820,#16047,#16048);
#12954=AXIS2_PLACEMENT_3D('',#26821,#16049,#16050);
#12955=AXIS2_PLACEMENT_3D('',#26822,#16051,#16052);
#12956=AXIS2_PLACEMENT_3D('',#26829,#16055,#16056);
#12957=AXIS2_PLACEMENT_3D('',#26833,#16058,#16059);
#12958=AXIS2_PLACEMENT_3D('',#26837,#16061,#16062);
#12959=AXIS2_PLACEMENT_3D('',#26841,#16065,#16066);
#12960=AXIS2_PLACEMENT_3D('',#26847,#16070,#16071);
#12961=AXIS2_PLACEMENT_3D('',#26851,#16074,#16075);
#12962=AXIS2_PLACEMENT_3D('',#26854,#16077,#16078);
#12963=AXIS2_PLACEMENT_3D('',#26855,#16079,#16080);
#12964=AXIS2_PLACEMENT_3D('',#26859,#16083,#16084);
#12965=AXIS2_PLACEMENT_3D('',#26862,#16086,#16087);
#12966=AXIS2_PLACEMENT_3D('',#26863,#16088,#16089);
#12967=AXIS2_PLACEMENT_3D('',#26867,#16092,#16093);
#12968=AXIS2_PLACEMENT_3D('',#26870,#16095,#16096);
#12969=AXIS2_PLACEMENT_3D('',#26871,#16097,#16098);
#12970=AXIS2_PLACEMENT_3D('',#26875,#16101,#16102);
#12971=AXIS2_PLACEMENT_3D('',#26877,#16104,#16105);
#12972=AXIS2_PLACEMENT_3D('',#26878,#16106,#16107);
#12973=AXIS2_PLACEMENT_3D('',#26887,#16112,#16113);
#12974=AXIS2_PLACEMENT_3D('',#26893,#16117,#16118);
#12975=AXIS2_PLACEMENT_3D('',#26895,#16119,#16120);
#12976=AXIS2_PLACEMENT_3D('',#26898,#16122,#16123);
#12977=AXIS2_PLACEMENT_3D('',#26899,#16124,#16125);
#12978=AXIS2_PLACEMENT_3D('',#26905,#16129,#16130);
#12979=AXIS2_PLACEMENT_3D('',#26907,#16131,#16132);
#12980=AXIS2_PLACEMENT_3D('',#26910,#16134,#16135);
#12981=AXIS2_PLACEMENT_3D('',#26911,#16136,#16137);
#12982=AXIS2_PLACEMENT_3D('',#26917,#16141,#16142);
#12983=AXIS2_PLACEMENT_3D('',#26919,#16143,#16144);
#12984=AXIS2_PLACEMENT_3D('',#26922,#16146,#16147);
#12985=AXIS2_PLACEMENT_3D('',#26923,#16148,#16149);
#12986=AXIS2_PLACEMENT_3D('',#26929,#16153,#16154);
#12987=AXIS2_PLACEMENT_3D('',#26932,#16157,#16158);
#12988=AXIS2_PLACEMENT_3D('',#26933,#16159,#16160);
#12989=AXIS2_PLACEMENT_3D('',#26934,#16161,#16162);
#12990=AXIS2_PLACEMENT_3D('',#26943,#16166,#16167);
#12991=AXIS2_PLACEMENT_3D('',#26947,#16169,#16170);
#12992=AXIS2_PLACEMENT_3D('',#26951,#16172,#16173);
#12993=AXIS2_PLACEMENT_3D('',#26953,#16175,#16176);
#12994=AXIS2_PLACEMENT_3D('',#26959,#16180,#16181);
#12995=AXIS2_PLACEMENT_3D('',#26963,#16184,#16185);
#12996=AXIS2_PLACEMENT_3D('',#26965,#16186,#16187);
#12997=AXIS2_PLACEMENT_3D('',#26967,#16189,#16190);
#12998=AXIS2_PLACEMENT_3D('',#26971,#16193,#16194);
#12999=AXIS2_PLACEMENT_3D('',#26973,#16195,#16196);
#13000=AXIS2_PLACEMENT_3D('',#26975,#16198,#16199);
#13001=AXIS2_PLACEMENT_3D('',#26979,#16202,#16203);
#13002=AXIS2_PLACEMENT_3D('',#26981,#16204,#16205);
#13003=AXIS2_PLACEMENT_3D('',#26983,#16207,#16208);
#13004=AXIS2_PLACEMENT_3D('',#26987,#16211,#16212);
#13005=AXIS2_PLACEMENT_3D('',#26989,#16214,#16215);
#13006=AXIS2_PLACEMENT_3D('',#26990,#16216,#16217);
#13007=AXIS2_PLACEMENT_3D('',#26999,#16221,#16222);
#13008=AXIS2_PLACEMENT_3D('',#27003,#16224,#16225);
#13009=AXIS2_PLACEMENT_3D('',#27007,#16227,#16228);
#13010=AXIS2_PLACEMENT_3D('',#27009,#16230,#16231);
#13011=AXIS2_PLACEMENT_3D('',#27015,#16235,#16236);
#13012=AXIS2_PLACEMENT_3D('',#27019,#16239,#16240);
#13013=AXIS2_PLACEMENT_3D('',#27021,#16241,#16242);
#13014=AXIS2_PLACEMENT_3D('',#27023,#16244,#16245);
#13015=AXIS2_PLACEMENT_3D('',#27027,#16248,#16249);
#13016=AXIS2_PLACEMENT_3D('',#27029,#16250,#16251);
#13017=AXIS2_PLACEMENT_3D('',#27031,#16253,#16254);
#13018=AXIS2_PLACEMENT_3D('',#27035,#16257,#16258);
#13019=AXIS2_PLACEMENT_3D('',#27037,#16259,#16260);
#13020=AXIS2_PLACEMENT_3D('',#27039,#16262,#16263);
#13021=AXIS2_PLACEMENT_3D('',#27043,#16266,#16267);
#13022=AXIS2_PLACEMENT_3D('',#27045,#16269,#16270);
#13023=AXIS2_PLACEMENT_3D('',#27046,#16271,#16272);
#13024=AXIS2_PLACEMENT_3D('',#27055,#16277,#16278);
#13025=AXIS2_PLACEMENT_3D('',#27061,#16282,#16283);
#13026=AXIS2_PLACEMENT_3D('',#27063,#16284,#16285);
#13027=AXIS2_PLACEMENT_3D('',#27065,#16286,#16287);
#13028=AXIS2_PLACEMENT_3D('',#27067,#16289,#16290);
#13029=AXIS2_PLACEMENT_3D('',#27073,#16294,#16295);
#13030=AXIS2_PLACEMENT_3D('',#27075,#16296,#16297);
#13031=AXIS2_PLACEMENT_3D('',#27077,#16298,#16299);
#13032=AXIS2_PLACEMENT_3D('',#27079,#16301,#16302);
#13033=AXIS2_PLACEMENT_3D('',#27085,#16306,#16307);
#13034=AXIS2_PLACEMENT_3D('',#27087,#16308,#16309);
#13035=AXIS2_PLACEMENT_3D('',#27089,#16310,#16311);
#13036=AXIS2_PLACEMENT_3D('',#27091,#16313,#16314);
#13037=AXIS2_PLACEMENT_3D('',#27097,#16318,#16319);
#13038=AXIS2_PLACEMENT_3D('',#27100,#16322,#16323);
#13039=AXIS2_PLACEMENT_3D('',#27101,#16324,#16325);
#13040=AXIS2_PLACEMENT_3D('',#27102,#16326,#16327);
#13041=AXIS2_PLACEMENT_3D('',#27109,#16330,#16331);
#13042=AXIS2_PLACEMENT_3D('',#27113,#16333,#16334);
#13043=AXIS2_PLACEMENT_3D('',#27117,#16336,#16337);
#13044=AXIS2_PLACEMENT_3D('',#27121,#16340,#16341);
#13045=AXIS2_PLACEMENT_3D('',#27127,#16345,#16346);
#13046=AXIS2_PLACEMENT_3D('',#27131,#16349,#16350);
#13047=AXIS2_PLACEMENT_3D('',#27134,#16352,#16353);
#13048=AXIS2_PLACEMENT_3D('',#27135,#16354,#16355);
#13049=AXIS2_PLACEMENT_3D('',#27139,#16358,#16359);
#13050=AXIS2_PLACEMENT_3D('',#27142,#16361,#16362);
#13051=AXIS2_PLACEMENT_3D('',#27143,#16363,#16364);
#13052=AXIS2_PLACEMENT_3D('',#27147,#16367,#16368);
#13053=AXIS2_PLACEMENT_3D('',#27150,#16370,#16371);
#13054=AXIS2_PLACEMENT_3D('',#27151,#16372,#16373);
#13055=AXIS2_PLACEMENT_3D('',#27155,#16376,#16377);
#13056=AXIS2_PLACEMENT_3D('',#27157,#16379,#16380);
#13057=AXIS2_PLACEMENT_3D('',#27158,#16381,#16382);
#13058=AXIS2_PLACEMENT_3D('',#27161,#16383,#16384);
#13059=AXIS2_PLACEMENT_3D('',#27165,#16386,#16387);
#13060=AXIS2_PLACEMENT_3D('',#27167,#16389,#16390);
#13061=AXIS2_PLACEMENT_3D('',#27170,#16391,#16392);
#13062=AXIS2_PLACEMENT_3D('',#27174,#16394,#16395);
#13063=AXIS2_PLACEMENT_3D('',#27176,#16397,#16398);
#13064=AXIS2_PLACEMENT_3D('',#27179,#16399,#16400);
#13065=AXIS2_PLACEMENT_3D('',#27183,#16402,#16403);
#13066=AXIS2_PLACEMENT_3D('',#27185,#16405,#16406);
#13067=AXIS2_PLACEMENT_3D('',#27188,#16407,#16408);
#13068=AXIS2_PLACEMENT_3D('',#27192,#16410,#16411);
#13069=AXIS2_PLACEMENT_3D('',#27194,#16413,#16414);
#13070=AXIS2_PLACEMENT_3D('',#27203,#16419,#16420);
#13071=AXIS2_PLACEMENT_3D('',#27212,#16425,#16426);
#13072=AXIS2_PLACEMENT_3D('',#27221,#16431,#16432);
#13073=AXIS2_PLACEMENT_3D('',#27230,#16437,#16438);
#13074=AXIS2_PLACEMENT_3D('',#27239,#16445,#16446);
#13075=AXIS2_PLACEMENT_3D('',#27244,#16449,#16450);
#13076=AXIS2_PLACEMENT_3D('',#27249,#16453,#16454);
#13077=AXIS2_PLACEMENT_3D('',#27254,#16457,#16458);
#13078=AXIS2_PLACEMENT_3D('',#27255,#16459,#16460);
#13079=AXIS2_PLACEMENT_3D('',#27263,#16466,#16467);
#13080=AXIS2_PLACEMENT_3D('',#27268,#16470,#16471);
#13081=AXIS2_PLACEMENT_3D('',#27273,#16474,#16475);
#13082=AXIS2_PLACEMENT_3D('',#27278,#16478,#16479);
#13083=AXIS2_PLACEMENT_3D('',#27280,#16481,#16482);
#13084=AXIS2_PLACEMENT_3D('',#27282,#16484,#16485);
#13085=AXIS2_PLACEMENT_3D('',#27284,#16487,#16488);
#13086=AXIS2_PLACEMENT_3D('',#27285,#16489,#16490);
#13087=AXIS2_PLACEMENT_3D('',#27287,#16492,#16493);
#13088=AXIS2_PLACEMENT_3D('',#27289,#16495,#16496);
#13089=AXIS2_PLACEMENT_3D('',#27290,#16497,#16498);
#13090=AXIS2_PLACEMENT_3D('',#27292,#16500,#16501);
#13091=AXIS2_PLACEMENT_3D('',#27294,#16503,#16504);
#13092=AXIS2_PLACEMENT_3D('',#27295,#16505,#16506);
#13093=AXIS2_PLACEMENT_3D('',#27297,#16508,#16509);
#13094=AXIS2_PLACEMENT_3D('',#27299,#16511,#16512);
#13095=AXIS2_PLACEMENT_3D('',#27300,#16513,#16514);
#13096=AXIS2_PLACEMENT_3D('',#27301,#16515,#16516);
#13097=AXIS2_PLACEMENT_3D('',#27302,#16517,#16518);
#13098=AXIS2_PLACEMENT_3D('',#27303,#16519,#16520);
#13099=AXIS2_PLACEMENT_3D('',#27304,#16521,#16522);
#13100=AXIS2_PLACEMENT_3D('',#27306,#16523,#16524);
#13101=AXIS2_PLACEMENT_3D('',#27309,#16526,#16527);
#13102=AXIS2_PLACEMENT_3D('',#27310,#16528,#16529);
#13103=AXIS2_PLACEMENT_3D('',#27312,#16530,#16531);
#13104=AXIS2_PLACEMENT_3D('',#27315,#16533,#16534);
#13105=AXIS2_PLACEMENT_3D('',#27316,#16535,#16536);
#13106=AXIS2_PLACEMENT_3D('',#27325,#16541,#16542);
#13107=AXIS2_PLACEMENT_3D('',#27331,#16546,#16547);
#13108=AXIS2_PLACEMENT_3D('',#27333,#16548,#16549);
#13109=AXIS2_PLACEMENT_3D('',#27336,#16551,#16552);
#13110=AXIS2_PLACEMENT_3D('',#27337,#16553,#16554);
#13111=AXIS2_PLACEMENT_3D('',#27343,#16558,#16559);
#13112=AXIS2_PLACEMENT_3D('',#27345,#16560,#16561);
#13113=AXIS2_PLACEMENT_3D('',#27348,#16563,#16564);
#13114=AXIS2_PLACEMENT_3D('',#27349,#16565,#16566);
#13115=AXIS2_PLACEMENT_3D('',#27355,#16570,#16571);
#13116=AXIS2_PLACEMENT_3D('',#27357,#16572,#16573);
#13117=AXIS2_PLACEMENT_3D('',#27360,#16575,#16576);
#13118=AXIS2_PLACEMENT_3D('',#27361,#16577,#16578);
#13119=AXIS2_PLACEMENT_3D('',#27367,#16582,#16583);
#13120=AXIS2_PLACEMENT_3D('',#27369,#16584,#16585);
#13121=AXIS2_PLACEMENT_3D('',#27372,#16587,#16588);
#13122=AXIS2_PLACEMENT_3D('',#27373,#16589,#16590);
#13123=AXIS2_PLACEMENT_3D('',#27379,#16594,#16595);
#13124=AXIS2_PLACEMENT_3D('',#27385,#16599,#16600);
#13125=AXIS2_PLACEMENT_3D('',#27388,#16603,#16604);
#13126=AXIS2_PLACEMENT_3D('',#27389,#16605,#16606);
#13127=AXIS2_PLACEMENT_3D('',#27390,#16607,#16608);
#13128=AXIS2_PLACEMENT_3D('',#27392,#16609,#16610);
#13129=AXIS2_PLACEMENT_3D('',#27395,#16612,#16613);
#13130=AXIS2_PLACEMENT_3D('',#27396,#16614,#16615);
#13131=AXIS2_PLACEMENT_3D('',#27398,#16616,#16617);
#13132=AXIS2_PLACEMENT_3D('',#27401,#16619,#16620);
#13133=AXIS2_PLACEMENT_3D('',#27402,#16621,#16622);
#13134=AXIS2_PLACEMENT_3D('',#27411,#16627,#16628);
#13135=AXIS2_PLACEMENT_3D('',#27417,#16632,#16633);
#13136=AXIS2_PLACEMENT_3D('',#27419,#16634,#16635);
#13137=AXIS2_PLACEMENT_3D('',#27422,#16637,#16638);
#13138=AXIS2_PLACEMENT_3D('',#27423,#16639,#16640);
#13139=AXIS2_PLACEMENT_3D('',#27429,#16644,#16645);
#13140=AXIS2_PLACEMENT_3D('',#27431,#16646,#16647);
#13141=AXIS2_PLACEMENT_3D('',#27434,#16649,#16650);
#13142=AXIS2_PLACEMENT_3D('',#27435,#16651,#16652);
#13143=AXIS2_PLACEMENT_3D('',#27441,#16656,#16657);
#13144=AXIS2_PLACEMENT_3D('',#27443,#16658,#16659);
#13145=AXIS2_PLACEMENT_3D('',#27446,#16661,#16662);
#13146=AXIS2_PLACEMENT_3D('',#27447,#16663,#16664);
#13147=AXIS2_PLACEMENT_3D('',#27453,#16668,#16669);
#13148=AXIS2_PLACEMENT_3D('',#27456,#16672,#16673);
#13149=AXIS2_PLACEMENT_3D('',#27457,#16674,#16675);
#13150=AXIS2_PLACEMENT_3D('',#27458,#16676,#16677);
#13151=AXIS2_PLACEMENT_3D('',#27460,#16678,#16679);
#13152=AXIS2_PLACEMENT_3D('',#27463,#16681,#16682);
#13153=AXIS2_PLACEMENT_3D('',#27464,#16683,#16684);
#13154=AXIS2_PLACEMENT_3D('',#27466,#16685,#16686);
#13155=AXIS2_PLACEMENT_3D('',#27469,#16688,#16689);
#13156=AXIS2_PLACEMENT_3D('',#27470,#16690,#16691);
#13157=AXIS2_PLACEMENT_3D('',#27479,#16696,#16697);
#13158=AXIS2_PLACEMENT_3D('',#27485,#16701,#16702);
#13159=AXIS2_PLACEMENT_3D('',#27487,#16703,#16704);
#13160=AXIS2_PLACEMENT_3D('',#27489,#16705,#16706);
#13161=AXIS2_PLACEMENT_3D('',#27491,#16708,#16709);
#13162=AXIS2_PLACEMENT_3D('',#27497,#16713,#16714);
#13163=AXIS2_PLACEMENT_3D('',#27499,#16715,#16716);
#13164=AXIS2_PLACEMENT_3D('',#27501,#16717,#16718);
#13165=AXIS2_PLACEMENT_3D('',#27503,#16720,#16721);
#13166=AXIS2_PLACEMENT_3D('',#27509,#16725,#16726);
#13167=AXIS2_PLACEMENT_3D('',#27511,#16727,#16728);
#13168=AXIS2_PLACEMENT_3D('',#27513,#16729,#16730);
#13169=AXIS2_PLACEMENT_3D('',#27515,#16732,#16733);
#13170=AXIS2_PLACEMENT_3D('',#27521,#16737,#16738);
#13171=AXIS2_PLACEMENT_3D('',#27524,#16741,#16742);
#13172=AXIS2_PLACEMENT_3D('',#27525,#16743,#16744);
#15109=DIRECTION('axis',(0.,0.,1.));
#15110=DIRECTION('refdir',(1.,0.,0.));
#15111=DIRECTION('center_axis',(0.,1.,0.));
#15112=DIRECTION('ref_axis',(0.,0.,1.));
#15113=DIRECTION('',(1.,0.,6.12323399573677E-17));
#15114=DIRECTION('',(0.,0.,1.));
#15115=DIRECTION('',(-1.,0.,0.));
#15116=DIRECTION('',(0.,0.,1.));
#15117=DIRECTION('center_axis',(1.,0.,0.));
#15118=DIRECTION('ref_axis',(0.,0.,-1.));
#15119=DIRECTION('',(0.,-1.,0.));
#15120=DIRECTION('',(0.,0.,1.));
#15121=DIRECTION('',(0.,1.,0.));
#15122=DIRECTION('center_axis',(0.,0.,1.));
#15123=DIRECTION('ref_axis',(1.,0.,0.));
#15124=DIRECTION('center_axis',(-6.12323399573677E-17,0.,1.));
#15125=DIRECTION('ref_axis',(1.,0.,6.12323399573677E-17));
#15126=DIRECTION('',(0.,0.,1.));
#15127=DIRECTION('center_axis',(0.,0.,-1.));
#15128=DIRECTION('ref_axis',(-1.,0.,0.));
#15129=DIRECTION('center_axis',(0.164410656039629,-0.986391978972162,0.));
#15130=DIRECTION('ref_axis',(0.986391978972162,0.164410656039629,0.));
#15131=DIRECTION('',(-0.986391978972162,-0.164410656039629,-6.03990889876441E-17));
#15132=DIRECTION('',(0.,0.,1.));
#15133=DIRECTION('',(0.986391978972162,0.164410656039629,0.));
#15134=DIRECTION('center_axis',(0.,0.,1.));
#15135=DIRECTION('ref_axis',(1.,0.,0.));
#15136=DIRECTION('center_axis',(6.12323399573677E-17,0.,-1.));
#15137=DIRECTION('ref_axis',(1.,-1.01179555320898E-15,6.12323399573676E-17));
#15138=DIRECTION('',(0.,0.,1.));
#15139=DIRECTION('center_axis',(0.,0.,1.));
#15140=DIRECTION('ref_axis',(-1.,0.,0.));
#15141=DIRECTION('center_axis',(1.,0.,0.));
#15142=DIRECTION('ref_axis',(0.,0.,-1.));
#15143=DIRECTION('',(0.,-1.,0.));
#15144=DIRECTION('',(0.,0.,1.));
#15145=DIRECTION('',(0.,1.,0.));
#15146=DIRECTION('center_axis',(0.,0.,1.));
#15147=DIRECTION('ref_axis',(1.,0.,0.));
#15148=DIRECTION('center_axis',(6.12323399573677E-17,0.,-1.));
#15149=DIRECTION('ref_axis',(1.,-1.01179555320898E-15,6.12323399573676E-17));
#15150=DIRECTION('',(0.,0.,1.));
#15151=DIRECTION('center_axis',(0.,0.,1.));
#15152=DIRECTION('ref_axis',(-1.,1.77064221811572E-15,0.));
#15153=DIRECTION('center_axis',(0.164410656039629,0.986391978972162,0.));
#15154=DIRECTION('ref_axis',(-0.986391978972162,0.164410656039629,0.));
#15155=DIRECTION('',(0.986391978972162,-0.164410656039629,6.03990889876441E-17));
#15156=DIRECTION('',(0.,0.,1.));
#15157=DIRECTION('',(-0.986391978972162,0.164410656039629,0.));
#15158=DIRECTION('center_axis',(0.,0.,1.));
#15159=DIRECTION('ref_axis',(1.,0.,0.));
#15160=DIRECTION('center_axis',(-6.12323399573677E-17,0.,1.));
#15161=DIRECTION('ref_axis',(1.,0.,6.12323399573677E-17));
#15162=DIRECTION('',(0.,0.,1.));
#15163=DIRECTION('center_axis',(0.,0.,-1.));
#15164=DIRECTION('ref_axis',(-1.,0.,0.));
#15165=DIRECTION('center_axis',(1.,0.,0.));
#15166=DIRECTION('ref_axis',(0.,0.,-1.));
#15167=DIRECTION('',(0.,-1.,0.));
#15168=DIRECTION('',(0.,0.,1.));
#15169=DIRECTION('',(0.,1.,0.));
#15170=DIRECTION('center_axis',(0.,-1.,0.));
#15171=DIRECTION('ref_axis',(0.,0.,-1.));
#15172=DIRECTION('',(-1.,0.,-6.12323399573677E-17));
#15173=DIRECTION('',(0.,0.,1.));
#15174=DIRECTION('',(1.,0.,0.));
#15175=DIRECTION('center_axis',(-1.,0.,0.));
#15176=DIRECTION('ref_axis',(0.,0.,1.));
#15177=DIRECTION('',(0.,1.,0.));
#15178=DIRECTION('',(0.,-1.,0.));
#15179=DIRECTION('center_axis',(0.,0.,-1.));
#15180=DIRECTION('ref_axis',(-1.,0.,0.));
#15181=DIRECTION('center_axis',(-6.12323399573677E-17,0.,1.));
#15182=DIRECTION('ref_axis',(1.,0.,6.12323399573677E-17));
#15183=DIRECTION('center_axis',(-1.,1.6672859221772E-24,-3.30995181697817E-47));
#15184=DIRECTION('ref_axis',(0.,1.98523347012726E-23,1.));
#15185=DIRECTION('',(-1.70606001339062E-24,1.,1.32348898008484E-23));
#15186=DIRECTION('center_axis',(-1.,1.6672859221772E-24,0.));
#15187=DIRECTION('ref_axis',(0.,0.,1.));
#15188=DIRECTION('',(0.,0.164410656039629,-0.986391978972162));
#15189=DIRECTION('center_axis',(1.,-1.6672859221772E-24,0.));
#15190=DIRECTION('ref_axis',(3.37390496397365E-39,2.02359110641796E-15,
1.));
#15191=DIRECTION('',(-1.70606001339062E-24,1.,1.32348898008484E-23));
#15192=DIRECTION('center_axis',(1.,-1.6672859221772E-24,0.));
#15193=DIRECTION('ref_axis',(4.63911932546376E-39,2.7824377713247E-15,1.));
#15194=DIRECTION('',(0.,0.164410656039629,0.986391978972162));
#15195=DIRECTION('center_axis',(-1.,1.6672859221772E-24,0.));
#15196=DIRECTION('ref_axis',(0.,0.,1.));
#15197=DIRECTION('',(-1.70606001339062E-24,1.,1.32348898008484E-23));
#15198=DIRECTION('',(-2.16840434497101E-19,1.98523347012726E-23,1.));
#15199=DIRECTION('',(1.70606001339062E-24,-1.,-1.32348898008484E-23));
#15200=DIRECTION('',(-2.16840434497101E-19,1.98523347012726E-23,1.));
#15201=DIRECTION('center_axis',(2.16840434497101E-19,1.98523347012726E-23,
1.));
#15202=DIRECTION('ref_axis',(1.,-2.52031592887251E-24,-2.16840434497101E-19));
#15203=DIRECTION('',(1.,-2.52031592887251E-24,-2.16840434497101E-19));
#15204=DIRECTION('',(1.70606001339062E-24,-1.,-1.32348898008484E-23));
#15205=DIRECTION('',(1.,-2.52031592887251E-24,-2.16840434497101E-19));
#15206=DIRECTION('center_axis',(1.70606001339062E-24,-1.,1.98523347012726E-23));
#15207=DIRECTION('ref_axis',(-9.11574503592928E-64,-1.98523347012726E-23,
-1.));
#15208=DIRECTION('',(1.,-2.52031592887251E-24,-2.16840434497101E-19));
#15209=DIRECTION('',(-0.198787259314375,-1.98523347012726E-23,-0.980042665160185));
#15210=DIRECTION('center_axis',(-2.16840434497101E-19,-1.98523347012726E-23,
-1.));
#15211=DIRECTION('ref_axis',(-1.,2.52031592887251E-24,2.16840434497101E-19));
#15212=DIRECTION('',(1.,-2.52031592887251E-24,-2.16840434497101E-19));
#15213=DIRECTION('',(-1.70606001339062E-24,1.,1.32348898008484E-23));
#15214=DIRECTION('center_axis',(1.,-2.52031592887251E-24,-2.16840434497101E-19));
#15215=DIRECTION('ref_axis',(-2.16840434497101E-19,5.46506401086678E-43,
-1.));
#15216=DIRECTION('',(1.,-2.52031592887251E-24,-2.16840434497101E-19));
#15217=DIRECTION('center_axis',(-0.980042665160176,-7.49762143682472E-14,
0.198787259314424));
#15218=DIRECTION('ref_axis',(0.198787259314424,-4.70069536847622E-12,0.980042665160176));
#15219=DIRECTION('center_axis',(1.0842021724855E-19,0.986391978972162,-0.164410656039629));
#15220=DIRECTION('ref_axis',(-1.44445765116552E-36,0.164410656039629,0.986391978972162));
#15221=DIRECTION('',(1.,-2.52031592887251E-24,-2.16840434497101E-19));
#15222=DIRECTION('',(0.196186965810001,0.161215582689263,0.967222937250987));
#15223=DIRECTION('center_axis',(1.,-2.52031592887251E-24,-2.16840434497101E-19));
#15224=DIRECTION('ref_axis',(-2.16840434497101E-19,5.46506401086678E-43,
-1.));
#15225=DIRECTION('',(1.,-2.52031592887251E-24,-2.16840434497101E-19));
#15226=DIRECTION('center_axis',(0.980042665160181,4.41011730354711E-14,
-0.198787259314396));
#15227=DIRECTION('ref_axis',(0.198787259314396,-7.64602919273965E-13,0.980042665160181));
#15228=DIRECTION('center_axis',(-2.16840434497101E-19,-1.98523347012726E-23,
-1.));
#15229=DIRECTION('ref_axis',(-1.,2.52031592887251E-24,2.16840434497101E-19));
#15230=DIRECTION('',(1.,-2.52031592887251E-24,-2.16840434497101E-19));
#15231=DIRECTION('',(-1.70606001339062E-24,1.,1.32348898008484E-23));
#15232=DIRECTION('center_axis',(1.,-2.52031592887251E-24,-2.16840434497101E-19));
#15233=DIRECTION('ref_axis',(-2.16840434497101E-19,5.46506401086678E-43,
-1.));
#15234=DIRECTION('',(1.,-2.52031592887251E-24,-2.16840434497101E-19));
#15235=DIRECTION('center_axis',(0.980042665160188,1.60789922741767E-14,
-0.198787259314364));
#15236=DIRECTION('ref_axis',(0.198787259314364,7.36955750229359E-12,0.980042665160188));
#15237=DIRECTION('center_axis',(1.0842021724855E-19,-0.986391978972162,
-0.164410656039629));
#15238=DIRECTION('ref_axis',(2.16840434497101E-19,0.164410656039629,-0.986391978972162));
#15239=DIRECTION('',(1.,-2.52031592887251E-24,-2.16840434497101E-19));
#15240=DIRECTION('',(-0.196186965810001,0.161215582689263,-0.967222937250987));
#15241=DIRECTION('center_axis',(1.,-2.52031592887251E-24,-2.16840434497101E-19));
#15242=DIRECTION('ref_axis',(-2.16840434497101E-19,5.46506401086678E-43,
-1.));
#15243=DIRECTION('',(1.,-2.52031592887251E-24,-2.16840434497101E-19));
#15244=DIRECTION('center_axis',(-0.980042665160195,-9.32929719057768E-14,
0.198787259314327));
#15245=DIRECTION('ref_axis',(0.198787259314327,2.85203844610398E-12,0.980042665160195));
#15246=DIRECTION('center_axis',(-2.16840434497101E-19,-1.98523347012726E-23,
-1.));
#15247=DIRECTION('ref_axis',(-1.,2.52031592887251E-24,2.16840434497101E-19));
#15248=DIRECTION('',(1.,-2.52031592887251E-24,-2.16840434497101E-19));
#15249=DIRECTION('',(-1.70606001339062E-24,1.,1.32348898008484E-23));
#15250=DIRECTION('center_axis',(-1.70606001339062E-24,1.,-1.98523347012726E-23));
#15251=DIRECTION('ref_axis',(9.11574503592928E-64,1.98523347012726E-23,
1.));
#15252=DIRECTION('',(0.198787259314375,1.98523347012726E-23,0.980042665160185));
#15253=DIRECTION('center_axis',(-0.980042665160186,8.27180612553027E-24,
0.198787259314375));
#15254=DIRECTION('ref_axis',(0.198787259314375,1.98523347012726E-23,0.980042665160185));
#15255=DIRECTION('center_axis',(-0.980042665160186,-3.47415857272272E-23,
0.198787259314375));
#15256=DIRECTION('ref_axis',(0.198787259314375,-6.61744490042422E-24,0.980042665160185));
#15257=DIRECTION('',(2.40300129244162E-15,1.,1.18470558471201E-14));
#15258=DIRECTION('',(-0.198787259314375,6.79161872365112E-15,-0.980042665160185));
#15259=DIRECTION('',(-1.45507196095848E-15,-1.,-7.17366179404169E-15));
#15260=DIRECTION('',(0.198787259314375,-6.79161872365112E-15,0.980042665160185));
#15261=DIRECTION('',(3.30872245021211E-23,1.,-1.32348898008484E-23));
#15262=DIRECTION('center_axis',(-0.980042665160169,5.02500160127644E-14,
0.198787259314459));
#15263=DIRECTION('ref_axis',(0.198787259314459,7.90533358256112E-12,0.980042665160169));
#15264=DIRECTION('',(-0.196186965810001,0.161215582689269,-0.967222937250986));
#15265=DIRECTION('center_axis',(0.980042665160191,2.27047187493627E-14,
-0.198787259314346));
#15266=DIRECTION('ref_axis',(0.198787259314346,3.87807928502627E-12,0.980042665160191));
#15267=DIRECTION('',(1.54401270509304E-15,1.,7.61214923421315E-15));
#15268=DIRECTION('center_axis',(0.980042665160188,-1.48340309301132E-14,
-0.198787259314363));
#15269=DIRECTION('ref_axis',(0.198787259314363,-3.96081673643786E-12,0.980042665160188));
#15270=DIRECTION('',(0.196186965810001,0.161215582689256,0.967222937250988));
#15271=DIRECTION('center_axis',(-0.980042665160184,-1.70918421812105E-14,
0.198787259314383));
#15272=DIRECTION('ref_axis',(0.198787259314383,-4.35767870224177E-11,0.980042665160184));
#15273=DIRECTION('center_axis',(0.389639990836698,-7.17366180396786E-15,
0.920967251068559));
#15274=DIRECTION('ref_axis',(0.920967251068559,2.57459965496616E-23,-0.389639990836698));
#15275=DIRECTION('',(-0.920967251068559,-2.65990265724083E-23,0.389639990836698));
#15276=DIRECTION('',(-1.45507196095848E-15,-1.,-7.17366179404169E-15));
#15277=DIRECTION('',(-0.920967251068559,-2.65990265724083E-23,0.389639990836698));
#15278=DIRECTION('center_axis',(2.70017457815614E-15,1.,6.38223076123854E-15));
#15279=DIRECTION('ref_axis',(-2.22044604925031E-16,-6.38223076123854E-15,
1.));
#15280=DIRECTION('',(0.198787259314375,-6.79161872365112E-15,0.980042665160185));
#15281=DIRECTION('',(-0.920967251068559,-2.65990265724083E-23,0.389639990836698));
#15282=DIRECTION('center_axis',(-0.389639990836698,-7.3468396926393E-39,
-0.920967251068559));
#15283=DIRECTION('ref_axis',(-0.920967251068559,-2.65990265724083E-23,0.389639990836698));
#15284=DIRECTION('',(3.30872245021211E-23,1.,-1.32348898008484E-23));
#15285=DIRECTION('',(-0.920967251068559,-2.65990265724083E-23,0.389639990836698));
#15286=DIRECTION('center_axis',(-0.920967251068559,-2.65990265724083E-23,
0.389639990836698));
#15287=DIRECTION('ref_axis',(0.389639990836698,2.27914651832168E-37,0.920967251068559));
#15288=DIRECTION('center_axis',(-0.980042665160215,-1.25938390471903E-13,
0.19878725931423));
#15289=DIRECTION('ref_axis',(0.19878725931423,2.5853135894082E-11,0.980042665160215));
#15290=DIRECTION('',(-0.920967251068559,-2.65990265724083E-23,0.389639990836698));
#15291=DIRECTION('center_axis',(-0.0640609665127394,-0.986391978972161,
-0.151416829939202));
#15292=DIRECTION('ref_axis',(3.8859753641063E-16,0.151728482244607,-0.988422211241607));
#15293=DIRECTION('',(-0.196186965810001,0.161215582689269,-0.967222937250986));
#15294=DIRECTION('',(-0.920967251068559,-2.65990265724083E-23,0.389639990836698));
#15295=DIRECTION('center_axis',(-0.920967251068559,-2.65990265724083E-23,
0.389639990836698));
#15296=DIRECTION('ref_axis',(0.389639990836698,5.40790242502236E-38,0.920967251068559));
#15297=DIRECTION('center_axis',(0.980042665160185,-4.60002666111622E-15,
-0.198787259314377));
#15298=DIRECTION('ref_axis',(0.198787259314377,2.73860543621281E-12,0.980042665160185));
#15299=DIRECTION('',(-0.920967251068559,-2.65990265724083E-23,0.389639990836698));
#15300=DIRECTION('center_axis',(-0.389639990836698,7.61214924744803E-15,
-0.920967251068559));
#15301=DIRECTION('ref_axis',(-0.920967251068559,-2.6599026609348E-23,0.389639990836698));
#15302=DIRECTION('',(1.54401270509304E-15,1.,7.61214923421315E-15));
#15303=DIRECTION('',(-0.920967251068559,-2.65990265724083E-23,0.389639990836698));
#15304=DIRECTION('center_axis',(-0.920967251068559,-2.65990265724083E-23,
0.389639990836698));
#15305=DIRECTION('ref_axis',(0.389639990836698,3.20788036696344E-38,0.920967251068559));
#15306=DIRECTION('center_axis',(0.980042665160175,4.09782191554472E-14,
-0.198787259314427));
#15307=DIRECTION('ref_axis',(0.198787259314427,-1.19923446014724E-11,0.980042665160175));
#15308=DIRECTION('',(-0.920967251068559,-2.65990265724083E-23,0.389639990836698));
#15309=DIRECTION('center_axis',(-0.0640609665127342,0.986391978972163,-0.15141682993919));
#15310=DIRECTION('ref_axis',(-2.80362758003424E-16,0.151728482244595,0.988422211241609));
#15311=DIRECTION('',(0.196186965810001,0.161215582689256,0.967222937250988));
#15312=DIRECTION('',(-0.920967251068559,-2.65990265724083E-23,0.389639990836698));
#15313=DIRECTION('center_axis',(-0.920967251068559,-2.65990265724083E-23,
0.389639990836698));
#15314=DIRECTION('ref_axis',(0.389639990836698,2.27914651832168E-37,0.920967251068559));
#15315=DIRECTION('center_axis',(-0.980042665160188,-5.1617363387258E-14,
0.198787259314362));
#15316=DIRECTION('ref_axis',(0.198787259314362,4.05302242487948E-11,0.980042665160188));
#15317=DIRECTION('',(-0.920967251068559,-2.65990265724083E-23,0.389639990836698));
#15318=DIRECTION('center_axis',(-0.389639990836698,1.18470558636637E-14,
-0.920967251068559));
#15319=DIRECTION('ref_axis',(-0.920967251068559,-2.6599026296095E-23,0.389639990836698));
#15320=DIRECTION('',(2.40300129244162E-15,1.,1.18470558471201E-14));
#15321=DIRECTION('',(-0.920967251068559,-2.65990265724083E-23,0.389639990836698));
#15322=DIRECTION('center_axis',(-2.70017457815614E-15,-1.,-6.38223076123854E-15));
#15323=DIRECTION('ref_axis',(2.22044604925031E-16,6.38223076123854E-15,
-1.));
#15324=DIRECTION('',(-0.198787259314375,6.79161872365112E-15,-0.980042665160185));
#15325=DIRECTION('center_axis',(-0.980042665160186,-5.12851979782877E-23,
0.198787259314375));
#15326=DIRECTION('ref_axis',(0.198787259314375,-6.61744490042422E-24,0.980042665160185));
#15327=DIRECTION('center_axis',(5.76441489372891E-24,-1.,-6.92992146256797E-15));
#15328=DIRECTION('ref_axis',(1.3010426069826E-18,6.92992146256797E-15,-1.));
#15329=DIRECTION('',(1.3010426069826E-18,-1.98523347012727E-23,-1.));
#15330=DIRECTION('',(-1.,3.41212002678124E-24,8.67361737988404E-19));
#15331=DIRECTION('',(-0.198787259314375,6.79161869718135E-15,-0.980042665160185));
#15332=DIRECTION('',(-1.,3.41212002678124E-24,8.67361737988404E-19));
#15333=DIRECTION('center_axis',(1.3010426069826E-18,1.18470558768986E-14,
-1.));
#15334=DIRECTION('ref_axis',(-5.81611368201347E-24,1.,1.18470558768986E-14));
#15335=DIRECTION('',(5.81611368201347E-24,-1.,-1.18470558768986E-14));
#15336=DIRECTION('',(2.40300126044007E-15,1.,1.18470558768986E-14));
#15337=DIRECTION('',(-1.,3.41212002678124E-24,8.67361737988404E-19));
#15338=DIRECTION('center_axis',(-1.,3.41212002678124E-24,8.67361737988404E-19));
#15339=DIRECTION('ref_axis',(8.67361737988404E-19,-2.95954235665401E-42,
1.));
#15340=DIRECTION('center_axis',(1.,-3.41212002678124E-24,-8.67361737988404E-19));
#15341=DIRECTION('ref_axis',(-8.67361737988404E-19,2.95954235665401E-42,
-1.));
#15342=DIRECTION('center_axis',(-0.980042665160201,6.09039309723804E-14,
0.198787259314301));
#15343=DIRECTION('ref_axis',(0.198787259314301,1.98355794240169E-13,0.9800426651602));
#15344=DIRECTION('',(-1.,3.41212002678124E-24,8.67361737988404E-19));
#15345=DIRECTION('center_axis',(5.42101086242754E-20,0.986391978972163,
-0.164410656039623));
#15346=DIRECTION('ref_axis',(-1.3010426069826E-18,0.164410656039623,0.986391978972163));
#15347=DIRECTION('',(1.3010426069826E-18,-0.164410656039623,-0.986391978972163));
#15348=DIRECTION('',(0.196186965810001,0.161215582689256,0.967222937250988));
#15349=DIRECTION('',(-1.,3.41212002678124E-24,8.67361737988404E-19));
#15350=DIRECTION('center_axis',(-1.,3.41212002678124E-24,8.67361737988404E-19));
#15351=DIRECTION('ref_axis',(8.67361737988404E-19,-2.95954235665401E-42,
1.));
#15352=DIRECTION('center_axis',(-1.,3.41212002678124E-24,8.67361737988404E-19));
#15353=DIRECTION('ref_axis',(-8.67361737988404E-19,-2.30183488355044E-14,
-1.));
#15354=DIRECTION('center_axis',(0.980042665160188,-1.44120101355155E-14,
-0.198787259314364));
#15355=DIRECTION('ref_axis',(0.198787259314364,9.45740959535352E-13,0.980042665160188));
#15356=DIRECTION('',(-1.,3.41212002678124E-24,8.67361737988404E-19));
#15357=DIRECTION('center_axis',(1.3010426069826E-18,7.61214926068292E-15,
-1.));
#15358=DIRECTION('ref_axis',(-6.15215580586314E-24,1.,7.61214926068292E-15));
#15359=DIRECTION('',(6.15215580586314E-24,-1.,-7.61214926068292E-15));
#15360=DIRECTION('',(1.54401265703901E-15,1.,7.61214926730037E-15));
#15361=DIRECTION('',(-1.,3.41212002678124E-24,8.67361737988404E-19));
#15362=DIRECTION('center_axis',(-1.,3.41212002678124E-24,8.67361737988404E-19));
#15363=DIRECTION('ref_axis',(8.67361737988404E-19,-2.95954235665401E-42,
1.));
#15364=DIRECTION('center_axis',(-1.,3.41212002678124E-24,8.67361737988404E-19));
#15365=DIRECTION('ref_axis',(-8.67361737988404E-19,-1.01179555320898E-15,
-1.));
#15366=DIRECTION('center_axis',(0.980042665160185,-5.02204745571411E-15,
-0.198787259314378));
#15367=DIRECTION('ref_axis',(0.198787259314378,7.98881519935689E-12,0.980042665160185));
#15368=DIRECTION('',(-1.,3.41212002678124E-24,8.67361737988404E-19));
#15369=DIRECTION('center_axis',(2.40741243048404E-35,-0.986391978972161,
-0.164410656039636));
#15370=DIRECTION('ref_axis',(4.33680868994201E-19,0.164410656039636,-0.986391978972161));
#15371=DIRECTION('',(-4.33680868994201E-19,-0.164410656039636,0.986391978972161));
#15372=DIRECTION('',(-0.196186965810001,0.161215582689269,-0.967222937250986));
#15373=DIRECTION('',(-1.,3.41212002678124E-24,8.67361737988404E-19));
#15374=DIRECTION('center_axis',(-1.,3.41212002678124E-24,8.67361737988404E-19));
#15375=DIRECTION('ref_axis',(8.67361737988404E-19,-2.95954235665401E-42,
1.));
#15376=DIRECTION('center_axis',(1.,-3.41212002678124E-24,-8.67361737988404E-19));
#15377=DIRECTION('ref_axis',(-8.67361737988404E-19,2.95954235665401E-42,
-1.));
#15378=DIRECTION('center_axis',(-0.980042665160198,-4.68316475765215E-14,
0.198787259314315));
#15379=DIRECTION('ref_axis',(0.198787259314315,-2.51180706998856E-11,0.980042665160198));
#15380=DIRECTION('',(-1.,3.41212002678124E-24,8.67361737988404E-19));
#15381=DIRECTION('center_axis',(-8.67361737988404E-19,-1.98523347012726E-23,
-1.));
#15382=DIRECTION('ref_axis',(-1.,3.41212002678124E-24,8.67361737988404E-19));
#15383=DIRECTION('',(3.43796942092352E-24,-1.,-1.98523347012727E-23));
#15384=DIRECTION('',(-3.43796942092352E-24,1.,1.98523347012727E-23));
#15385=DIRECTION('',(-1.,3.41212002678124E-24,8.67361737988404E-19));
#15386=DIRECTION('center_axis',(-5.76441489372891E-24,1.,6.92992146256797E-15));
#15387=DIRECTION('ref_axis',(-1.3010426069826E-18,-6.92992146256797E-15,
1.));
#15388=DIRECTION('',(1.3010426069826E-18,-1.98523347012727E-23,-1.));
#15389=DIRECTION('',(0.198787259314375,-6.79161869718135E-15,0.980042665160185));
#15390=DIRECTION('',(-1.,3.41212002678124E-24,8.67361737988404E-19));
#15391=DIRECTION('center_axis',(-1.3010426069826E-18,-7.17366181720274E-15,
1.));
#15392=DIRECTION('ref_axis',(5.97121004686716E-24,-1.,-7.17366181720274E-15));
#15393=DIRECTION('',(-5.97121004686716E-24,1.,7.17366181720274E-15));
#15394=DIRECTION('',(-1.4550719198321E-15,-1.,-7.17366180396785E-15));
#15395=DIRECTION('center_axis',(-0.980042665160186,1.32348898008484E-23,
0.198787259314375));
#15396=DIRECTION('ref_axis',(0.198787259314375,1.98523347012727E-23,0.980042665160185));
#15397=DIRECTION('center_axis',(1.,-3.41212002678124E-24,1.3010426069826E-18));
#15398=DIRECTION('ref_axis',(1.3010426069826E-18,-1.98523347012726E-23,
-1.));
#15399=DIRECTION('center_axis',(0.,1.,0.));
#15400=DIRECTION('ref_axis',(0.,0.,1.));
#15401=DIRECTION('',(-1.,0.,-5.55111512312578E-17));
#15402=DIRECTION('',(0.,0.,-1.));
#15403=DIRECTION('',(1.,0.,-5.55111512312578E-17));
#15404=DIRECTION('',(0.,0.,-1.));
#15405=DIRECTION('center_axis',(-1.,0.,0.));
#15406=DIRECTION('ref_axis',(0.,0.,1.));
#15407=DIRECTION('',(0.,-1.,0.));
#15408=DIRECTION('',(0.,0.,-1.));
#15409=DIRECTION('',(0.,1.,0.));
#15410=DIRECTION('center_axis',(0.,0.,-1.));
#15411=DIRECTION('ref_axis',(-1.,0.,0.));
#15412=DIRECTION('center_axis',(5.55111512312578E-17,0.,-1.));
#15413=DIRECTION('ref_axis',(-1.,0.,-5.55111512312578E-17));
#15414=DIRECTION('',(0.,0.,-1.));
#15415=DIRECTION('center_axis',(5.55111512312578E-17,0.,1.));
#15416=DIRECTION('ref_axis',(1.,0.,-5.55111512312578E-17));
#15417=DIRECTION('center_axis',(-0.164410656039629,-0.986391978972162,0.));
#15418=DIRECTION('ref_axis',(0.986391978972162,-0.164410656039629,0.));
#15419=DIRECTION('',(0.986391978972162,-0.164410656039629,5.47557543180234E-17));
#15420=DIRECTION('',(0.,0.,-1.));
#15421=DIRECTION('',(-0.986391978972162,0.164410656039629,5.47557543180234E-17));
#15422=DIRECTION('center_axis',(0.,0.,-1.));
#15423=DIRECTION('ref_axis',(-1.,0.,0.));
#15424=DIRECTION('center_axis',(-5.55111512312578E-17,0.,1.));
#15425=DIRECTION('ref_axis',(-1.,-1.011795553209E-15,-5.55111512312578E-17));
#15426=DIRECTION('',(0.,0.,-1.));
#15427=DIRECTION('center_axis',(-5.55111512312578E-17,0.,-1.));
#15428=DIRECTION('ref_axis',(1.,0.,-5.55111512312578E-17));
#15429=DIRECTION('center_axis',(-1.,0.,0.));
#15430=DIRECTION('ref_axis',(0.,0.,1.));
#15431=DIRECTION('',(0.,-1.,0.));
#15432=DIRECTION('',(0.,0.,-1.));
#15433=DIRECTION('',(0.,1.,0.));
#15434=DIRECTION('center_axis',(0.,0.,-1.));
#15435=DIRECTION('ref_axis',(-1.,0.,0.));
#15436=DIRECTION('center_axis',(-5.55111512312578E-17,0.,1.));
#15437=DIRECTION('ref_axis',(-1.,5.31192665434724E-15,-5.55111512312578E-17));
#15438=DIRECTION('',(0.,0.,-1.));
#15439=DIRECTION('center_axis',(-5.55111512312578E-17,0.,-1.));
#15440=DIRECTION('ref_axis',(1.,1.77064221811575E-15,-5.55111512312578E-17));
#15441=DIRECTION('center_axis',(-0.164410656039629,0.986391978972162,0.));
#15442=DIRECTION('ref_axis',(-0.986391978972162,-0.164410656039629,0.));
#15443=DIRECTION('',(-0.986391978972162,-0.164410656039629,-5.47557543180234E-17));
#15444=DIRECTION('',(0.,0.,-1.));
#15445=DIRECTION('',(0.986391978972162,0.164410656039629,-5.47557543180234E-17));
#15446=DIRECTION('center_axis',(0.,0.,-1.));
#15447=DIRECTION('ref_axis',(-1.,0.,0.));
#15448=DIRECTION('center_axis',(5.55111512312578E-17,0.,-1.));
#15449=DIRECTION('ref_axis',(-1.,0.,-5.55111512312578E-17));
#15450=DIRECTION('',(0.,0.,-1.));
#15451=DIRECTION('center_axis',(5.55111512312578E-17,0.,1.));
#15452=DIRECTION('ref_axis',(1.,0.,-5.55111512312578E-17));
#15453=DIRECTION('center_axis',(-1.,0.,0.));
#15454=DIRECTION('ref_axis',(0.,0.,1.));
#15455=DIRECTION('',(0.,-1.,0.));
#15456=DIRECTION('',(0.,0.,-1.));
#15457=DIRECTION('',(0.,1.,0.));
#15458=DIRECTION('center_axis',(0.,-1.,0.));
#15459=DIRECTION('ref_axis',(0.,0.,-1.));
#15460=DIRECTION('',(1.,0.,5.55111512312578E-17));
#15461=DIRECTION('',(0.,0.,-1.));
#15462=DIRECTION('',(-1.,0.,5.55111512312578E-17));
#15463=DIRECTION('center_axis',(1.,0.,0.));
#15464=DIRECTION('ref_axis',(0.,0.,-1.));
#15465=DIRECTION('',(0.,1.,0.));
#15466=DIRECTION('',(0.,-1.,0.));
#15467=DIRECTION('center_axis',(5.55111512312578E-17,0.,1.));
#15468=DIRECTION('ref_axis',(1.,0.,-5.55111512312578E-17));
#15469=DIRECTION('center_axis',(5.55111512312578E-17,0.,-1.));
#15470=DIRECTION('ref_axis',(-1.,0.,-5.55111512312578E-17));
#15471=DIRECTION('center_axis',(-1.,5.97767239540274E-24,-8.67361737988403E-19));
#15472=DIRECTION('ref_axis',(-8.67361737988403E-19,6.61744490042422E-24,
1.));
#15473=DIRECTION('',(6.81131535649133E-24,-1.,6.61744490042422E-24));
#15474=DIRECTION('',(-4.33680868994202E-19,1.98523347012727E-23,1.));
#15475=DIRECTION('',(-6.81131535649133E-24,1.,-6.61744490042422E-24));
#15476=DIRECTION('',(-4.33680868994202E-19,1.98523347012727E-23,1.));
#15477=DIRECTION('',(6.81131535649133E-24,-1.,6.61744490042422E-24));
#15478=DIRECTION('center_axis',(-1.,5.97767239540274E-24,6.50521303491302E-19));
#15479=DIRECTION('ref_axis',(6.50521303491302E-19,-3.88860323850136E-42,
1.));
#15480=DIRECTION('',(-8.67361737988403E-19,-0.164410656039629,0.986391978972162));
#15481=DIRECTION('center_axis',(1.,-5.97767239540274E-24,-6.50521303491302E-19));
#15482=DIRECTION('ref_axis',(6.50521303491302E-19,-3.88860323850136E-42,
1.));
#15483=DIRECTION('',(6.81131535649133E-24,-1.,6.61744490042422E-24));
#15484=DIRECTION('center_axis',(1.,-5.97767239540274E-24,-6.50521303491302E-19));
#15485=DIRECTION('ref_axis',(6.50521303491302E-19,-2.02359110641796E-15,
1.));
#15486=DIRECTION('',(1.51788304147971E-18,-0.164410656039629,-0.986391978972162));
#15487=DIRECTION('center_axis',(-1.,5.97767239540274E-24,6.50521303491302E-19));
#15488=DIRECTION('ref_axis',(6.50521303491302E-19,-3.88860323850136E-42,
1.));
#15489=DIRECTION('center_axis',(-6.50521303491302E-19,-6.61744490042422E-24,
-1.));
#15490=DIRECTION('ref_axis',(-1.,5.97767239540274E-24,6.50521303491302E-19));
#15491=DIRECTION('',(-1.,5.97767239540274E-24,6.50521303491302E-19));
#15492=DIRECTION('',(-6.81131535649133E-24,1.,-6.61744490042422E-24));
#15493=DIRECTION('',(-1.,5.97767239540274E-24,6.50521303491302E-19));
#15494=DIRECTION('center_axis',(6.81131535649133E-24,-1.,6.61744490042422E-24));
#15495=DIRECTION('ref_axis',(8.67361737988403E-19,-6.61744490042422E-24,
-1.));
#15496=DIRECTION('',(0.198787259314375,-6.61744490042422E-24,-0.980042665160185));
#15497=DIRECTION('',(-1.,5.97767239540274E-24,6.50521303491302E-19));
#15498=DIRECTION('center_axis',(6.50521303491302E-19,6.61744490042422E-24,
1.));
#15499=DIRECTION('ref_axis',(1.,-5.97767239540274E-24,-6.50521303491302E-19));
#15500=DIRECTION('',(6.81131535649133E-24,-1.,6.61744490042422E-24));
#15501=DIRECTION('',(-1.,5.97767239540274E-24,6.50521303491302E-19));
#15502=DIRECTION('center_axis',(-1.,5.97767239540274E-24,6.50521303491302E-19));
#15503=DIRECTION('ref_axis',(6.50521303491302E-19,-3.88860323850136E-42,
1.));
#15504=DIRECTION('center_axis',(-0.980042665160172,-3.50952492787524E-14,
-0.198787259314441));
#15505=DIRECTION('ref_axis',(0.198787259314441,-1.6456332591569E-11,-0.980042665160172));
#15506=DIRECTION('',(-1.,5.97767239540274E-24,6.50521303491302E-19));
#15507=DIRECTION('center_axis',(-1.0842021724855E-19,0.986391978972162,
0.16441065603963));
#15508=DIRECTION('ref_axis',(-6.50521303491303E-19,-0.164410656039629,0.986391978972162));
#15509=DIRECTION('',(-0.196186965810001,-0.161215582689263,0.967222937250987));
#15510=DIRECTION('',(-1.,5.97767239540274E-24,6.50521303491302E-19));
#15511=DIRECTION('center_axis',(-1.,5.97767239540274E-24,6.50521303491302E-19));
#15512=DIRECTION('ref_axis',(6.50521303491302E-19,-3.88860323850136E-42,
1.));
#15513=DIRECTION('center_axis',(0.980042665160175,3.79396694343426E-14,
0.198787259314425));
#15514=DIRECTION('ref_axis',(0.198787259314425,3.87086750237462E-12,-0.980042665160175));
#15515=DIRECTION('',(-1.,5.97767239540274E-24,6.50521303491302E-19));
#15516=DIRECTION('center_axis',(6.50521303491302E-19,6.61744490042422E-24,
1.));
#15517=DIRECTION('ref_axis',(1.,-5.97767239540274E-24,-6.50521303491302E-19));
#15518=DIRECTION('',(6.81131535649133E-24,-1.,6.61744490042422E-24));
#15519=DIRECTION('',(-1.,5.97767239540274E-24,6.50521303491302E-19));
#15520=DIRECTION('center_axis',(-1.,5.97767239540274E-24,6.50521303491302E-19));
#15521=DIRECTION('ref_axis',(6.50521303491302E-19,-3.88860323850136E-42,
1.));
#15522=DIRECTION('center_axis',(0.980042665160169,-9.74657025123624E-14,
0.198787259314457));
#15523=DIRECTION('ref_axis',(0.198787259314457,9.35920069890102E-12,-0.980042665160169));
#15524=DIRECTION('',(-1.,5.97767239540274E-24,6.50521303491302E-19));
#15525=DIRECTION('center_axis',(-3.79470760369927E-19,-0.986391978972162,
0.164410656039629));
#15526=DIRECTION('ref_axis',(1.51788304147971E-18,-0.164410656039629,-0.986391978972162));
#15527=DIRECTION('',(0.196186965810001,-0.161215582689263,-0.967222937250987));
#15528=DIRECTION('',(-1.,5.97767239540274E-24,6.50521303491302E-19));
#15529=DIRECTION('center_axis',(-1.,5.97767239540274E-24,6.50521303491302E-19));
#15530=DIRECTION('ref_axis',(6.50521303491302E-19,-3.88860323850136E-42,
1.));
#15531=DIRECTION('center_axis',(-0.980042665160186,-2.44983071264037E-14,
-0.198787259314374));
#15532=DIRECTION('ref_axis',(0.198787259314374,-1.03406121780998E-11,-0.980042665160186));
#15533=DIRECTION('',(-1.,5.97767239540274E-24,6.50521303491302E-19));
#15534=DIRECTION('center_axis',(6.50521303491302E-19,6.61744490042422E-24,
1.));
#15535=DIRECTION('ref_axis',(1.,-5.97767239540274E-24,-6.50521303491302E-19));
#15536=DIRECTION('',(6.81131535649133E-24,-1.,6.61744490042422E-24));
#15537=DIRECTION('',(-1.,5.97767239540274E-24,6.50521303491302E-19));
#15538=DIRECTION('center_axis',(-6.81131535649133E-24,1.,-6.61744490042422E-24));
#15539=DIRECTION('ref_axis',(-8.67361737988403E-19,6.61744490042422E-24,
1.));
#15540=DIRECTION('',(-0.198787259314375,6.61744490042422E-24,0.980042665160185));
#15541=DIRECTION('center_axis',(-0.980042665160186,4.96308367531816E-24,
-0.198787259314375));
#15542=DIRECTION('ref_axis',(-0.198787259314375,6.61744490042422E-24,0.980042665160185));
#15543=DIRECTION('center_axis',(1.08050467514739E-23,1.,-1.32348898008484E-23));
#15544=DIRECTION('ref_axis',(3.46944695195361E-18,1.32348898008484E-23,
1.));
#15545=DIRECTION('',(-0.198787259314375,1.98523347012726E-23,0.980042665160185));
#15546=DIRECTION('',(-1.,-1.07791973573316E-23,-1.30104260698261E-18));
#15547=DIRECTION('',(-3.46944695195361E-18,-1.32348898008484E-23,-1.));
#15548=DIRECTION('',(-1.,-1.07791973573316E-23,-1.30104260698261E-18));
#15549=DIRECTION('center_axis',(-1.3010426069826E-18,1.32348898008484E-23,
1.));
#15550=DIRECTION('ref_axis',(1.,1.07791973573316E-23,1.3010426069826E-18));
#15551=DIRECTION('',(-1.08050467514739E-23,-1.,-1.32348898008484E-23));
#15552=DIRECTION('',(-1.,-1.07791973573316E-23,-1.30104260698261E-18));
#15553=DIRECTION('',(1.08050467514739E-23,1.,1.32348898008484E-23));
#15554=DIRECTION('center_axis',(-1.,-1.07791973573316E-23,-1.3010426069826E-18));
#15555=DIRECTION('ref_axis',(-1.3010426069826E-18,-1.40241950309628E-41,
1.));
#15556=DIRECTION('center_axis',(-0.980042665160171,3.72032431477704E-14,
-0.198787259314447));
#15557=DIRECTION('ref_axis',(0.198787259314447,2.49978107929975E-11,-0.980042665160171));
#15558=DIRECTION('',(-1.,-1.07791973573316E-23,-1.30104260698261E-18));
#15559=DIRECTION('center_axis',(1.,1.07791973573316E-23,1.3010426069826E-18));
#15560=DIRECTION('ref_axis',(1.30104260698261E-18,1.40241950309628E-41,
-1.));
#15561=DIRECTION('center_axis',(4.87890977618476E-19,-0.986391978972162,
0.164410656039629));
#15562=DIRECTION('ref_axis',(-3.46944695195361E-18,-0.164410656039629,-0.986391978972162));
#15563=DIRECTION('',(0.196186965810001,-0.161215582689263,-0.967222937250987));
#15564=DIRECTION('',(-1.,-1.07791973573316E-23,-1.30104260698261E-18));
#15565=DIRECTION('',(3.46944695195361E-18,0.164410656039629,0.986391978972162));
#15566=DIRECTION('center_axis',(-1.,-1.07791973573316E-23,-1.3010426069826E-18));
#15567=DIRECTION('ref_axis',(-1.3010426069826E-18,-1.40241950309628E-41,
1.));
#15568=DIRECTION('center_axis',(0.98004266516019,3.28754198991703E-14,0.198787259314354));
#15569=DIRECTION('ref_axis',(0.198787259314354,8.48405160975645E-13,-0.98004266516019));
#15570=DIRECTION('',(-1.,-1.07791973573316E-23,-1.30104260698261E-18));
#15571=DIRECTION('center_axis',(-1.,-1.07791973573316E-23,-1.3010426069826E-18));
#15572=DIRECTION('ref_axis',(1.3010426069826E-18,1.01179555320898E-15,-1.));
#15573=DIRECTION('center_axis',(-1.3010426069826E-18,1.32348898008484E-23,
1.));
#15574=DIRECTION('ref_axis',(1.,1.07791973573316E-23,1.3010426069826E-18));
#15575=DIRECTION('',(-1.08050467514739E-23,-1.,-1.32348898008484E-23));
#15576=DIRECTION('',(-1.,-1.07791973573316E-23,-1.30104260698261E-18));
#15577=DIRECTION('',(1.08050467514739E-23,1.,1.32348898008484E-23));
#15578=DIRECTION('center_axis',(-1.,-1.07791973573316E-23,-1.3010426069826E-18));
#15579=DIRECTION('ref_axis',(-1.3010426069826E-18,-1.40241950309628E-41,
1.));
#15580=DIRECTION('center_axis',(0.980042665160196,-3.01322847342843E-14,
0.198787259314322));
#15581=DIRECTION('ref_axis',(0.198787259314322,9.80607162696455E-12,-0.980042665160196));
#15582=DIRECTION('',(-1.,-1.07791973573316E-23,-1.30104260698261E-18));
#15583=DIRECTION('center_axis',(-1.,-1.07791973573316E-23,-1.3010426069826E-18));
#15584=DIRECTION('ref_axis',(1.3010426069826E-18,1.77064221811572E-15,-1.));
#15585=DIRECTION('center_axis',(5.42101086242751E-19,0.986391978972162,
0.164410656039629));
#15586=DIRECTION('ref_axis',(2.16840434497101E-18,-0.164410656039629,0.986391978972162));
#15587=DIRECTION('',(-0.196186965810001,-0.161215582689263,0.967222937250987));
#15588=DIRECTION('',(-1.,-1.07791973573316E-23,-1.30104260698261E-18));
#15589=DIRECTION('',(-2.168404344971E-18,0.164410656039629,-0.986391978972162));
#15590=DIRECTION('center_axis',(-1.,-1.07791973573316E-23,-1.3010426069826E-18));
#15591=DIRECTION('ref_axis',(-1.3010426069826E-18,-1.40241950309628E-41,
1.));
#15592=DIRECTION('center_axis',(-0.980042665160224,1.39583377813246E-13,
-0.198787259314183));
#15593=DIRECTION('ref_axis',(0.198787259314183,2.0130592482984E-11,-0.980042665160224));
#15594=DIRECTION('',(-1.,-1.07791973573316E-23,-1.30104260698261E-18));
#15595=DIRECTION('center_axis',(1.,1.07791973573316E-23,1.3010426069826E-18));
#15596=DIRECTION('ref_axis',(1.3010426069826E-18,1.40241950309628E-41,-1.));
#15597=DIRECTION('center_axis',(-1.3010426069826E-18,1.32348898008484E-23,
1.));
#15598=DIRECTION('ref_axis',(1.,1.07791973573316E-23,1.3010426069826E-18));
#15599=DIRECTION('',(-1.08050467514739E-23,-1.,-1.32348898008484E-23));
#15600=DIRECTION('',(-1.,-1.07791973573316E-23,-1.30104260698261E-18));
#15601=DIRECTION('',(1.08050467514739E-23,1.,1.32348898008484E-23));
#15602=DIRECTION('center_axis',(-1.08050467514739E-23,-1.,1.32348898008484E-23));
#15603=DIRECTION('ref_axis',(-3.46944695195361E-18,-1.32348898008484E-23,
-1.));
#15604=DIRECTION('',(0.198787259314375,-1.98523347012726E-23,-0.980042665160185));
#15605=DIRECTION('',(-1.,-1.07791973573316E-23,-1.30104260698261E-18));
#15606=DIRECTION('',(-3.46944695195361E-18,-1.32348898008484E-23,-1.));
#15607=DIRECTION('center_axis',(1.3010426069826E-18,-1.32348898008484E-23,
-1.));
#15608=DIRECTION('ref_axis',(-1.,-1.07791973573316E-23,-1.3010426069826E-18));
#15609=DIRECTION('',(1.08050467514739E-23,1.,1.32348898008484E-23));
#15610=DIRECTION('',(-1.08050467514739E-23,-1.,-1.32348898008484E-23));
#15611=DIRECTION('center_axis',(1.,1.07791973573316E-23,-3.46944695195361E-18));
#15612=DIRECTION('ref_axis',(-3.46944695195361E-18,-1.32348898008484E-23,
-1.));
#15613=DIRECTION('center_axis',(-0.980042665160186,-1.48892510259545E-23,
-0.198787259314375));
#15614=DIRECTION('ref_axis',(-0.198787259314375,1.98523347012726E-23,0.980042665160185));
#15615=DIRECTION('center_axis',(-0.980042665160186,5.16987882845642E-23,
-0.198787259314375));
#15616=DIRECTION('ref_axis',(-0.198787259314375,-1.98523347012727E-23,0.980042665160186));
#15617=DIRECTION('',(4.79764755280756E-23,-1.,1.32348898008484E-23));
#15618=DIRECTION('',(-0.198787259314375,-1.98523347012727E-23,0.980042665160185));
#15619=DIRECTION('',(-4.79764755280756E-23,1.,-1.32348898008484E-23));
#15620=DIRECTION('',(0.198787259314375,1.98523347012727E-23,-0.980042665160185));
#15621=DIRECTION('',(4.79764755280756E-23,-1.,1.32348898008484E-23));
#15622=DIRECTION('center_axis',(-0.980042665160192,-1.1109697417788E-14,
-0.198787259314345));
#15623=DIRECTION('ref_axis',(0.198787259314345,-8.89157906913263E-12,-0.980042665160192));
#15624=DIRECTION('',(-0.196186965810001,-0.161215582689263,0.967222937250987));
#15625=DIRECTION('center_axis',(0.980042665160184,-1.0212903229267E-14,
0.198787259314383));
#15626=DIRECTION('ref_axis',(0.198787259314383,-1.20235415482955E-11,-0.980042665160184));
#15627=DIRECTION('',(4.79764755280756E-23,-1.,1.32348898008484E-23));
#15628=DIRECTION('center_axis',(0.980042665160188,1.68386297044527E-14,
0.198787259314362));
#15629=DIRECTION('ref_axis',(0.198787259314362,5.91971428266698E-13,-0.980042665160188));
#15630=DIRECTION('',(0.196186965810001,-0.161215582689263,-0.967222937250987));
#15631=DIRECTION('center_axis',(-0.980042665160183,2.8030621177186E-14,
-0.198787259314389));
#15632=DIRECTION('ref_axis',(0.198787259314389,-8.39289157340378E-12,-0.980042665160183));
#15633=DIRECTION('center_axis',(0.389639990836698,6.61744490042423E-24,
-0.920967251068559));
#15634=DIRECTION('ref_axis',(-0.920967251068559,5.55244986176219E-23,-0.389639990836698));
#15635=DIRECTION('',(-0.920967251068559,6.70016296167952E-23,-0.389639990836698));
#15636=DIRECTION('',(-4.79764755280756E-23,1.,-1.32348898008484E-23));
#15637=DIRECTION('',(-0.920967251068559,6.70016296167952E-23,-0.389639990836698));
#15638=DIRECTION('center_axis',(4.79764755280756E-23,-1.,-3.63959469523332E-23));
#15639=DIRECTION('ref_axis',(-1.11022302462516E-16,3.63959469523332E-23,
-1.));
#15640=DIRECTION('',(0.198787259314375,1.32348898008484E-23,-0.980042665160185));
#15641=DIRECTION('',(-0.920967251068559,6.70016296167952E-23,-0.389639990836698));
#15642=DIRECTION('center_axis',(-0.389639990836698,-9.92616735063634E-24,
0.920967251068559));
#15643=DIRECTION('ref_axis',(0.920967251068559,-6.70016296167952E-23,0.389639990836698));
#15644=DIRECTION('',(4.79764755280756E-23,-1.,1.32348898008484E-23));
#15645=DIRECTION('',(-0.920967251068559,6.70016296167952E-23,-0.389639990836698));
#15646=DIRECTION('center_axis',(-0.920967251068559,6.70016296167952E-23,
-0.389639990836698));
#15647=DIRECTION('ref_axis',(-0.389639990836698,5.58402704648591E-37,0.920967251068559));
#15648=DIRECTION('center_axis',(-0.980042665160215,1.23232182126544E-13,
-0.198787259314232));
#15649=DIRECTION('ref_axis',(0.198787259314232,3.04736265298492E-11,-0.980042665160214));
#15650=DIRECTION('',(-0.920967251068559,6.70016296167952E-23,-0.389639990836698));
#15651=DIRECTION('center_axis',(-0.0640609665127368,0.986391978972162,0.151416829939196));
#15652=DIRECTION('ref_axis',(5.5015443345664E-17,-0.151728482244601,0.988422211241608));
#15653=DIRECTION('',(-0.196186965810001,-0.161215582689263,0.967222937250987));
#15654=DIRECTION('',(-0.920967251068559,6.70016296167952E-23,-0.389639990836698));
#15655=DIRECTION('center_axis',(-0.920967251068559,6.70016296167952E-23,
-0.389639990836698));
#15656=DIRECTION('ref_axis',(-0.389639990836698,1.72143967328141E-37,0.920967251068559));
#15657=DIRECTION('center_axis',(0.980042665160173,5.74370301447608E-14,
0.198787259314435));
#15658=DIRECTION('ref_axis',(0.198787259314435,-7.91172988590792E-12,-0.980042665160173));
#15659=DIRECTION('',(-0.920967251068559,6.70016296167952E-23,-0.389639990836698));
#15660=DIRECTION('center_axis',(-0.389639990836698,-9.92616735063634E-24,
0.920967251068559));
#15661=DIRECTION('ref_axis',(0.920967251068559,-6.70016296167952E-23,0.389639990836698));
#15662=DIRECTION('',(4.79764755280756E-23,-1.,1.32348898008484E-23));
#15663=DIRECTION('',(-0.920967251068559,6.70016296167952E-23,-0.389639990836698));
#15664=DIRECTION('center_axis',(-0.920967251068559,6.70016296167952E-23,
-0.389639990836698));
#15665=DIRECTION('ref_axis',(-0.389639990836698,1.72143967328141E-37,0.920967251068559));
#15666=DIRECTION('center_axis',(0.980042665160181,-1.32514529503713E-14,
0.198787259314395));
#15667=DIRECTION('ref_axis',(0.198787259314395,2.44975507155414E-12,-0.980042665160181));
#15668=DIRECTION('',(-0.920967251068559,6.70016296167952E-23,-0.389639990836698));
#15669=DIRECTION('center_axis',(-0.0640609665127368,-0.986391978972162,
0.151416829939196));
#15670=DIRECTION('ref_axis',(-5.50609226423701E-17,-0.151728482244601,-0.988422211241608));
#15671=DIRECTION('',(0.196186965810001,-0.161215582689263,-0.967222937250987));
#15672=DIRECTION('',(-0.920967251068559,6.70016296167952E-23,-0.389639990836698));
#15673=DIRECTION('center_axis',(-0.920967251068559,6.70016296167952E-23,
-0.389639990836698));
#15674=DIRECTION('ref_axis',(-0.389639990836698,5.58402704648591E-37,0.920967251068559));
#15675=DIRECTION('center_axis',(-0.980042665160197,-5.27568195326752E-14,
-0.198787259314317));
#15676=DIRECTION('ref_axis',(0.198787259314317,-5.60688280667672E-11,-0.980042665160197));
#15677=DIRECTION('',(-0.920967251068559,6.70016296167952E-23,-0.389639990836698));
#15678=DIRECTION('center_axis',(-0.389639990836698,-9.92616735063634E-24,
0.920967251068559));
#15679=DIRECTION('ref_axis',(0.920967251068559,-6.70016296167952E-23,0.389639990836698));
#15680=DIRECTION('',(4.79764755280756E-23,-1.,1.32348898008484E-23));
#15681=DIRECTION('',(-0.920967251068559,6.70016296167952E-23,-0.389639990836698));
#15682=DIRECTION('center_axis',(-4.79764755280756E-23,1.,3.63959469523332E-23));
#15683=DIRECTION('ref_axis',(1.11022302462516E-16,-3.63959469523332E-23,
1.));
#15684=DIRECTION('',(-0.198787259314375,-1.32348898008484E-23,0.980042665160185));
#15685=DIRECTION('center_axis',(-0.980042665160186,4.30133918527574E-23,
-0.198787259314375));
#15686=DIRECTION('ref_axis',(-0.198787259314375,-1.32348898008484E-23,0.980042665160185));
#15687=DIRECTION('center_axis',(1.28626585251996E-22,-1.,7.63278329429795E-17));
#15688=DIRECTION('ref_axis',(2.64697796016969E-23,-7.63278329429795E-17,
-1.));
#15689=DIRECTION('',(1.02125158911203E-14,-1.38777878078145E-17,-1.));
#15690=DIRECTION('',(1.,-1.48065329646992E-22,-3.97046694025453E-23));
#15691=DIRECTION('center_axis',(1.28626585251996E-22,-1.,4.85722573273505E-17));
#15692=DIRECTION('ref_axis',(-3.57010491314168E-39,-4.85722573273505E-17,
-1.));
#15693=DIRECTION('',(0.164410656039619,6.93889390390723E-18,0.986391978972164));
#15694=DIRECTION('center_axis',(-1.28626585251996E-22,1.,-4.85722573273505E-17));
#15695=DIRECTION('ref_axis',(-3.57010491314211E-39,-4.85722573273506E-17,
-1.));
#15696=DIRECTION('',(1.,-1.9935052762528E-22,1.0378694093902E-14));
#15697=DIRECTION('center_axis',(-1.28626585251996E-22,1.,-4.85722573273505E-17));
#15698=DIRECTION('ref_axis',(3.57010491314192E-39,4.85722573273505E-17,
1.));
#15699=DIRECTION('',(0.16441065603964,-2.77555756156289E-17,-0.986391978972161));
#15700=DIRECTION('center_axis',(1.28626585251996E-22,-1.,4.85722573273505E-17));
#15701=DIRECTION('ref_axis',(3.57010491314168E-39,4.85722573273505E-17,
1.));
#15702=DIRECTION('',(1.,-1.48065329646992E-22,-3.97046694025453E-23));
#15703=DIRECTION('',(-1.02125158911203E-14,1.38777878078145E-17,1.));
#15704=DIRECTION('',(-1.,1.72467157717306E-22,-1.0198899135044E-14));
#15705=DIRECTION('center_axis',(1.0198899135044E-14,-1.38777878078145E-17,
-1.));
#15706=DIRECTION('ref_axis',(-1.,1.72467157717306E-22,-1.0198899135044E-14));
#15707=DIRECTION('',(-1.23249911270401E-22,1.,1.38777878078144E-17));
#15708=DIRECTION('',(-1.,-1.00447013890157E-14,-1.01988991218091E-14));
#15709=DIRECTION('',(-1.23249911270401E-22,1.,1.38777878078144E-17));
#15710=DIRECTION('center_axis',(-1.,1.44343016890503E-22,-1.02125158911203E-14));
#15711=DIRECTION('ref_axis',(-1.02125158911203E-14,1.38777878078145E-17,
1.));
#15712=DIRECTION('',(-1.23249911270401E-22,1.,1.38777878078144E-17));
#15713=DIRECTION('',(-7.22133935627488E-15,0.707106781186548,0.707106781186547));
#15714=DIRECTION('center_axis',(3.97046694025453E-23,1.38777878078145E-17,
1.));
#15715=DIRECTION('ref_axis',(1.,-1.48065329646992E-22,-3.97046694025453E-23));
#15716=DIRECTION('',(-1.23249911270401E-22,1.,1.38777878078144E-17));
#15717=DIRECTION('',(1.,-1.54197836190994E-16,-3.97046694025453E-23));
#15718=DIRECTION('center_axis',(-1.23249911270401E-22,1.,1.38777878078144E-17));
#15719=DIRECTION('ref_axis',(3.42087223188502E-39,-1.38777878078144E-17,
1.));
#15720=DIRECTION('',(-1.23249911270401E-22,1.,1.38777878078144E-17));
#15721=DIRECTION('center_axis',(-2.13533570892991E-15,-0.70710678118654,
0.707106781186555));
#15722=DIRECTION('ref_axis',(-5.92260635202438E-13,-0.707106781186555,-0.70710678118654));
#15723=DIRECTION('center_axis',(0.986391978972161,4.33680868994202E-18,
0.16441065603964));
#15724=DIRECTION('ref_axis',(0.16441065603964,-2.77555756156289E-17,-0.986391978972161));
#15725=DIRECTION('',(-1.23249911270401E-22,1.,1.38777878078144E-17));
#15726=DIRECTION('',(0.117049568370797,-0.702246181386631,-0.702246181386631));
#15727=DIRECTION('center_axis',(-1.23249911270401E-22,1.,1.38777878078144E-17));
#15728=DIRECTION('ref_axis',(3.42087223188512E-39,-1.38777878078144E-17,
1.));
#15729=DIRECTION('',(-1.23249911270401E-22,1.,1.38777878078144E-17));
#15730=DIRECTION('center_axis',(5.7517460173195E-15,0.70710678118654,-0.707106781186555));
#15731=DIRECTION('ref_axis',(1.26621527472326E-13,0.707106781186555,0.70710678118654));
#15732=DIRECTION('center_axis',(-1.0378694093902E-14,1.38777878078145E-17,
1.));
#15733=DIRECTION('ref_axis',(1.,-1.9935052762528E-22,1.0378694093902E-14));
#15734=DIRECTION('',(-1.23249911270401E-22,1.,1.38777878078144E-17));
#15735=DIRECTION('',(1.,1.02244962936934E-14,1.0378694093902E-14));
#15736=DIRECTION('center_axis',(-1.23249911270401E-22,1.,1.38777878078144E-17));
#15737=DIRECTION('ref_axis',(3.42087223188522E-39,-1.38777878078144E-17,
1.));
#15738=DIRECTION('',(-1.23249911270401E-22,1.,1.38777878078144E-17));
#15739=DIRECTION('center_axis',(-1.20786666363705E-14,0.70710678118656,
-0.707106781186535));
#15740=DIRECTION('ref_axis',(5.92625417861852E-14,0.707106781186535,0.70710678118656));
#15741=DIRECTION('center_axis',(-0.986391978972164,6.93889390390723E-18,
0.164410656039619));
#15742=DIRECTION('ref_axis',(0.164410656039619,2.77555756156289E-17,0.986391978972164));
#15743=DIRECTION('',(-1.23249911270401E-22,1.,1.38777878078144E-17));
#15744=DIRECTION('',(0.117049568370782,0.702246181386633,0.702246181386632));
#15745=DIRECTION('center_axis',(-1.23249911270401E-22,1.,1.38777878078144E-17));
#15746=DIRECTION('ref_axis',(3.42087223188502E-39,-1.38777878078144E-17,
1.));
#15747=DIRECTION('',(-1.23249911270401E-22,1.,1.38777878078144E-17));
#15748=DIRECTION('center_axis',(-2.31004499420576E-14,-0.707106781186537,
0.707106781186558));
#15749=DIRECTION('ref_axis',(2.54103796788768E-13,-0.707106781186558,-0.707106781186537));
#15750=DIRECTION('center_axis',(3.97046694025453E-23,1.38777878078145E-17,
1.));
#15751=DIRECTION('ref_axis',(1.,-1.48065329646992E-22,-3.97046694025453E-23));
#15752=DIRECTION('',(-1.23249911270401E-22,1.,1.38777878078144E-17));
#15753=DIRECTION('',(1.,-1.54197836190994E-16,-3.97046694025453E-23));
#15754=DIRECTION('center_axis',(1.,-1.44343016890503E-22,1.02125158911203E-14));
#15755=DIRECTION('ref_axis',(1.02125158911203E-14,-1.38777878078145E-17,
-1.));
#15756=DIRECTION('',(7.22133935627488E-15,-0.707106781186548,-0.707106781186547));
#15757=DIRECTION('center_axis',(-1.09034144081742E-16,-0.707106781186547,
0.707106781186548));
#15758=DIRECTION('ref_axis',(1.19114008210604E-22,-0.707106781186548,-0.707106781186547));
#15759=DIRECTION('center_axis',(1.2516276642837E-22,1.,7.63278329429795E-17));
#15760=DIRECTION('ref_axis',(-3.08395300977893E-16,-7.63278329429795E-17,
1.));
#15761=DIRECTION('',(9.90412056201823E-15,-1.38777878078144E-16,1.));
#15762=DIRECTION('',(-1.,-5.28361616268246E-23,9.89050390189491E-15));
#15763=DIRECTION('',(-9.90412056201823E-15,1.38777878078144E-16,-1.));
#15764=DIRECTION('',(1.,6.97416653958771E-23,3.08395271199391E-16));
#15765=DIRECTION('center_axis',(1.2516276643693E-22,1.,4.85722573273506E-17));
#15766=DIRECTION('ref_axis',(-3.47396462810159E-39,4.85722573273506E-17,
-1.));
#15767=DIRECTION('',(0.16441065603964,-1.2490009027033E-16,0.986391978972161));
#15768=DIRECTION('center_axis',(-1.2516276643693E-22,-1.,-4.85722573273506E-17));
#15769=DIRECTION('ref_axis',(-3.47396462810152E-39,4.85722573273506E-17,
-1.));
#15770=DIRECTION('',(1.,1.18907213054498E-23,-1.00702988590986E-14));
#15771=DIRECTION('center_axis',(-1.2516276643693E-22,-1.,-4.85722573273506E-17));
#15772=DIRECTION('ref_axis',(3.47396462810149E-39,-4.85722573273506E-17,
1.));
#15773=DIRECTION('',(0.164410656039619,1.04083408558608E-16,-0.986391978972164));
#15774=DIRECTION('center_axis',(1.2516276643693E-22,1.,4.85722573273506E-17));
#15775=DIRECTION('ref_axis',(3.47396462810128E-39,-4.85722573273506E-17,
1.));
#15776=DIRECTION('',(1.,6.97416653958771E-23,3.08395271199391E-16));
#15777=DIRECTION('center_axis',(9.89050390189491E-15,-1.38777878078144E-17,
1.));
#15778=DIRECTION('ref_axis',(1.,5.28361616268246E-23,-9.89050390189491E-15));
#15779=DIRECTION('',(-1.26041645837768E-22,-1.,1.38777878078145E-17));
#15780=DIRECTION('',(1.,1.00447015947769E-14,-9.89050390024055E-15));
#15781=DIRECTION('',(-1.26041645837768E-22,-1.,1.38777878078145E-17));
#15782=DIRECTION('center_axis',(-1.,2.37814426108995E-23,9.90412057029004E-15));
#15783=DIRECTION('ref_axis',(9.90412057029004E-15,-1.38777878078144E-17,
1.));
#15784=DIRECTION('',(7.00327079679616E-15,-0.707106781186548,0.707106781186548));
#15785=DIRECTION('',(-1.26041645837768E-22,-1.,1.38777878078145E-17));
#15786=DIRECTION('center_axis',(3.08395271199391E-16,1.38777878078144E-17,
-1.));
#15787=DIRECTION('ref_axis',(-1.,-6.97416653958771E-23,-3.08395271199391E-16));
#15788=DIRECTION('',(-1.,1.54197564307067E-16,-3.0839526954503E-16));
#15789=DIRECTION('',(-1.26041645837768E-22,-1.,1.38777878078145E-17));
#15790=DIRECTION('center_axis',(-1.26041645837768E-22,-1.,1.38777878078145E-17));
#15791=DIRECTION('ref_axis',(-1.74917921588424E-39,-1.38777878078145E-17,
-1.));
#15792=DIRECTION('center_axis',(-1.54326535327199E-14,-0.707106781186548,
-0.707106781186547));
#15793=DIRECTION('ref_axis',(-1.3938976131661E-12,0.707106781186547,-0.707106781186548));
#15794=DIRECTION('',(-1.26041645837768E-22,-1.,1.38777878078145E-17));
#15795=DIRECTION('center_axis',(0.986391978972161,-2.60208521396521E-18,
-0.16441065603964));
#15796=DIRECTION('ref_axis',(-0.16441065603964,2.83749245036362E-35,-0.986391978972161));
#15797=DIRECTION('',(-0.117049568370797,0.702246181386631,-0.702246181386631));
#15798=DIRECTION('',(-1.26041645837768E-22,-1.,1.38777878078145E-17));
#15799=DIRECTION('center_axis',(-1.26041645837768E-22,-1.,1.38777878078145E-17));
#15800=DIRECTION('ref_axis',(-1.74917921588424E-39,-1.38777878078144E-17,
-1.));
#15801=DIRECTION('center_axis',(1.4379365043299E-15,0.707106781186542,0.707106781186553));
#15802=DIRECTION('ref_axis',(1.34200807773731E-12,-0.707106781186553,0.707106781186542));
#15803=DIRECTION('',(-1.26041645837768E-22,-1.,1.38777878078145E-17));
#15804=DIRECTION('center_axis',(-1.00702988590986E-14,1.38777878078144E-17,
-1.));
#15805=DIRECTION('ref_axis',(-1.,-1.18907213054498E-23,1.00702988590986E-14));
#15806=DIRECTION('',(-1.,-1.02244964855993E-14,1.00702988557898E-14));
#15807=DIRECTION('',(-1.26041645837768E-22,-1.,1.38777878078145E-17));
#15808=DIRECTION('center_axis',(-1.26041645837768E-22,-1.,1.38777878078145E-17));
#15809=DIRECTION('ref_axis',(-1.74917921588424E-39,-1.38777878078145E-17,
-1.));
#15810=DIRECTION('center_axis',(1.29414285389683E-14,0.707106781186545,
0.70710678118655));
#15811=DIRECTION('ref_axis',(1.69540060192356E-13,-0.70710678118655,0.707106781186545));
#15812=DIRECTION('',(-1.26041645837768E-22,-1.,1.38777878078145E-17));
#15813=DIRECTION('center_axis',(-0.986391978972164,2.60208521396522E-18,
-0.164410656039619));
#15814=DIRECTION('ref_axis',(-0.164410656039619,2.08166817117217E-17,0.986391978972164));
#15815=DIRECTION('',(-0.117049568370783,-0.702246181386632,0.702246181386632));
#15816=DIRECTION('',(-1.26041645837768E-22,-1.,1.38777878078145E-17));
#15817=DIRECTION('center_axis',(-1.26041645837768E-22,-1.,1.38777878078145E-17));
#15818=DIRECTION('ref_axis',(-1.74917921588424E-39,-1.38777878078145E-17,
-1.));
#15819=DIRECTION('center_axis',(1.94121428084521E-14,-0.707106781186553,
-0.707106781186542));
#15820=DIRECTION('ref_axis',(6.99433665140334E-13,0.707106781186542,-0.707106781186553));
#15821=DIRECTION('',(-1.26041645837768E-22,-1.,1.38777878078145E-17));
#15822=DIRECTION('center_axis',(3.08395271199391E-16,1.38777878078144E-17,
-1.));
#15823=DIRECTION('ref_axis',(-1.,-6.97416653958771E-23,-3.08395271199391E-16));
#15824=DIRECTION('',(-1.,1.54197564307067E-16,-3.0839526954503E-16));
#15825=DIRECTION('',(-1.26041645837768E-22,-1.,1.38777878078145E-17));
#15826=DIRECTION('center_axis',(1.,-2.37814426108995E-23,-9.90412057029004E-15));
#15827=DIRECTION('ref_axis',(-9.90412057029004E-15,1.38777878078144E-17,
-1.));
#15828=DIRECTION('',(-7.00327079679616E-15,0.707106781186548,-0.707106781186548));
#15829=DIRECTION('center_axis',(1.09034183786412E-16,-0.707106781186548,
-0.707106781186547));
#15830=DIRECTION('ref_axis',(4.63221142954057E-23,0.707106781186547,-0.707106781186548));
#15831=DIRECTION('center_axis',(1.,-3.54987407349455E-30,-1.04916075827077E-14));
#15832=DIRECTION('ref_axis',(-1.04916075827077E-14,-9.86076131526265E-32,
-1.));
#15833=DIRECTION('',(1.04916075827077E-14,3.82856869892695E-16,1.));
#15834=DIRECTION('',(0.,-1.,3.46944695195361E-16));
#15835=DIRECTION('',(1.04916075827077E-14,3.82856869892695E-16,1.));
#15836=DIRECTION('',(0.,-1.,3.46944695195361E-16));
#15837=DIRECTION('center_axis',(0.,-3.46944695195361E-16,-1.));
#15838=DIRECTION('ref_axis',(0.,1.,-3.46944695195361E-16));
#15839=DIRECTION('',(1.,0.,0.));
#15840=DIRECTION('',(0.,-1.,3.46944695195361E-16));
#15841=DIRECTION('',(1.,0.,0.));
#15842=DIRECTION('center_axis',(0.,-1.,3.46944695195361E-16));
#15843=DIRECTION('ref_axis',(0.,-3.46944695195361E-16,-1.));
#15844=DIRECTION('center_axis',(4.93038065763132E-32,1.,-3.82856869892695E-16));
#15845=DIRECTION('ref_axis',(0.,3.82856869892695E-16,1.));
#15846=DIRECTION('',(0.,-1.,3.46944695195361E-16));
#15847=DIRECTION('center_axis',(4.93038065763132E-32,1.,-3.82856869892695E-16));
#15848=DIRECTION('ref_axis',(1.88763010596022E-47,3.82856869892695E-16,
1.));
#15849=DIRECTION('center_axis',(-1.,3.54987407349455E-30,1.06581410364015E-14));
#15850=DIRECTION('ref_axis',(1.06581410364015E-14,1.97215226305253E-31,
1.));
#15851=DIRECTION('',(-1.06581410364015E-14,-3.82856869892696E-16,-1.));
#15852=DIRECTION('',(0.,-1.,3.46944695195361E-16));
#15853=DIRECTION('',(-1.06581410364015E-14,-3.82856869892696E-16,-1.));
#15854=DIRECTION('center_axis',(0.,-1.,3.46944695195361E-16));
#15855=DIRECTION('ref_axis',(0.,-3.46944695195361E-16,-1.));
#15856=DIRECTION('center_axis',(-4.93038065763132E-32,-1.,3.82856869892695E-16));
#15857=DIRECTION('ref_axis',(-9.72346137165803E-63,-3.82856869892695E-16,
-1.));
#15858=DIRECTION('',(0.,-1.,3.46944695195361E-16));
#15859=DIRECTION('center_axis',(-4.93038065763132E-32,-1.,3.82856869892695E-16));
#15860=DIRECTION('ref_axis',(-1.88763010596022E-47,-3.82856869892695E-16,
-1.));
#15861=DIRECTION('center_axis',(-1.16018306073329E-14,-3.46944695195361E-16,
-1.));
#15862=DIRECTION('ref_axis',(-1.,0.,1.16018306073329E-14));
#15863=DIRECTION('',(1.,-4.73316543132607E-30,-1.16018306073329E-14));
#15864=DIRECTION('',(0.,-1.,3.46944695195361E-16));
#15865=DIRECTION('',(1.,-4.73316543132607E-30,-1.16018306073329E-14));
#15866=DIRECTION('center_axis',(0.,-1.,3.46944695195361E-16));
#15867=DIRECTION('ref_axis',(0.,-3.46944695195361E-16,-1.));
#15868=DIRECTION('center_axis',(4.93038065763132E-32,1.,-3.82856869892695E-16));
#15869=DIRECTION('ref_axis',(-2.43086534291451E-62,-3.82856869892695E-16,
-1.));
#15870=DIRECTION('',(0.,-1.,3.46944695195361E-16));
#15871=DIRECTION('center_axis',(4.93038065763132E-32,1.,-3.82856869892695E-16));
#15872=DIRECTION('ref_axis',(-1.88763010596022E-47,-3.82856869892695E-16,
-1.));
#15873=DIRECTION('center_axis',(-1.,0.,0.));
#15874=DIRECTION('ref_axis',(0.,9.86076131526265E-32,1.));
#15875=DIRECTION('',(0.,-3.82856869891308E-16,-1.));
#15876=DIRECTION('',(0.,-1.,3.46944695195361E-16));
#15877=DIRECTION('',(0.,-3.82856869891308E-16,-1.));
#15878=DIRECTION('center_axis',(1.0991207943789E-14,3.46944695195361E-16,
1.));
#15879=DIRECTION('ref_axis',(1.,0.,-1.0991207943789E-14));
#15880=DIRECTION('',(-1.,3.94430452610506E-30,1.0991207943789E-14));
#15881=DIRECTION('',(-1.,3.94430452610506E-30,1.0991207943789E-14));
#15882=DIRECTION('center_axis',(-4.93038065763132E-32,-1.,3.82856869892695E-16));
#15883=DIRECTION('ref_axis',(0.,-3.82856869892695E-16,-1.));
#15884=DIRECTION('center_axis',(-4.93038065763132E-32,-1.,3.82856869892695E-16));
#15885=DIRECTION('ref_axis',(0.,-3.82856869892695E-16,-1.));
#15886=DIRECTION('center_axis',(-1.,-6.85322911410754E-30,-1.02140518265514E-14));
#15887=DIRECTION('ref_axis',(-1.02140518265514E-14,0.,1.));
#15888=DIRECTION('',(-1.02140518265514E-14,6.57977215693388E-16,1.));
#15889=DIRECTION('',(-1.75644810928116E-31,1.,-6.93889390390723E-16));
#15890=DIRECTION('',(-1.02140518265514E-14,6.57977215693388E-16,1.));
#15891=DIRECTION('',(-1.75644810928116E-31,1.,-6.93889390390723E-16));
#15892=DIRECTION('center_axis',(-1.11022302462516E-16,-6.93889390390723E-16,
-1.));
#15893=DIRECTION('ref_axis',(-1.75644810928116E-31,1.,-6.93889390390723E-16));
#15894=DIRECTION('',(-1.,-1.22464679914735E-16,1.11022302462516E-16));
#15895=DIRECTION('',(-1.75644810928116E-31,1.,-6.93889390390723E-16));
#15896=DIRECTION('',(-1.,-1.22464679914735E-16,1.11022302462516E-16));
#15897=DIRECTION('center_axis',(-1.75644810928116E-31,1.,-6.93889390390723E-16));
#15898=DIRECTION('ref_axis',(7.77876909732643E-62,6.93889390390723E-16,
1.));
#15899=DIRECTION('center_axis',(1.22464679914736E-16,-1.,6.57977215693389E-16));
#15900=DIRECTION('ref_axis',(-8.05789691110799E-32,6.57977215693389E-16,
1.));
#15901=DIRECTION('',(-1.75644810928116E-31,1.,-6.93889390390723E-16));
#15902=DIRECTION('center_axis',(1.22464679914736E-16,-1.,6.57977215693389E-16));
#15903=DIRECTION('ref_axis',(6.07126862973252E-47,6.57977215693389E-16,
1.));
#15904=DIRECTION('center_axis',(1.,7.09974814698911E-30,1.0547118733939E-14));
#15905=DIRECTION('ref_axis',(1.0547118733939E-14,1.4791141972894E-31,-1.));
#15906=DIRECTION('',(1.0547118733939E-14,-6.57977215693387E-16,-1.));
#15907=DIRECTION('',(-1.75644810928116E-31,1.,-6.93889390390723E-16));
#15908=DIRECTION('',(1.0547118733939E-14,-6.57977215693387E-16,-1.));
#15909=DIRECTION('center_axis',(-1.75644810928116E-31,1.,-6.93889390390723E-16));
#15910=DIRECTION('ref_axis',(0.,6.93889390390723E-16,1.));
#15911=DIRECTION('center_axis',(-1.22464679914736E-16,1.,-6.57977215693389E-16));
#15912=DIRECTION('ref_axis',(8.05789691110799E-32,-6.57977215693389E-16,
-1.));
#15913=DIRECTION('',(-1.75644810928116E-31,1.,-6.93889390390723E-16));
#15914=DIRECTION('center_axis',(-1.22464679914736E-16,1.,-6.57977215693389E-16));
#15915=DIRECTION('ref_axis',(4.9731792179006E-48,-6.57977215693389E-16,
-1.));
#15916=DIRECTION('center_axis',(1.14908083048704E-14,-6.93889390390723E-16,
-1.));
#15917=DIRECTION('ref_axis',(-1.,1.4791141972894E-31,-1.14908083048704E-14));
#15918=DIRECTION('',(-1.,-1.22464679914743E-16,-1.14908083048704E-14));
#15919=DIRECTION('',(-1.75644810928116E-31,1.,-6.93889390390723E-16));
#15920=DIRECTION('',(-1.,-1.22464679914743E-16,-1.14908083048704E-14));
#15921=DIRECTION('center_axis',(-1.75644810928116E-31,1.,-6.93889390390723E-16));
#15922=DIRECTION('ref_axis',(-7.77876909732643E-62,6.93889390390723E-16,
1.));
#15923=DIRECTION('center_axis',(1.22464679914736E-16,-1.,6.57977215693389E-16));
#15924=DIRECTION('ref_axis',(8.05789691110799E-32,-6.57977215693389E-16,
-1.));
#15925=DIRECTION('',(-1.75644810928116E-31,1.,-6.93889390390723E-16));
#15926=DIRECTION('center_axis',(1.22464679914736E-16,-1.,6.57977215693389E-16));
#15927=DIRECTION('ref_axis',(1.25397265995815E-46,-6.57977215693389E-16,
-1.));
#15928=DIRECTION('center_axis',(1.,-2.95822839457879E-31,-1.11022302462516E-16));
#15929=DIRECTION('ref_axis',(-1.11022302462516E-16,0.,-1.));
#15930=DIRECTION('',(-1.11022302462516E-16,-6.57977215694776E-16,-1.));
#15931=DIRECTION('',(-1.75644810928116E-31,1.,-6.93889390390723E-16));
#15932=DIRECTION('',(-1.11022302462516E-16,-6.57977215694776E-16,-1.));
#15933=DIRECTION('center_axis',(-1.07136521876328E-14,6.93889390390723E-16,
1.));
#15934=DIRECTION('ref_axis',(1.,-3.45126646034193E-31,1.07136521876328E-14));
#15935=DIRECTION('',(1.,1.22464679914742E-16,1.07136521876328E-14));
#15936=DIRECTION('',(1.,1.22464679914742E-16,1.07136521876328E-14));
#15937=DIRECTION('center_axis',(-1.22464679914736E-16,1.,-6.57977215693389E-16));
#15938=DIRECTION('ref_axis',(-1.11022302462516E-16,-6.57977215693389E-16,
-1.));
#15939=DIRECTION('center_axis',(-1.22464679914736E-16,1.,-6.57977215693389E-16));
#15940=DIRECTION('ref_axis',(-1.11022302462516E-16,-6.57977215693389E-16,
-1.));
#15941=DIRECTION('center_axis',(1.,-3.6253356482683E-30,1.04493185757658E-14));
#15942=DIRECTION('ref_axis',(-1.04493185757658E-14,0.,1.));
#15943=DIRECTION('',(1.04493185757658E-14,3.82856869892695E-16,-1.));
#15944=DIRECTION('',(0.,-1.,-3.46944695195361E-16));
#15945=DIRECTION('',(1.04493185757658E-14,3.82856869892695E-16,-1.));
#15946=DIRECTION('',(0.,-1.,-3.46944695195361E-16));
#15947=DIRECTION('center_axis',(0.,-3.46944695195361E-16,1.));
#15948=DIRECTION('ref_axis',(0.,1.,3.46944695195361E-16));
#15949=DIRECTION('',(1.,0.,0.));
#15950=DIRECTION('',(1.,0.,0.));
#15951=DIRECTION('',(0.,-1.,-3.46944695195361E-16));
#15952=DIRECTION('center_axis',(0.,-1.,-3.46944695195361E-16));
#15953=DIRECTION('ref_axis',(0.,-3.46944695195361E-16,1.));
#15954=DIRECTION('center_axis',(0.,-1.,-3.82856869892695E-16));
#15955=DIRECTION('ref_axis',(0.,3.82856869892695E-16,-1.));
#15956=DIRECTION('center_axis',(0.,-1.,-3.82856869892695E-16));
#15957=DIRECTION('ref_axis',(0.,3.82856869892695E-16,-1.));
#15958=DIRECTION('',(0.,-1.,-3.46944695195361E-16));
#15959=DIRECTION('center_axis',(-1.,3.70563421514164E-30,-1.06807634371093E-14));
#15960=DIRECTION('ref_axis',(1.06807634371093E-14,0.,-1.));
#15961=DIRECTION('',(-1.06807634371093E-14,-3.82856869892695E-16,1.));
#15962=DIRECTION('',(-1.06807634371093E-14,-3.82856869892695E-16,1.));
#15963=DIRECTION('',(0.,-1.,-3.46944695195361E-16));
#15964=DIRECTION('center_axis',(0.,-1.,-3.46944695195361E-16));
#15965=DIRECTION('ref_axis',(0.,-3.46944695195361E-16,1.));
#15966=DIRECTION('center_axis',(0.,1.,3.82856869892695E-16));
#15967=DIRECTION('ref_axis',(0.,-3.82856869892695E-16,1.));
#15968=DIRECTION('center_axis',(0.,1.,3.82856869892695E-16));
#15969=DIRECTION('ref_axis',(0.,-3.82856869892695E-16,1.));
#15970=DIRECTION('',(0.,-1.,-3.46944695195361E-16));
#15971=DIRECTION('center_axis',(-1.16517419313919E-14,-3.46944695195361E-16,
1.));
#15972=DIRECTION('ref_axis',(-1.,-1.09476442525376E-46,-1.16517419313919E-14));
#15973=DIRECTION('',(1.,-4.5545613262468E-30,1.16517419313919E-14));
#15974=DIRECTION('',(1.,-4.5545613262468E-30,1.16517419313919E-14));
#15975=DIRECTION('',(0.,-1.,-3.46944695195361E-16));
#15976=DIRECTION('center_axis',(0.,-1.,-3.46944695195361E-16));
#15977=DIRECTION('ref_axis',(0.,-3.46944695195361E-16,1.));
#15978=DIRECTION('center_axis',(0.,-1.,-3.82856869892695E-16));
#15979=DIRECTION('ref_axis',(0.,-3.82856869892695E-16,1.));
#15980=DIRECTION('center_axis',(0.,-1.,-3.82856869892695E-16));
#15981=DIRECTION('ref_axis',(0.,-3.82856869892695E-16,1.));
#15982=DIRECTION('',(0.,-1.,-3.46944695195361E-16));
#15983=DIRECTION('center_axis',(-1.,0.,0.));
#15984=DIRECTION('ref_axis',(0.,0.,-1.));
#15985=DIRECTION('',(0.,-3.82856869891308E-16,1.));
#15986=DIRECTION('',(0.,-3.82856869891308E-16,1.));
#15987=DIRECTION('',(0.,-1.,-3.46944695195361E-16));
#15988=DIRECTION('center_axis',(1.09273919746571E-14,3.46944695195361E-16,
-1.));
#15989=DIRECTION('ref_axis',(1.,-3.28429327576129E-46,1.09273919746571E-14));
#15990=DIRECTION('',(-1.,4.01021285003471E-30,-1.09273919746571E-14));
#15991=DIRECTION('',(-1.,4.01021285003471E-30,-1.09273919746571E-14));
#15992=DIRECTION('center_axis',(0.,-1.,-3.82856869892695E-16));
#15993=DIRECTION('ref_axis',(0.,-3.82856869892695E-16,1.));
#15994=DIRECTION('center_axis',(0.,-1.,-3.82856869892695E-16));
#15995=DIRECTION('ref_axis',(0.,-3.82856869892695E-16,1.));
#15996=DIRECTION('center_axis',(-1.,-7.10622655070755E-30,1.02411517586486E-14));
#15997=DIRECTION('ref_axis',(-1.02411517586486E-14,0.,-1.));
#15998=DIRECTION('',(-1.02411517586486E-14,6.57977215693388E-16,-1.));
#15999=DIRECTION('',(0.,1.,6.93889390390723E-16));
#16000=DIRECTION('',(-1.02411517586486E-14,6.57977215693388E-16,-1.));
#16001=DIRECTION('',(0.,1.,6.93889390390723E-16));
#16002=DIRECTION('center_axis',(-2.08166817117217E-16,-6.93889390390723E-16,
1.));
#16003=DIRECTION('ref_axis',(0.,1.,6.93889390390723E-16));
#16004=DIRECTION('',(-1.,-1.22464679914735E-16,-2.08166817117217E-16));
#16005=DIRECTION('',(-1.,-1.22464679914735E-16,-2.08166817117217E-16));
#16006=DIRECTION('',(0.,1.,6.93889390390723E-16));
#16007=DIRECTION('center_axis',(0.,1.,6.93889390390723E-16));
#16008=DIRECTION('ref_axis',(0.,6.93889390390723E-16,-1.));
#16009=DIRECTION('center_axis',(-1.22464679914735E-16,1.,6.57977215693389E-16));
#16010=DIRECTION('ref_axis',(-8.05789691110797E-32,6.57977215693389E-16,
-1.));
#16011=DIRECTION('center_axis',(-1.22464679914735E-16,1.,6.57977215693389E-16));
#16012=DIRECTION('ref_axis',(7.11800305454381E-47,6.57977215693389E-16,
-1.));
#16013=DIRECTION('',(0.,1.,6.93889390390723E-16));
#16014=DIRECTION('center_axis',(1.,7.26682368445424E-30,-1.04725966199921E-14));
#16015=DIRECTION('ref_axis',(1.04725966199921E-14,0.,1.));
#16016=DIRECTION('',(1.04725966199921E-14,-6.57977215693388E-16,1.));
#16017=DIRECTION('',(1.04725966199921E-14,-6.57977215693388E-16,1.));
#16018=DIRECTION('',(0.,1.,6.93889390390723E-16));
#16019=DIRECTION('center_axis',(0.,1.,6.93889390390723E-16));
#16020=DIRECTION('ref_axis',(0.,6.93889390390723E-16,-1.));
#16021=DIRECTION('center_axis',(1.22464679914735E-16,-1.,-6.57977215693389E-16));
#16022=DIRECTION('ref_axis',(8.05789691110797E-32,-6.57977215693389E-16,
1.));
#16023=DIRECTION('center_axis',(1.22464679914735E-16,-1.,-6.57977215693389E-16));
#16024=DIRECTION('ref_axis',(-1.64418092827499E-47,-6.57977215693389E-16,
1.));
#16025=DIRECTION('',(0.,1.,6.93889390390723E-16));
#16026=DIRECTION('center_axis',(1.14435751142747E-14,-6.93889390390723E-16,
1.));
#16027=DIRECTION('ref_axis',(-1.,-8.75811540203011E-47,1.14435751142747E-14));
#16028=DIRECTION('',(-1.,-1.22464679914743E-16,1.14435751142747E-14));
#16029=DIRECTION('',(-1.,-1.22464679914743E-16,1.14435751142747E-14));
#16030=DIRECTION('',(0.,1.,6.93889390390723E-16));
#16031=DIRECTION('center_axis',(0.,1.,6.93889390390723E-16));
#16032=DIRECTION('ref_axis',(0.,6.93889390390723E-16,-1.));
#16033=DIRECTION('center_axis',(-1.22464679914735E-16,1.,6.57977215693389E-16));
#16034=DIRECTION('ref_axis',(8.05789691110797E-32,-6.57977215693389E-16,
1.));
#16035=DIRECTION('center_axis',(-1.22464679914735E-16,1.,6.57977215693389E-16));
#16036=DIRECTION('ref_axis',(1.03982277495164E-46,-6.57977215693389E-16,
1.));
#16037=DIRECTION('',(0.,1.,6.93889390390723E-16));
#16038=DIRECTION('center_axis',(1.,-1.44444745829043E-31,2.08166817117217E-16));
#16039=DIRECTION('ref_axis',(-2.08166817117217E-16,0.,1.));
#16040=DIRECTION('',(-2.08166817117217E-16,-6.57977215694776E-16,1.));
#16041=DIRECTION('',(-2.08166817117217E-16,-6.57977215694776E-16,1.));
#16042=DIRECTION('',(0.,1.,6.93889390390723E-16));
#16043=DIRECTION('center_axis',(-1.07192251575398E-14,6.93889390390723E-16,
-1.));
#16044=DIRECTION('ref_axis',(1.,6.56858655152258E-46,-1.07192251575398E-14));
#16045=DIRECTION('',(1.,1.22464679914743E-16,-1.07192251575398E-14));
#16046=DIRECTION('',(1.,1.22464679914743E-16,-1.07192251575398E-14));
#16047=DIRECTION('center_axis',(-1.22464679914735E-16,1.,6.57977215693389E-16));
#16048=DIRECTION('ref_axis',(-2.08166817117217E-16,-6.57977215693389E-16,
1.));
#16049=DIRECTION('center_axis',(-1.22464679914735E-16,1.,6.57977215693389E-16));
#16050=DIRECTION('ref_axis',(-2.08166817117217E-16,-6.57977215693389E-16,
1.));
#16051=DIRECTION('center_axis',(3.46944695195361E-17,1.,-1.14491749414469E-16));
#16052=DIRECTION('ref_axis',(2.13821176807408E-50,1.14491749414469E-16,
1.));
#16053=DIRECTION('',(1.09356967925578E-14,-5.89805981832114E-17,-1.));
#16054=DIRECTION('',(1.,4.77048955893622E-17,-5.55111512312578E-17));
#16055=DIRECTION('center_axis',(-3.46944695195361E-17,-1.,2.16840434497101E-17));
#16056=DIRECTION('ref_axis',(3.21991412577252E-33,-2.16840434497101E-17,
-1.));
#16057=DIRECTION('',(-7.71605002114484E-15,6.33174068731535E-17,1.));
#16058=DIRECTION('center_axis',(3.46944695195361E-17,1.,-2.16840434497101E-17));
#16059=DIRECTION('ref_axis',(-3.21991412577236E-33,2.16840434497101E-17,
1.));
#16060=DIRECTION('',(1.,5.29090660172926E-17,1.16018306073329E-14));
#16061=DIRECTION('center_axis',(-3.46944695195361E-17,-1.,2.16840434497101E-17));
#16062=DIRECTION('ref_axis',(-3.2199141257724E-33,2.16840434497101E-17,
1.));
#16063=DIRECTION('',(0.,5.20417042793042E-17,1.));
#16064=DIRECTION('',(-1.,-4.77048955893622E-17,-1.03805852802452E-14));
#16065=DIRECTION('center_axis',(1.03805852802452E-14,-5.72458747072346E-17,
-1.));
#16066=DIRECTION('ref_axis',(-1.,-4.77048955893622E-17,-1.03805852802452E-14));
#16067=DIRECTION('',(4.59701721133853E-17,1.,4.16333634234433E-17));
#16068=DIRECTION('',(-1.,-1.04308922610485E-14,-1.04360964314765E-14));
#16069=DIRECTION('',(4.59701721133853E-17,1.,4.16333634234433E-17));
#16070=DIRECTION('center_axis',(-1.,-4.77048955893622E-17,2.48264406893667E-33));
#16071=DIRECTION('ref_axis',(0.,5.20417042793042E-17,1.));
#16072=DIRECTION('',(4.59701721133853E-17,1.,4.16333634234433E-17));
#16073=DIRECTION('',(-2.77555756156289E-16,0.707106781186548,0.707106781186547));
#16074=DIRECTION('center_axis',(4.59701721133853E-17,1.,4.16333634234433E-17));
#16075=DIRECTION('ref_axis',(-4.30625898502832E-33,-4.16333634234433E-17,
1.));
#16076=DIRECTION('',(4.59701721133853E-17,1.,4.16333634234433E-17));
#16077=DIRECTION('center_axis',(9.57910591987181E-15,-0.707106781186552,
0.707106781186543));
#16078=DIRECTION('ref_axis',(3.75170549529962E-13,-0.707106781186543,-0.707106781186552));
#16079=DIRECTION('center_axis',(-1.16018306073329E-14,5.63785129692462E-17,
1.));
#16080=DIRECTION('ref_axis',(1.,5.8113236445223E-17,1.16018306073329E-14));
#16081=DIRECTION('',(4.59701721133853E-17,1.,4.16333634234433E-17));
#16082=DIRECTION('',(1.,1.17015772072015E-14,1.16018306073329E-14));
#16083=DIRECTION('center_axis',(4.59701721133853E-17,1.,4.16333634234433E-17));
#16084=DIRECTION('ref_axis',(-4.30625898502839E-33,-4.16333634234433E-17,
1.));
#16085=DIRECTION('',(4.59701721133853E-17,1.,4.16333634234433E-17));
#16086=DIRECTION('center_axis',(2.87774982255266E-14,0.70710678118654,-0.707106781186555));
#16087=DIRECTION('ref_axis',(-1.67738755276477E-12,0.707106781186555,0.70710678118654));
#16088=DIRECTION('center_axis',(-1.,-4.9439619065339E-17,-7.71605002114484E-15));
#16089=DIRECTION('ref_axis',(-7.71605002114484E-15,6.33174068731535E-17,
1.));
#16090=DIRECTION('',(4.59701721133853E-17,1.,4.16333634234433E-17));
#16091=DIRECTION('',(-5.71764857681955E-15,0.707106781186548,0.707106781186547));
#16092=DIRECTION('center_axis',(4.59701721133853E-17,1.,4.16333634234433E-17));
#16093=DIRECTION('ref_axis',(-4.3062589850284E-33,-4.16333634234433E-17,
1.));
#16094=DIRECTION('',(4.59701721133853E-17,1.,4.16333634234433E-17));
#16095=DIRECTION('center_axis',(-6.92543468531269E-14,-0.707106781186525,
0.70710678118657));
#16096=DIRECTION('ref_axis',(-5.72091053931135E-13,-0.70710678118657,-0.707106781186525));
#16097=DIRECTION('center_axis',(5.55111512312578E-17,5.20417042793042E-17,
1.));
#16098=DIRECTION('ref_axis',(1.,4.77048955893622E-17,-5.55111512312578E-17));
#16099=DIRECTION('',(4.59701721133853E-17,1.,4.16333634234433E-17));
#16100=DIRECTION('',(1.,4.77048955893622E-17,-5.55111512312578E-17));
#16101=DIRECTION('center_axis',(1.,5.03069808033274E-17,1.09356967925578E-14));
#16102=DIRECTION('ref_axis',(1.09356967925578E-14,-5.89805981832114E-17,
-1.));
#16103=DIRECTION('',(7.82707232360735E-15,-0.707106781186548,-0.707106781186547));
#16104=DIRECTION('center_axis',(-1.66533453693774E-16,-0.707106781186547,
0.707106781186548));
#16105=DIRECTION('ref_axis',(2.77555756156289E-16,-0.707106781186548,-0.707106781186547));
#16106=DIRECTION('center_axis',(1.,1.0769163338864E-14,-1.46936793852784E-39));
#16107=DIRECTION('ref_axis',(-1.0769163338864E-14,1.,6.61744490042422E-24));
#16108=DIRECTION('',(-7.43849426498854E-15,0.707106781186548,-0.707106781186547));
#16109=DIRECTION('',(0.,-1.32348898008484E-23,-1.));
#16110=DIRECTION('',(7.4940054162198E-15,-0.707106781186548,-0.707106781186547));
#16111=DIRECTION('',(0.,-1.32348898008484E-23,-1.));
#16112=DIRECTION('center_axis',(0.,1.,-1.32348898008484E-23));
#16113=DIRECTION('ref_axis',(0.,1.32348898008484E-23,1.));
#16114=DIRECTION('',(-1.,-1.66533453693773E-16,1.32348898008484E-23));
#16115=DIRECTION('',(0.,-1.32348898008484E-23,-1.));
#16116=DIRECTION('',(1.,1.66533453693773E-16,-1.32348898008484E-23));
#16117=DIRECTION('center_axis',(0.,-1.32348898008484E-23,-1.));
#16118=DIRECTION('ref_axis',(-1.,0.,0.));
#16119=DIRECTION('center_axis',(7.7668426377335E-15,-0.707106781186543,
-0.707106781186552));
#16120=DIRECTION('ref_axis',(-1.50420492628612E-12,0.707106781186552,-0.707106781186543));
#16121=DIRECTION('',(0.,-1.32348898008484E-23,-1.));
#16122=DIRECTION('center_axis',(-8.47880321285962E-15,-0.707106781186537,
0.707106781186558));
#16123=DIRECTION('ref_axis',(-1.33652306564903E-12,-0.707106781186558,-0.707106781186537));
#16124=DIRECTION('center_axis',(-1.,-7.66053886991358E-15,6.61744490042422E-24));
#16125=DIRECTION('ref_axis',(7.66053886991358E-15,-1.,-3.97046694025453E-23));
#16126=DIRECTION('',(5.21804821573823E-15,-0.707106781186548,0.707106781186547));
#16127=DIRECTION('',(0.,-1.32348898008484E-23,-1.));
#16128=DIRECTION('',(-5.27355936696949E-15,0.707106781186548,0.707106781186547));
#16129=DIRECTION('center_axis',(0.,-1.32348898008484E-23,-1.));
#16130=DIRECTION('ref_axis',(-1.,0.,0.));
#16131=DIRECTION('center_axis',(2.62788531700192E-14,0.707106781186538,
0.707106781186557));
#16132=DIRECTION('ref_axis',(-1.00193785715871E-13,-0.707106781186557,0.707106781186538));
#16133=DIRECTION('',(0.,-1.32348898008484E-23,-1.));
#16134=DIRECTION('center_axis',(1.15454633599422E-14,0.707106781186547,
-0.707106781186548));
#16135=DIRECTION('ref_axis',(-1.20981655275665E-12,0.707106781186548,0.707106781186547));
#16136=DIRECTION('center_axis',(-1.17128529097954E-14,1.,2.64697796016969E-23));
#16137=DIRECTION('ref_axis',(-1.,-1.17128529097954E-14,0.));
#16138=DIRECTION('',(-1.,-1.17128529097954E-14,1.16517419311056E-14));
#16139=DIRECTION('',(0.,-1.32348898008484E-23,-1.));
#16140=DIRECTION('',(1.,1.17128529097954E-14,1.16517419311056E-14));
#16141=DIRECTION('center_axis',(0.,-1.32348898008484E-23,-1.));
#16142=DIRECTION('ref_axis',(-1.,0.,0.));
#16143=DIRECTION('center_axis',(1.37214219933299E-14,-0.70710678118655,
-0.707106781186545));
#16144=DIRECTION('ref_axis',(-1.13009119520484E-12,0.707106781186545,-0.70710678118655));
#16145=DIRECTION('',(0.,-1.32348898008484E-23,-1.));
#16146=DIRECTION('center_axis',(2.9902344155278E-14,-0.707106781186557,
0.707106781186538));
#16147=DIRECTION('ref_axis',(-1.59121631194934E-12,-0.707106781186538,-0.707106781186557));
#16148=DIRECTION('center_axis',(-1.,-1.66533453693773E-16,2.20405190779179E-39));
#16149=DIRECTION('ref_axis',(0.,1.32348898008484E-23,1.));
#16150=DIRECTION('',(-2.22044604925031E-16,-0.707106781186548,0.707106781186547));
#16151=DIRECTION('',(0.,-1.32348898008484E-23,-1.));
#16152=DIRECTION('',(1.66533453693773E-16,0.707106781186548,0.707106781186547));
#16153=DIRECTION('center_axis',(1.04360964314765E-14,-1.,0.));
#16154=DIRECTION('ref_axis',(1.,1.04360964314765E-14,0.));
#16155=DIRECTION('',(1.,1.04360964314765E-14,-1.03810223757158E-14));
#16156=DIRECTION('',(-1.,-1.04360964314765E-14,-1.03810223757158E-14));
#16157=DIRECTION('center_axis',(-1.11022302462516E-16,-0.707106781186547,
0.707106781186548));
#16158=DIRECTION('ref_axis',(-1.66533453693773E-16,-0.707106781186548,-0.707106781186547));
#16159=DIRECTION('center_axis',(-1.66533453693773E-16,-0.707106781186547,
-0.707106781186548));
#16160=DIRECTION('ref_axis',(2.22044604925031E-16,0.707106781186548,-0.707106781186547));
#16161=DIRECTION('center_axis',(-7.8062556418956E-18,-1.,-9.19403442267707E-17));
#16162=DIRECTION('ref_axis',(4.44089209850062E-16,9.19403442267707E-17,
-1.));
#16163=DIRECTION('',(1.06026298851702E-14,-1.45716771982052E-16,1.));
#16164=DIRECTION('',(-1.,-1.21430643318376E-17,1.08246744900953E-14));
#16165=DIRECTION('',(4.44089209850062E-16,1.50920942409982E-16,-1.));
#16166=DIRECTION('center_axis',(7.80625564189562E-18,1.,4.07660016854549E-17));
#16167=DIRECTION('ref_axis',(-3.99480000183453E-34,4.07660016854549E-17,
-1.));
#16168=DIRECTION('',(1.,1.47451495458029E-17,-1.19904086659517E-14));
#16169=DIRECTION('center_axis',(-7.80625564189562E-18,-1.,-4.07660016854549E-17));
#16170=DIRECTION('ref_axis',(-3.99480000183441E-34,4.07660016854549E-17,
-1.));
#16171=DIRECTION('',(-7.32747196252603E-15,1.50920942409982E-16,-1.));
#16172=DIRECTION('center_axis',(7.80625564189562E-18,1.,4.07660016854549E-17));
#16173=DIRECTION('ref_axis',(3.99480000183447E-34,-4.07660016854549E-17,
1.));
#16174=DIRECTION('',(1.,1.73472347597681E-17,-3.33066907387547E-16));
#16175=DIRECTION('center_axis',(1.08246744900953E-14,-3.20923843055709E-17,
1.));
#16176=DIRECTION('ref_axis',(1.,1.21430643318377E-17,-1.08246744900953E-14));
#16177=DIRECTION('',(-1.21430643318376E-17,-1.,2.60208521396521E-17));
#16178=DIRECTION('',(1.,1.03866568124111E-14,-1.0769163338864E-14));
#16179=DIRECTION('',(-1.21430643318376E-17,-1.,2.60208521396521E-17));
#16180=DIRECTION('center_axis',(-1.,-1.7347234759768E-17,-4.44089209850062E-16));
#16181=DIRECTION('ref_axis',(-4.44089209850062E-16,-2.94902990916057E-17,
1.));
#16182=DIRECTION('',(-2.77555756156289E-16,-0.707106781186548,0.707106781186547));
#16183=DIRECTION('',(-1.21430643318376E-17,-1.,2.60208521396521E-17));
#16184=DIRECTION('center_axis',(-1.21430643318376E-17,-1.,2.60208521396521E-17));
#16185=DIRECTION('ref_axis',(-3.1597288150103E-34,-2.60208521396521E-17,
-1.));
#16186=DIRECTION('center_axis',(-1.13913692020097E-14,-0.707106781186534,
-0.707106781186561));
#16187=DIRECTION('ref_axis',(1.83534137375699E-13,0.707106781186561,-0.707106781186534));
#16188=DIRECTION('',(-1.21430643318376E-17,-1.,2.60208521396521E-17));
#16189=DIRECTION('center_axis',(-1.19904086659517E-14,2.08166817117216E-17,
-1.));
#16190=DIRECTION('ref_axis',(-1.,-1.82145964977565E-17,1.19904086659517E-14));
#16191=DIRECTION('',(-1.,-1.1669484822896E-14,1.21569421196455E-14));
#16192=DIRECTION('',(-1.21430643318376E-17,-1.,2.60208521396521E-17));
#16193=DIRECTION('center_axis',(-1.21430643318376E-17,-1.,2.60208521396521E-17));
#16194=DIRECTION('ref_axis',(-3.1597288150103E-34,-2.60208521396521E-17,
-1.));
#16195=DIRECTION('center_axis',(1.37856278924687E-14,0.707106781186535,
0.70710678118656));
#16196=DIRECTION('ref_axis',(-8.00926025379328E-13,-0.70710678118656,0.707106781186535));
#16197=DIRECTION('',(-1.21430643318376E-17,-1.,2.60208521396521E-17));
#16198=DIRECTION('center_axis',(-1.,-1.3010426069826E-17,7.32747196252603E-15));
#16199=DIRECTION('ref_axis',(7.32747196252603E-15,-2.60208521396521E-17,
1.));
#16200=DIRECTION('',(5.10702591327571E-15,-0.707106781186548,0.707106781186547));
#16201=DIRECTION('',(-1.21430643318376E-17,-1.,2.60208521396521E-17));
#16202=DIRECTION('center_axis',(-1.21430643318376E-17,-1.,2.60208521396521E-17));
#16203=DIRECTION('ref_axis',(-3.1597288150103E-34,-2.60208521396521E-17,
-1.));
#16204=DIRECTION('center_axis',(-3.88342131886675E-15,-0.70710678118655,
-0.707106781186545));
#16205=DIRECTION('ref_axis',(-1.83322773685989E-12,0.707106781186545,-0.70710678118655));
#16206=DIRECTION('',(-1.21430643318376E-17,-1.,2.60208521396521E-17));
#16207=DIRECTION('center_axis',(-3.33066907387547E-16,2.94902990916057E-17,
-1.));
#16208=DIRECTION('ref_axis',(-1.,-1.73472347597681E-17,3.33066907387547E-16));
#16209=DIRECTION('',(-1.,-1.73472347597681E-17,3.33066907387547E-16));
#16210=DIRECTION('',(-1.21430643318376E-17,-1.,2.60208521396521E-17));
#16211=DIRECTION('center_axis',(1.,2.42861286636753E-17,-1.06026298851702E-14));
#16212=DIRECTION('ref_axis',(-1.06026298851702E-14,2.42861286636753E-17,
-1.));
#16213=DIRECTION('',(-7.27196081129477E-15,0.707106781186548,-0.707106781186547));
#16214=DIRECTION('center_axis',(3.33066907387547E-16,-0.707106781186547,
-0.707106781186548));
#16215=DIRECTION('ref_axis',(2.77555756156289E-16,0.707106781186548,-0.707106781186547));
#16216=DIRECTION('center_axis',(1.30104260698256E-17,-1.,-2.51534904016636E-17));
#16217=DIRECTION('ref_axis',(-6.93889390390723E-15,-2.51534904016637E-17,
1.));
#16218=DIRECTION('',(-3.88578058618805E-15,-2.60208521396521E-17,-1.));
#16219=DIRECTION('',(1.,-1.3010426069826E-17,-3.38618022510673E-15));
#16220=DIRECTION('',(-6.93889390390723E-15,3.72965547335013E-17,1.));
#16221=DIRECTION('center_axis',(-1.3010426069826E-17,1.,8.8470897274817E-17));
#16222=DIRECTION('ref_axis',(8.23786441056261E-34,-8.8470897274817E-17,
1.));
#16223=DIRECTION('',(-1.,1.64798730217797E-17,4.77395900588817E-15));
#16224=DIRECTION('center_axis',(1.3010426069826E-17,-1.,-8.8470897274817E-17));
#16225=DIRECTION('ref_axis',(8.23786441056244E-34,-8.8470897274817E-17,
1.));
#16226=DIRECTION('',(7.21644966006352E-16,3.55618312575245E-17,1.));
#16227=DIRECTION('center_axis',(-1.3010426069826E-17,1.,8.8470897274817E-17));
#16228=DIRECTION('ref_axis',(-8.23786441056256E-34,8.8470897274817E-17,
-1.));
#16229=DIRECTION('',(-1.,1.73472347597681E-17,-7.04991620636974E-15));
#16230=DIRECTION('center_axis',(-3.38618022510673E-15,-3.64291929955129E-17,
-1.));
#16231=DIRECTION('ref_axis',(-1.,1.3010426069826E-17,3.38618022510673E-15));
#16232=DIRECTION('',(1.21430643318376E-17,-1.,-2.77555756156289E-17));
#16233=DIRECTION('',(-1.,4.73926453636863E-15,3.38618022510672E-15));
#16234=DIRECTION('',(1.21430643318376E-17,-1.,-2.77555756156289E-17));
#16235=DIRECTION('center_axis',(1.,-1.73472347597681E-17,6.93889390390723E-15));
#16236=DIRECTION('ref_axis',(6.93889390390723E-15,-3.72965547335013E-17,
-1.));
#16237=DIRECTION('',(4.88498130835068E-15,-0.707106781186548,-0.707106781186548));
#16238=DIRECTION('',(1.21430643318376E-17,-1.,-2.77555756156289E-17));
#16239=DIRECTION('center_axis',(1.21430643318376E-17,-1.,-2.77555756156289E-17));
#16240=DIRECTION('ref_axis',(-3.37037740267765E-34,2.77555756156289E-17,
-1.));
#16241=DIRECTION('center_axis',(-3.52096866244013E-14,-0.707106781186563,
0.707106781186532));
#16242=DIRECTION('ref_axis',(4.00992146975888E-12,-0.707106781186532,-0.707106781186563));
#16243=DIRECTION('',(1.21430643318376E-17,-1.,-2.77555756156289E-17));
#16244=DIRECTION('center_axis',(4.49640324973188E-15,3.46944695195361E-17,
1.));
#16245=DIRECTION('ref_axis',(1.,-1.21430643318376E-17,-4.49640324973188E-15));
#16246=DIRECTION('',(1.,-6.00648003556969E-15,-4.94049245958194E-15));
#16247=DIRECTION('',(1.21430643318376E-17,-1.,-2.77555756156289E-17));
#16248=DIRECTION('center_axis',(1.21430643318376E-17,-1.,-2.77555756156289E-17));
#16249=DIRECTION('ref_axis',(-3.37037740267765E-34,2.77555756156289E-17,
-1.));
#16250=DIRECTION('center_axis',(7.75441568951419E-16,0.707106781186544,
-0.707106781186551));
#16251=DIRECTION('ref_axis',(-7.1228105608578E-13,0.707106781186551,0.707106781186544));
#16252=DIRECTION('',(1.21430643318376E-17,-1.,-2.77555756156289E-17));
#16253=DIRECTION('center_axis',(1.,-1.56125112837912E-17,-7.21644966006352E-16));
#16254=DIRECTION('ref_axis',(-7.21644966006352E-16,-3.55618312575245E-17,
-1.));
#16255=DIRECTION('',(-5.55111512312578E-16,-0.707106781186548,-0.707106781186547));
#16256=DIRECTION('',(1.21430643318376E-17,-1.,-2.77555756156289E-17));
#16257=DIRECTION('center_axis',(1.21430643318376E-17,-1.,-2.77555756156289E-17));
#16258=DIRECTION('ref_axis',(-3.37037740267765E-34,2.77555756156289E-17,
-1.));
#16259=DIRECTION('center_axis',(1.2168053465783E-14,-0.707106781186539,
0.707106781186556));
#16260=DIRECTION('ref_axis',(4.94238761493454E-13,-0.707106781186556,-0.707106781186539));
#16261=DIRECTION('',(1.21430643318376E-17,-1.,-2.77555756156289E-17));
#16262=DIRECTION('center_axis',(-7.04991620636974E-15,3.72965547335013E-17,
1.));
#16263=DIRECTION('ref_axis',(1.,-1.73472347597681E-17,7.04991620636974E-15));
#16264=DIRECTION('',(1.,5.62137142390284E-15,7.4940054162198E-15));
#16265=DIRECTION('',(1.21430643318376E-17,-1.,-2.77555756156289E-17));
#16266=DIRECTION('center_axis',(-1.,1.99493199737333E-17,3.88578058618805E-15));
#16267=DIRECTION('ref_axis',(3.88578058618805E-15,2.60208521396521E-17,
1.));
#16268=DIRECTION('',(2.77555756156289E-15,0.707106781186548,0.707106781186548));
#16269=DIRECTION('center_axis',(-8.32667268468867E-16,-0.707106781186548,
0.707106781186548));
#16270=DIRECTION('ref_axis',(-2.22044604925031E-16,-0.707106781186548,-0.707106781186548));
#16271=DIRECTION('center_axis',(-1.,5.44009282066327E-15,-1.33226766263741E-15));
#16272=DIRECTION('ref_axis',(-5.44009282066327E-15,-1.,4.63221143029696E-23));
#16273=DIRECTION('',(-4.71844785465691E-15,-0.707106781186548,0.707106781186548));
#16274=DIRECTION('',(-1.33226760969785E-15,-1.11022342167185E-16,1.));
#16275=DIRECTION('',(2.94209101525666E-15,0.707106781186547,0.707106781186548));
#16276=DIRECTION('',(-1.33226760969785E-15,-1.11022342167185E-16,1.));
#16277=DIRECTION('center_axis',(-5.6621374255883E-15,1.,1.11022223053177E-16));
#16278=DIRECTION('ref_axis',(-1.,-5.6621374255883E-15,-1.32348898008484E-23));
#16279=DIRECTION('',(-1.,-5.6621374255883E-15,5.15950545417941E-15));
#16280=DIRECTION('',(1.,5.6621374255883E-15,6.98296269881226E-15));
#16281=DIRECTION('',(-1.33226760969785E-15,-1.11022342167185E-16,1.));
#16282=DIRECTION('center_axis',(-1.33226760969785E-15,-1.11022342167185E-16,
1.));
#16283=DIRECTION('ref_axis',(1.,-1.47911470422133E-31,1.33226760969785E-15));
#16284=DIRECTION('center_axis',(2.59541991477666E-14,-0.707106781186537,
-0.707106781186559));
#16285=DIRECTION('ref_axis',(-1.63630723245591E-12,0.707106781186559,-0.707106781186536));
#16286=DIRECTION('center_axis',(1.21680534657822E-14,-0.70710678118654,
0.707106781186555));
#16287=DIRECTION('ref_axis',(-2.30210285556933E-12,-0.707106781186556,-0.707106781186539));
#16288=DIRECTION('',(-1.33226760969785E-15,-1.11022342167185E-16,1.));
#16289=DIRECTION('center_axis',(1.,-2.22044604925031E-15,1.33226765601997E-15));
#16290=DIRECTION('ref_axis',(2.22044604925031E-15,1.,-1.98523347012727E-23));
#16291=DIRECTION('',(2.4980018054066E-15,0.707106781186548,-0.707106781186547));
#16292=DIRECTION('',(-6.66133814775094E-16,-0.707106781186547,-0.707106781186548));
#16293=DIRECTION('',(-1.33226760969785E-15,-1.11022342167185E-16,1.));
#16294=DIRECTION('center_axis',(-1.33226760969785E-15,-1.11022342167185E-16,
1.));
#16295=DIRECTION('ref_axis',(1.,-1.47911470422133E-31,1.33226760969785E-15));
#16296=DIRECTION('center_axis',(-1.72320348655873E-14,0.70710678118654,
0.707106781186555));
#16297=DIRECTION('ref_axis',(1.75729287719648E-12,-0.707106781186555,0.70710678118654));
#16298=DIRECTION('center_axis',(-9.0468183044332E-15,0.707106781186546,
-0.707106781186549));
#16299=DIRECTION('ref_axis',(-6.90431943935876E-13,0.707106781186549,0.707106781186546));
#16300=DIRECTION('',(-1.33226760969785E-15,-1.11022342167185E-16,1.));
#16301=DIRECTION('center_axis',(5.93969318174459E-15,1.,1.11022242905512E-16));
#16302=DIRECTION('ref_axis',(-1.,5.93969318174459E-15,-1.32348898008484E-23));
#16303=DIRECTION('',(-1.,5.93969318174459E-15,-6.4922364769262E-15));
#16304=DIRECTION('',(1.,-5.93969318174459E-15,-4.66877923229335E-15));
#16305=DIRECTION('',(-1.33226760969785E-15,-1.11022342167185E-16,1.));
#16306=DIRECTION('center_axis',(-1.33226760969785E-15,-1.11022342167185E-16,
1.));
#16307=DIRECTION('ref_axis',(1.,-1.47911470422133E-31,1.33226760969785E-15));
#16308=DIRECTION('center_axis',(-1.35919746160361E-14,-0.70710678118655,
-0.707106781186545));
#16309=DIRECTION('ref_axis',(-1.90544366423202E-12,0.707106781186545,-0.70710678118655));
#16310=DIRECTION('center_axis',(-1.91582118397469E-14,-0.707106781186557,
0.707106781186538));
#16311=DIRECTION('ref_axis',(6.31977432729113E-13,-0.707106781186538,-0.707106781186557));
#16312=DIRECTION('',(-1.33226760969785E-15,-1.11022342167185E-16,1.));
#16313=DIRECTION('center_axis',(1.,5.60662627435704E-15,1.33226764278508E-15));
#16314=DIRECTION('ref_axis',(-5.60662627435704E-15,1.,-5.29395592033938E-23));
#16315=DIRECTION('',(-3.10862446895044E-15,0.707106781186548,-0.707106781186548));
#16316=DIRECTION('',(4.88498130835069E-15,-0.707106781186547,-0.707106781186548));
#16317=DIRECTION('',(-1.33226760969785E-15,-1.11022342167185E-16,1.));
#16318=DIRECTION('center_axis',(-4.6074255521944E-15,-1.,-1.11022249522956E-16));
#16319=DIRECTION('ref_axis',(1.,-4.6074255521944E-15,2.64697796016969E-23));
#16320=DIRECTION('',(1.,-4.6074255521944E-15,5.22151693477125E-15));
#16321=DIRECTION('',(-1.,4.6074255521944E-15,3.39805966366862E-15));
#16322=DIRECTION('center_axis',(-9.9920072216264E-16,-0.707106781186548,
0.707106781186547));
#16323=DIRECTION('ref_axis',(-1.66533453693773E-16,-0.707106781186547,-0.707106781186548));
#16324=DIRECTION('center_axis',(3.88578058618804E-16,-0.707106781186547,
-0.707106781186548));
#16325=DIRECTION('ref_axis',(1.11022302462516E-16,0.707106781186548,-0.707106781186547));
#16326=DIRECTION('center_axis',(8.35269353682832E-16,1.,1.84748050191525E-16));
#16327=DIRECTION('ref_axis',(-5.27355936696949E-15,1.8474805019153E-16,
-1.));
#16328=DIRECTION('',(-5.6621374255883E-15,-1.25767452008318E-16,1.));
#16329=DIRECTION('',(-1.,8.52616588442601E-16,5.10702591327572E-15));
#16330=DIRECTION('center_axis',(-8.35269353682832E-16,-1.,-1.82145964977565E-16));
#16331=DIRECTION('ref_axis',(2.17344203489769E-33,-1.82145964977565E-16,
1.));
#16332=DIRECTION('',(2.55351295663786E-15,1.22298005056365E-16,-1.));
#16333=DIRECTION('center_axis',(8.35269353682832E-16,1.,1.82145964977565E-16));
#16334=DIRECTION('ref_axis',(-2.17344203489616E-33,1.82145964977565E-16,
-1.));
#16335=DIRECTION('',(-1.,8.44810332800705E-16,-6.60582699651968E-15));
#16336=DIRECTION('center_axis',(-8.35269353682832E-16,-1.,-1.82145964977565E-16));
#16337=DIRECTION('ref_axis',(-2.17344203489581E-33,1.82145964977565E-16,
-1.));
#16338=DIRECTION('',(-5.27355936696949E-15,1.25767452008318E-16,-1.));
#16339=DIRECTION('',(1.,-8.4741241801467E-16,5.21804821573823E-15));
#16340=DIRECTION('center_axis',(-5.16253706450698E-15,-1.05818132034585E-16,
1.));
#16341=DIRECTION('ref_axis',(1.,-8.67361737988404E-18,5.16253706450698E-15));
#16342=DIRECTION('',(8.32667268468867E-16,1.,1.02348685082632E-16));
#16343=DIRECTION('',(1.,-4.73406036594071E-15,5.21804821573824E-15));
#16344=DIRECTION('',(8.32667268468867E-16,1.,1.02348685082632E-16));
#16345=DIRECTION('center_axis',(1.,-8.52616588442601E-16,-5.27355936696949E-15));
#16346=DIRECTION('ref_axis',(-5.27355936696949E-15,4.33680868994202E-18,
-1.));
#16347=DIRECTION('',(8.32667268468867E-16,1.,1.02348685082632E-16));
#16348=DIRECTION('',(-3.10862446895044E-15,0.707106781186548,-0.707106781186547));
#16349=DIRECTION('center_axis',(8.32667268468867E-16,1.,1.02348685082632E-16));
#16350=DIRECTION('ref_axis',(-1.,8.32667268468867E-16,-1.86424000085681E-33));
#16351=DIRECTION('',(8.32667268468867E-16,1.,1.02348685082632E-16));
#16352=DIRECTION('center_axis',(8.47880321285959E-15,-0.707106781186537,
-0.707106781186558));
#16353=DIRECTION('ref_axis',(2.64873930696695E-12,0.707106781186558,-0.707106781186537));
#16354=DIRECTION('center_axis',(6.60582699651968E-15,1.00613961606655E-16,
-1.));
#16355=DIRECTION('ref_axis',(-1.,1.12757025938492E-17,-6.60582699651968E-15));
#16356=DIRECTION('',(8.32667268468867E-16,1.,1.02348685082632E-16));
#16357=DIRECTION('',(-1.,6.00387795035573E-15,-6.60582699651968E-15));
#16358=DIRECTION('center_axis',(8.32667268468867E-16,1.,1.02348685082632E-16));
#16359=DIRECTION('ref_axis',(-1.,8.32667268468867E-16,-1.86424000085607E-33));
#16360=DIRECTION('',(8.32667268468867E-16,1.,1.02348685082632E-16));
#16361=DIRECTION('center_axis',(-8.27137673548193E-15,0.707106781186542,
0.707106781186553));
#16362=DIRECTION('ref_axis',(-2.01011831778871E-13,-0.707106781186553,0.707106781186542));
#16363=DIRECTION('center_axis',(1.,-8.49147141490647E-16,2.55351295663786E-15));
#16364=DIRECTION('ref_axis',(2.55351295663786E-15,-2.60208521396521E-18,
-1.));
#16365=DIRECTION('',(8.32667268468867E-16,1.,1.02348685082632E-16));
#16366=DIRECTION('',(2.55351295663786E-15,0.707106781186548,-0.707106781186547));
#16367=DIRECTION('center_axis',(8.32667268468867E-16,1.,1.02348685082632E-16));
#16368=DIRECTION('ref_axis',(-1.,8.32667268468867E-16,-1.86424000085454E-33));
#16369=DIRECTION('',(8.32667268468867E-16,1.,1.02348685082632E-16));
#16370=DIRECTION('center_axis',(5.56623722370933E-15,-0.707106781186541,
-0.707106781186554));
#16371=DIRECTION('ref_axis',(-4.75568302221126E-13,0.707106781186554,-0.707106781186541));
#16372=DIRECTION('center_axis',(-5.10702591327572E-15,1.0842021724855E-16,
-1.));
#16373=DIRECTION('ref_axis',(-1.,1.12757025938492E-17,5.10702591327572E-15));
#16374=DIRECTION('',(8.32667268468867E-16,1.,1.02348685082632E-16));
#16375=DIRECTION('',(-1.,-5.6395860204006E-15,5.27355936696949E-15));
#16376=DIRECTION('center_axis',(-1.,8.45677694538693E-16,-5.6621374255883E-15));
#16377=DIRECTION('ref_axis',(-5.6621374255883E-15,-4.33680868994202E-18,
1.));
#16378=DIRECTION('',(-4.71844785465692E-15,-0.707106781186548,0.707106781186547));
#16379=DIRECTION('center_axis',(3.88578058618805E-16,-0.707106781186547,
-0.707106781186548));
#16380=DIRECTION('ref_axis',(1.11022302462516E-16,0.707106781186548,-0.707106781186547));
#16381=DIRECTION('center_axis',(-1.0345260002189E-14,1.,0.));
#16382=DIRECTION('ref_axis',(-1.,-1.0345260002189E-14,0.));
#16383=DIRECTION('center_axis',(-1.0345260002189E-14,1.,0.));
#16384=DIRECTION('ref_axis',(-1.,-1.0345260002189E-14,0.));
#16385=DIRECTION('',(-1.0345260002189E-14,1.,0.));
#16386=DIRECTION('center_axis',(-1.0345260002189E-14,1.,0.));
#16387=DIRECTION('ref_axis',(-1.,-1.0345260002189E-14,0.));
#16388=DIRECTION('',(-1.0345260002189E-14,1.,0.));
#16389=DIRECTION('center_axis',(-1.0345260002189E-14,1.,0.));
#16390=DIRECTION('ref_axis',(-1.,-1.0345260002189E-14,0.));
#16391=DIRECTION('center_axis',(-1.0345260002189E-14,1.,0.));
#16392=DIRECTION('ref_axis',(-1.,-1.0345260002189E-14,0.));
#16393=DIRECTION('',(-1.0345260002189E-14,1.,0.));
#16394=DIRECTION('center_axis',(-1.0345260002189E-14,1.,0.));
#16395=DIRECTION('ref_axis',(-1.,-1.0345260002189E-14,0.));
#16396=DIRECTION('',(-1.0345260002189E-14,1.,0.));
#16397=DIRECTION('center_axis',(-1.0345260002189E-14,1.,0.));
#16398=DIRECTION('ref_axis',(-1.,-1.0345260002189E-14,0.));
#16399=DIRECTION('center_axis',(-1.0345260002189E-14,1.,0.));
#16400=DIRECTION('ref_axis',(-1.,-1.0345260002189E-14,0.));
#16401=DIRECTION('',(-1.0345260002189E-14,1.,0.));
#16402=DIRECTION('center_axis',(-1.0345260002189E-14,1.,0.));
#16403=DIRECTION('ref_axis',(-1.,-1.0345260002189E-14,0.));
#16404=DIRECTION('',(-1.0345260002189E-14,1.,0.));
#16405=DIRECTION('center_axis',(-1.0345260002189E-14,1.,0.));
#16406=DIRECTION('ref_axis',(-1.,-1.0345260002189E-14,0.));
#16407=DIRECTION('center_axis',(-1.0345260002189E-14,1.,0.));
#16408=DIRECTION('ref_axis',(-1.,-1.0345260002189E-14,0.));
#16409=DIRECTION('',(-1.0345260002189E-14,1.,0.));
#16410=DIRECTION('center_axis',(-1.0345260002189E-14,1.,0.));
#16411=DIRECTION('ref_axis',(-1.,-1.0345260002189E-14,0.));
#16412=DIRECTION('',(-1.0345260002189E-14,1.,0.));
#16413=DIRECTION('center_axis',(1.,1.03805852802452E-14,0.));
#16414=DIRECTION('ref_axis',(-1.03805852802452E-14,1.,0.));
#16415=DIRECTION('',(0.,0.,1.));
#16416=DIRECTION('',(-1.03805852802452E-14,1.,1.32348898008484E-23));
#16417=DIRECTION('',(0.,0.,1.));
#16418=DIRECTION('',(1.03805852802452E-14,-1.,-1.32348898008484E-23));
#16419=DIRECTION('center_axis',(-1.36918376090096E-37,1.32348898008484E-23,
-1.));
#16420=DIRECTION('ref_axis',(0.,1.,1.32348898008484E-23));
#16421=DIRECTION('',(1.,1.0345260002189E-14,0.));
#16422=DIRECTION('',(1.03805852802452E-14,-1.,-1.32348898008484E-23));
#16423=DIRECTION('',(1.,1.0345260002189E-14,0.));
#16424=DIRECTION('',(-1.03805852802452E-14,1.,1.32348898008484E-23));
#16425=DIRECTION('center_axis',(-1.,-1.03805852802452E-14,0.));
#16426=DIRECTION('ref_axis',(1.03805852802452E-14,-1.,0.));
#16427=DIRECTION('',(0.,0.,-1.));
#16428=DIRECTION('',(-1.03805852802452E-14,1.,1.32348898008484E-23));
#16429=DIRECTION('',(0.,0.,-1.));
#16430=DIRECTION('',(1.03805852802452E-14,-1.,-1.32348898008484E-23));
#16431=DIRECTION('center_axis',(1.36918376090096E-37,-1.32348898008484E-23,
1.));
#16432=DIRECTION('ref_axis',(0.,-1.,-1.32348898008484E-23));
#16433=DIRECTION('',(-1.,-1.0345260002189E-14,0.));
#16434=DIRECTION('',(-1.03805852802452E-14,1.,1.32348898008484E-23));
#16435=DIRECTION('',(-1.,-1.0345260002189E-14,0.));
#16436=DIRECTION('',(1.03805852802452E-14,-1.,-1.32348898008484E-23));
#16437=DIRECTION('center_axis',(1.0345260002189E-14,-1.,0.));
#16438=DIRECTION('ref_axis',(1.,1.0345260002189E-14,0.));
#16439=DIRECTION('',(0.707106781186544,7.31520350068574E-15,0.70710678118655));
#16440=DIRECTION('',(0.707106781186551,7.31520350068581E-15,-0.707106781186544));
#16441=DIRECTION('',(-0.707106781186549,-7.31520350068578E-15,-0.707106781186547));
#16442=DIRECTION('',(-0.707106781186549,-7.31520350068579E-15,0.707106781186546));
#16443=DIRECTION('',(1.,1.11022302462513E-14,0.));
#16444=DIRECTION('',(-1.,-1.11022302462516E-14,0.));
#16445=DIRECTION('center_axis',(-1.0345260002189E-14,1.,0.));
#16446=DIRECTION('ref_axis',(-1.,-1.0345260002189E-14,0.));
#16447=DIRECTION('',(1.,1.11022302462513E-14,0.));
#16448=DIRECTION('',(-1.,-1.11022302462516E-14,0.));
#16449=DIRECTION('center_axis',(-1.0345260002189E-14,1.,0.));
#16450=DIRECTION('ref_axis',(-1.,-1.0345260002189E-14,0.));
#16451=DIRECTION('',(1.,1.11022302462513E-14,0.));
#16452=DIRECTION('',(-1.,-1.11022302462516E-14,0.));
#16453=DIRECTION('center_axis',(-1.0345260002189E-14,1.,0.));
#16454=DIRECTION('ref_axis',(-1.,-1.0345260002189E-14,0.));
#16455=DIRECTION('',(1.,1.11022302462513E-14,0.));
#16456=DIRECTION('',(-1.,-1.11022302462516E-14,0.));
#16457=DIRECTION('center_axis',(-1.0345260002189E-14,1.,0.));
#16458=DIRECTION('ref_axis',(-1.,-1.0345260002189E-14,0.));
#16459=DIRECTION('center_axis',(1.0345260002189E-14,-1.,0.));
#16460=DIRECTION('ref_axis',(1.,1.0345260002189E-14,0.));
#16461=DIRECTION('',(-0.707106781186544,-7.31520350068574E-15,-0.70710678118655));
#16462=DIRECTION('',(0.707106781186549,7.31520350068579E-15,-0.707106781186546));
#16463=DIRECTION('',(0.707106781186549,7.31520350068578E-15,0.707106781186546));
#16464=DIRECTION('',(-0.707106781186551,-7.31520350068581E-15,0.707106781186544));
#16465=DIRECTION('',(1.,1.11022302462513E-14,0.));
#16466=DIRECTION('center_axis',(-1.0345260002189E-14,1.,0.));
#16467=DIRECTION('ref_axis',(-1.,-1.0345260002189E-14,0.));
#16468=DIRECTION('',(-1.,-1.11022302462516E-14,0.));
#16469=DIRECTION('',(1.,1.11022302462513E-14,0.));
#16470=DIRECTION('center_axis',(-1.0345260002189E-14,1.,0.));
#16471=DIRECTION('ref_axis',(-1.,-1.0345260002189E-14,0.));
#16472=DIRECTION('',(-1.,-1.11022302462516E-14,0.));
#16473=DIRECTION('',(1.,1.11022302462513E-14,0.));
#16474=DIRECTION('center_axis',(-1.0345260002189E-14,1.,0.));
#16475=DIRECTION('ref_axis',(-1.,-1.0345260002189E-14,0.));
#16476=DIRECTION('',(-1.,-1.11022302462516E-14,0.));
#16477=DIRECTION('',(1.,1.11022302462513E-14,0.));
#16478=DIRECTION('center_axis',(-1.0345260002189E-14,1.,0.));
#16479=DIRECTION('ref_axis',(-1.,-1.0345260002189E-14,0.));
#16480=DIRECTION('',(-1.,-1.11022302462516E-14,0.));
#16481=DIRECTION('center_axis',(0.,0.,-1.));
#16482=DIRECTION('ref_axis',(-1.,0.,0.));
#16483=DIRECTION('',(-1.0345260002189E-14,1.,0.));
#16484=DIRECTION('center_axis',(-1.0345260002189E-14,1.,0.));
#16485=DIRECTION('ref_axis',(1.,1.0345260002189E-14,-1.54206576648375E-14));
#16486=DIRECTION('',(-1.0345260002189E-14,1.,0.));
#16487=DIRECTION('center_axis',(0.,0.,1.));
#16488=DIRECTION('ref_axis',(1.,0.,0.));
#16489=DIRECTION('center_axis',(0.,0.,-1.));
#16490=DIRECTION('ref_axis',(-1.,0.,0.));
#16491=DIRECTION('',(-1.0345260002189E-14,1.,0.));
#16492=DIRECTION('center_axis',(-1.0345260002189E-14,1.,0.));
#16493=DIRECTION('ref_axis',(1.,1.0345260002189E-14,-3.43024899888577E-15));
#16494=DIRECTION('',(-1.0345260002189E-14,1.,0.));
#16495=DIRECTION('center_axis',(0.,0.,1.));
#16496=DIRECTION('ref_axis',(1.,0.,0.));
#16497=DIRECTION('center_axis',(0.,0.,-1.));
#16498=DIRECTION('ref_axis',(-1.,0.,0.));
#16499=DIRECTION('',(-1.0345260002189E-14,1.,0.));
#16500=DIRECTION('center_axis',(-1.0345260002189E-14,1.,0.));
#16501=DIRECTION('ref_axis',(1.,1.0345260002189E-14,-3.43024899888577E-15));
#16502=DIRECTION('',(-1.0345260002189E-14,1.,0.));
#16503=DIRECTION('center_axis',(0.,0.,1.));
#16504=DIRECTION('ref_axis',(1.,0.,0.));
#16505=DIRECTION('center_axis',(0.,0.,-1.));
#16506=DIRECTION('ref_axis',(-1.,0.,0.));
#16507=DIRECTION('',(-1.0345260002189E-14,1.,0.));
#16508=DIRECTION('center_axis',(-1.0345260002189E-14,1.,0.));
#16509=DIRECTION('ref_axis',(1.,1.0345260002189E-14,-1.54206576648375E-14));
#16510=DIRECTION('',(-1.0345260002189E-14,1.,0.));
#16511=DIRECTION('center_axis',(0.,0.,1.));
#16512=DIRECTION('ref_axis',(1.,0.,0.));
#16513=DIRECTION('center_axis',(0.707106781186551,7.34018225370516E-15,
-0.707106781186545));
#16514=DIRECTION('ref_axis',(1.03805852802452E-14,-1.,-1.32348907848756E-23));
#16515=DIRECTION('center_axis',(0.707106781186546,7.34018223498815E-15,
0.707106781186549));
#16516=DIRECTION('ref_axis',(1.03805852802452E-14,-1.,-1.32348895751129E-23));
#16517=DIRECTION('center_axis',(-0.707106781186546,-7.34018225370512E-15,
0.707106781186549));
#16518=DIRECTION('ref_axis',(1.03805852802452E-14,-1.,-1.3234889647637E-23));
#16519=DIRECTION('center_axis',(-0.707106781186544,-7.34018223498813E-15,
-0.707106781186551));
#16520=DIRECTION('ref_axis',(1.03805852802452E-14,-1.,-1.3234890851888E-23));
#16521=DIRECTION('center_axis',(0.,1.,-1.54886929424668E-30));
#16522=DIRECTION('ref_axis',(0.,1.54886929424668E-30,1.));
#16523=DIRECTION('center_axis',(-1.02244964895189E-14,1.,-1.57659325248097E-30));
#16524=DIRECTION('ref_axis',(-1.,-1.02244964895189E-14,1.11669963790763E-45));
#16525=DIRECTION('',(0.,1.,-1.54886929424668E-30));
#16526=DIRECTION('center_axis',(0.,1.,-1.54886929424668E-30));
#16527=DIRECTION('ref_axis',(0.,1.54886929424668E-30,1.));
#16528=DIRECTION('center_axis',(0.,1.,-1.54886929424668E-30));
#16529=DIRECTION('ref_axis',(0.,1.54886929424668E-30,1.));
#16530=DIRECTION('center_axis',(-1.02244964895189E-14,1.,-1.57659325248097E-30));
#16531=DIRECTION('ref_axis',(-1.,-1.02244964895189E-14,1.11669963790763E-45));
#16532=DIRECTION('',(0.,1.,-1.54886929424668E-30));
#16533=DIRECTION('center_axis',(0.,1.,-1.54886929424668E-30));
#16534=DIRECTION('ref_axis',(0.,1.54886929424668E-30,1.));
#16535=DIRECTION('center_axis',(1.,1.00583182218564E-14,1.5419764230905E-16));
#16536=DIRECTION('ref_axis',(-1.00583182218564E-14,1.,-8.58115691226271E-47));
#16537=DIRECTION('',(-7.00327082348719E-15,0.707106781186548,-0.707106781186548));
#16538=DIRECTION('',(1.5419764230905E-16,0.,-1.));
#16539=DIRECTION('',(7.2213392205266E-15,-0.707106781186548,-0.707106781186548));
#16540=DIRECTION('',(1.5419764230905E-16,0.,-1.));
#16541=DIRECTION('center_axis',(1.5419764230905E-16,1.,2.37769128936696E-32));
#16542=DIRECTION('ref_axis',(-1.,1.5419764230905E-16,0.));
#16543=DIRECTION('',(-1.,1.5419764230905E-16,-3.08395284618099E-16));
#16544=DIRECTION('',(1.5419764230905E-16,0.,-1.));
#16545=DIRECTION('',(1.,-1.5419764230905E-16,4.20834312723671E-32));
#16546=DIRECTION('center_axis',(1.5419764230905E-16,0.,-1.));
#16547=DIRECTION('ref_axis',(-1.,0.,-1.5419764230905E-16));
#16548=DIRECTION('center_axis',(1.35884999659177E-14,-0.707106781186556,
-0.70710678118654));
#16549=DIRECTION('ref_axis',(7.81974184165328E-13,0.70710678118654,-0.707106781186556));
#16550=DIRECTION('',(1.5419764230905E-16,0.,-1.));
#16551=DIRECTION('center_axis',(-3.88242856169051E-15,-0.707106781186542,
0.707106781186553));
#16552=DIRECTION('ref_axis',(1.03154041315431E-12,-0.707106781186553,-0.707106781186542));
#16553=DIRECTION('center_axis',(-0.986391978972164,0.164410656039619,-1.52099317550065E-16));
#16554=DIRECTION('ref_axis',(-0.164410656039619,-0.986391978972164,-3.75602913472012E-33));
#16555=DIRECTION('',(-0.117049568370783,-0.702246181386632,0.702246181386632));
#16556=DIRECTION('',(1.5419764230905E-16,0.,-1.));
#16557=DIRECTION('',(0.117049568370782,0.702246181386632,0.702246181386632));
#16558=DIRECTION('center_axis',(1.5419764230905E-16,0.,-1.));
#16559=DIRECTION('ref_axis',(-1.,0.,-1.5419764230905E-16));
#16560=DIRECTION('center_axis',(7.18968252164918E-15,0.707106781186545,
0.70710678118655));
#16561=DIRECTION('ref_axis',(7.1847046487102E-14,-0.70710678118655,0.707106781186545));
#16562=DIRECTION('',(1.5419764230905E-16,0.,-1.));
#16563=DIRECTION('center_axis',(2.93339046883292E-14,0.70710678118655,-0.707106781186545));
#16564=DIRECTION('ref_axis',(-2.48050675356169E-14,0.707106781186545,0.70710678118655));
#16565=DIRECTION('center_axis',(-1.02244964895189E-14,1.,-1.57659325248097E-30));
#16566=DIRECTION('ref_axis',(-1.,-1.02244964895189E-14,0.));
#16567=DIRECTION('',(-1.,-1.02244964895189E-14,1.00702988472098E-14));
#16568=DIRECTION('',(1.5419764230905E-16,0.,-1.));
#16569=DIRECTION('',(1.,1.02244964895189E-14,1.03786941318279E-14));
#16570=DIRECTION('center_axis',(1.5419764230905E-16,0.,-1.));
#16571=DIRECTION('ref_axis',(-1.,0.,-1.5419764230905E-16));
#16572=DIRECTION('center_axis',(7.90865077381428E-15,0.707106781186547,
0.707106781186548));
#16573=DIRECTION('ref_axis',(1.11137487371557E-13,-0.707106781186548,0.707106781186547));
#16574=DIRECTION('',(1.5419764230905E-16,0.,-1.));
#16575=DIRECTION('center_axis',(-1.4379365043298E-15,0.707106781186546,
-0.707106781186549));
#16576=DIRECTION('ref_axis',(1.95860265341088E-13,0.707106781186549,0.707106781186546));
#16577=DIRECTION('center_axis',(0.986391978972161,0.16441065603964,1.52099317550065E-16));
#16578=DIRECTION('ref_axis',(-0.16441065603964,0.986391978972161,2.47052149569693E-33));
#16579=DIRECTION('',(-0.117049568370797,0.702246181386631,-0.702246181386631));
#16580=DIRECTION('',(1.5419764230905E-16,0.,-1.));
#16581=DIRECTION('',(0.117049568370797,-0.702246181386631,-0.702246181386631));
#16582=DIRECTION('center_axis',(1.5419764230905E-16,0.,-1.));
#16583=DIRECTION('ref_axis',(-1.,0.,-1.5419764230905E-16));
#16584=DIRECTION('center_axis',(4.24155320364734E-14,-0.707106781186531,
-0.707106781186564));
#16585=DIRECTION('ref_axis',(-3.16030793522856E-12,0.707106781186564,-0.707106781186531));
#16586=DIRECTION('',(1.5419764230905E-16,0.,-1.));
#16587=DIRECTION('center_axis',(3.88242856169019E-15,-0.707106781186542,
0.707106781186553));
#16588=DIRECTION('ref_axis',(-2.80400082562096E-12,-0.707106781186553,-0.707106781186542));
#16589=DIRECTION('center_axis',(1.5419764230905E-16,1.,2.37769128936696E-32));
#16590=DIRECTION('ref_axis',(-1.,1.5419764230905E-16,0.));
#16591=DIRECTION('',(-1.,1.5419764230905E-16,-3.08395284618099E-16));
#16592=DIRECTION('',(1.5419764230905E-16,0.,-1.));
#16593=DIRECTION('',(1.,-1.5419764230905E-16,4.20834312723671E-32));
#16594=DIRECTION('center_axis',(-1.,-1.00583182218564E-14,-1.5419764230905E-16));
#16595=DIRECTION('ref_axis',(1.00583182218564E-14,-1.,8.58115691226271E-47));
#16596=DIRECTION('',(7.00327082348719E-15,-0.707106781186548,0.707106781186548));
#16597=DIRECTION('',(1.5419764230905E-16,0.,-1.));
#16598=DIRECTION('',(-7.2213392205266E-15,0.707106781186548,0.707106781186548));
#16599=DIRECTION('center_axis',(1.00447015340375E-14,-1.,1.54886929424668E-30));
#16600=DIRECTION('ref_axis',(1.,1.00447015340375E-14,0.));
#16601=DIRECTION('',(1.,1.00447015340375E-14,-9.89050389172848E-15));
#16602=DIRECTION('',(-1.,-1.00447015340375E-14,-1.01988991763466E-14));
#16603=DIRECTION('center_axis',(-1.09034198519707E-16,-0.707106781186547,
0.707106781186548));
#16604=DIRECTION('ref_axis',(2.24898714345845E-34,-0.707106781186548,-0.707106781186547));
#16605=DIRECTION('center_axis',(1.09034198519707E-16,-0.707106781186547,
-0.707106781186548));
#16606=DIRECTION('ref_axis',(-2.32788945572025E-33,0.707106781186548,-0.707106781186547));
#16607=DIRECTION('center_axis',(-2.46519032881566E-32,1.,-9.82547376793264E-15));
#16608=DIRECTION('ref_axis',(-1.41407071595279E-47,9.82547376793264E-15,
1.));
#16609=DIRECTION('center_axis',(2.7856650715617E-30,1.,1.00475183728577E-14));
#16610=DIRECTION('ref_axis',(-2.21644180929503E-45,-1.00475183728577E-14,
1.));
#16611=DIRECTION('',(-2.46519032881566E-32,1.,-9.82547376793264E-15));
#16612=DIRECTION('center_axis',(-2.46519032881566E-32,1.,-9.82547376793264E-15));
#16613=DIRECTION('ref_axis',(-1.41407071595279E-47,9.82547376793264E-15,
1.));
#16614=DIRECTION('center_axis',(-2.46519032881566E-32,1.,-9.82547376793264E-15));
#16615=DIRECTION('ref_axis',(-1.41407071595279E-47,9.82547376793264E-15,
1.));
#16616=DIRECTION('center_axis',(2.7856650715617E-30,1.,1.00475183728577E-14));
#16617=DIRECTION('ref_axis',(-2.21644180929503E-45,-1.00475183728577E-14,
1.));
#16618=DIRECTION('',(-2.46519032881566E-32,1.,-9.82547376793264E-15));
#16619=DIRECTION('center_axis',(-2.46519032881566E-32,1.,-9.82547376793264E-15));
#16620=DIRECTION('ref_axis',(-1.41407071595279E-47,9.82547376793264E-15,
1.));
#16621=DIRECTION('center_axis',(-2.71170936169723E-30,-1.,-9.82547376793264E-15));
#16622=DIRECTION('ref_axis',(0.,9.82547376793264E-15,-1.));
#16623=DIRECTION('',(3.13467930853623E-16,-9.82547376793264E-15,1.));
#16624=DIRECTION('',(-1.,2.715561221586E-32,2.77555756156289E-16));
#16625=DIRECTION('',(3.13467930853623E-16,-9.82547376793264E-15,1.));
#16626=DIRECTION('',(-1.,2.715561221586E-32,2.77555756156289E-16));
#16627=DIRECTION('center_axis',(-2.77555756156289E-16,-6.10622663543836E-16,
-1.));
#16628=DIRECTION('ref_axis',(-2.46519032881566E-32,1.,-6.10622663543836E-16));
#16629=DIRECTION('',(6.12323399573677E-17,-1.,6.10622663543836E-16));
#16630=DIRECTION('',(-1.,2.715561221586E-32,2.77555756156289E-16));
#16631=DIRECTION('',(6.12323399573677E-17,-1.,6.10622663543836E-16));
#16632=DIRECTION('center_axis',(-1.,2.715561221586E-32,2.77555756156289E-16));
#16633=DIRECTION('ref_axis',(2.77555756156289E-16,-7.53719648245999E-48,
1.));
#16634=DIRECTION('center_axis',(1.,6.12323399573675E-17,-3.13467930853623E-16));
#16635=DIRECTION('ref_axis',(3.13467930853623E-16,-1.43147286699433E-32,
1.));
#16636=DIRECTION('',(-1.,2.715561221586E-32,2.77555756156289E-16));
#16637=DIRECTION('center_axis',(1.,6.12323399573675E-17,-3.13467930853623E-16));
#16638=DIRECTION('ref_axis',(3.13467930853623E-16,1.91943749077616E-32,
1.));
#16639=DIRECTION('center_axis',(2.7856650715617E-30,1.,1.00475183728577E-14));
#16640=DIRECTION('ref_axis',(0.,-1.00475183728577E-14,1.));
#16641=DIRECTION('',(-3.13467930853624E-16,1.00475183728577E-14,-1.));
#16642=DIRECTION('',(-1.,2.715561221586E-32,2.77555756156289E-16));
#16643=DIRECTION('',(-3.13467930853624E-16,1.00475183728577E-14,-1.));
#16644=DIRECTION('center_axis',(-1.,2.715561221586E-32,2.77555756156289E-16));
#16645=DIRECTION('ref_axis',(2.77555756156289E-16,-7.53719648245999E-48,
1.));
#16646=DIRECTION('center_axis',(-1.,-6.12323399573675E-17,3.13467930853623E-16));
#16647=DIRECTION('ref_axis',(-3.13467930853623E-16,3.10928443355873E-33,
-1.));
#16648=DIRECTION('',(-1.,2.715561221586E-32,2.77555756156289E-16));
#16649=DIRECTION('center_axis',(-1.,-6.12323399573675E-17,3.13467930853623E-16));
#16650=DIRECTION('ref_axis',(-3.13467930853623E-16,-1.91943749077616E-32,
-1.));
#16651=DIRECTION('center_axis',(-2.77555756156289E-16,1.0991207943789E-14,
-1.));
#16652=DIRECTION('ref_axis',(-2.46519032881566E-32,1.,1.0991207943789E-14));
#16653=DIRECTION('',(6.1232339957364E-17,-1.,-1.0991207943789E-14));
#16654=DIRECTION('',(-1.,2.715561221586E-32,2.77555756156289E-16));
#16655=DIRECTION('',(6.1232339957364E-17,-1.,-1.0991207943789E-14));
#16656=DIRECTION('center_axis',(-1.,2.715561221586E-32,2.77555756156289E-16));
#16657=DIRECTION('ref_axis',(2.77555756156289E-16,-7.53719648245999E-48,
1.));
#16658=DIRECTION('center_axis',(1.,6.12323399573675E-17,-3.13467930853623E-16));
#16659=DIRECTION('ref_axis',(-3.13467930853623E-16,1.43147286699433E-32,
-1.));
#16660=DIRECTION('',(-1.,2.715561221586E-32,2.77555756156289E-16));
#16661=DIRECTION('center_axis',(1.,6.12323399573675E-17,-3.13467930853623E-16));
#16662=DIRECTION('ref_axis',(-3.13467930853623E-16,-1.91943749077616E-32,
-1.));
#16663=DIRECTION('center_axis',(-1.97215226305253E-31,1.,-6.10622663543836E-16));
#16664=DIRECTION('ref_axis',(-2.46519032881566E-32,6.10622663543836E-16,
1.));
#16665=DIRECTION('',(-3.13467930852236E-16,-6.10622663543836E-16,-1.));
#16666=DIRECTION('',(-1.,2.715561221586E-32,2.77555756156289E-16));
#16667=DIRECTION('',(-3.13467930852236E-16,-6.10622663543836E-16,-1.));
#16668=DIRECTION('center_axis',(2.77555756156289E-16,-1.02695629777827E-14,
1.));
#16669=DIRECTION('ref_axis',(2.46519032881566E-32,-1.,-1.02695629777827E-14));
#16670=DIRECTION('',(-6.12323399573645E-17,1.,1.02695629777827E-14));
#16671=DIRECTION('',(-6.12323399573645E-17,1.,1.02695629777827E-14));
#16672=DIRECTION('center_axis',(-1.,-6.12323399573675E-17,3.13467930853623E-16));
#16673=DIRECTION('ref_axis',(-3.13467930853623E-16,-6.10622663543836E-16,
-1.));
#16674=DIRECTION('center_axis',(-1.,-6.12323399573675E-17,3.13467930853623E-16));
#16675=DIRECTION('ref_axis',(-3.13467930853623E-16,-6.10622663543836E-16,
-1.));
#16676=DIRECTION('center_axis',(0.,1.,-9.82547376793264E-15));
#16677=DIRECTION('ref_axis',(0.,9.82547376793264E-15,1.));
#16678=DIRECTION('center_axis',(2.7856650715617E-30,1.,-1.01030295240889E-14));
#16679=DIRECTION('ref_axis',(2.37107728436212E-45,1.01030295240889E-14,
1.));
#16680=DIRECTION('',(0.,1.,-9.82547376793264E-15));
#16681=DIRECTION('center_axis',(0.,1.,-9.82547376793264E-15));
#16682=DIRECTION('ref_axis',(0.,9.82547376793264E-15,1.));
#16683=DIRECTION('center_axis',(0.,1.,-9.82547376793264E-15));
#16684=DIRECTION('ref_axis',(0.,9.82547376793264E-15,1.));
#16685=DIRECTION('center_axis',(2.7856650715617E-30,1.,-1.01030295240889E-14));
#16686=DIRECTION('ref_axis',(2.37107728436212E-45,1.01030295240889E-14,
1.));
#16687=DIRECTION('',(0.,1.,-9.82547376793264E-15));
#16688=DIRECTION('center_axis',(0.,1.,-9.82547376793264E-15));
#16689=DIRECTION('ref_axis',(0.,9.82547376793264E-15,1.));
#16690=DIRECTION('center_axis',(-2.71170936169723E-30,-1.,9.82547376793264E-15));
#16691=DIRECTION('ref_axis',(0.,9.82547376793264E-15,1.));
#16692=DIRECTION('',(3.13467930853623E-16,-9.82547376793264E-15,-1.));
#16693=DIRECTION('',(-1.,-8.66668474974256E-33,-2.77555756156289E-16));
#16694=DIRECTION('',(3.13467930853623E-16,-9.82547376793264E-15,-1.));
#16695=DIRECTION('',(-1.,-8.66668474974256E-33,-2.77555756156289E-16));
#16696=DIRECTION('center_axis',(-2.77555756156289E-16,-6.10622663543836E-16,
1.));
#16697=DIRECTION('ref_axis',(0.,1.,6.10622663543836E-16));
#16698=DIRECTION('',(6.12323399573677E-17,-1.,-6.10622663543836E-16));
#16699=DIRECTION('',(6.12323399573677E-17,-1.,-6.10622663543836E-16));
#16700=DIRECTION('',(-1.,-8.66668474974256E-33,-2.77555756156289E-16));
#16701=DIRECTION('center_axis',(-1.,-8.66668474974256E-33,-2.77555756156289E-16));
#16702=DIRECTION('ref_axis',(2.77555756156289E-16,2.40548823908298E-48,
-1.));
#16703=DIRECTION('center_axis',(-1.,-6.12323399573675E-17,-3.13467930853623E-16));
#16704=DIRECTION('ref_axis',(3.13467930853623E-16,-1.43147286699433E-32,
-1.));
#16705=DIRECTION('center_axis',(-1.,-6.12323399573675E-17,-3.13467930853623E-16));
#16706=DIRECTION('ref_axis',(3.13467930853623E-16,1.91943749077616E-32,
-1.));
#16707=DIRECTION('',(-1.,-8.66668474974256E-33,-2.77555756156289E-16));
#16708=DIRECTION('center_axis',(2.7856650715617E-30,1.,-1.01030295240889E-14));
#16709=DIRECTION('ref_axis',(2.46519032881566E-32,-1.01030295240889E-14,
-1.));
#16710=DIRECTION('',(-3.13467930853624E-16,1.01030295240889E-14,1.));
#16711=DIRECTION('',(-3.13467930853624E-16,1.01030295240889E-14,1.));
#16712=DIRECTION('',(-1.,-8.66668474974256E-33,-2.77555756156289E-16));
#16713=DIRECTION('center_axis',(-1.,-8.66668474974256E-33,-2.77555756156289E-16));
#16714=DIRECTION('ref_axis',(2.77555756156289E-16,2.40548823908298E-48,
-1.));
#16715=DIRECTION('center_axis',(1.,6.12323399573675E-17,3.13467930853623E-16));
#16716=DIRECTION('ref_axis',(-3.13467930853623E-16,3.10928443355873E-33,
1.));
#16717=DIRECTION('center_axis',(1.,6.12323399573675E-17,3.13467930853623E-16));
#16718=DIRECTION('ref_axis',(-3.13467930853623E-16,-1.91943749077616E-32,
1.));
#16719=DIRECTION('',(-1.,-8.66668474974256E-33,-2.77555756156289E-16));
#16720=DIRECTION('center_axis',(-2.77555756156289E-16,1.0991207943789E-14,
1.));
#16721=DIRECTION('ref_axis',(-2.46519032881566E-32,1.,-1.0991207943789E-14));
#16722=DIRECTION('',(6.1232339957364E-17,-1.,1.0991207943789E-14));
#16723=DIRECTION('',(6.1232339957364E-17,-1.,1.0991207943789E-14));
#16724=DIRECTION('',(-1.,-8.66668474974256E-33,-2.77555756156289E-16));
#16725=DIRECTION('center_axis',(-1.,-8.66668474974256E-33,-2.77555756156289E-16));
#16726=DIRECTION('ref_axis',(2.77555756156289E-16,2.40548823908298E-48,
-1.));
#16727=DIRECTION('center_axis',(-1.,-6.12323399573675E-17,-3.13467930853623E-16));
#16728=DIRECTION('ref_axis',(-3.13467930853623E-16,1.43147286699433E-32,
1.));
#16729=DIRECTION('center_axis',(-1.,-6.12323399573675E-17,-3.13467930853623E-16));
#16730=DIRECTION('ref_axis',(-3.13467930853623E-16,-1.91943749077616E-32,
1.));
#16731=DIRECTION('',(-1.,-8.66668474974256E-33,-2.77555756156289E-16));
#16732=DIRECTION('center_axis',(-1.72563323017096E-31,1.,6.10622663543836E-16));
#16733=DIRECTION('ref_axis',(4.86173068582901E-63,6.10622663543836E-16,
-1.));
#16734=DIRECTION('',(-3.13467930852236E-16,-6.10622663543836E-16,1.));
#16735=DIRECTION('',(-3.13467930852236E-16,-6.10622663543836E-16,1.));
#16736=DIRECTION('',(-1.,-8.66668474974256E-33,-2.77555756156289E-16));
#16737=DIRECTION('center_axis',(2.77555756156289E-16,-1.02695629777827E-14,
-1.));
#16738=DIRECTION('ref_axis',(0.,-1.,1.02695629777827E-14));
#16739=DIRECTION('',(-6.12323399573645E-17,1.,-1.02695629777827E-14));
#16740=DIRECTION('',(-6.12323399573645E-17,1.,-1.02695629777827E-14));
#16741=DIRECTION('center_axis',(-1.,-6.12323399573675E-17,-3.13467930853623E-16));
#16742=DIRECTION('ref_axis',(-3.13467930853623E-16,-6.10622663543836E-16,
1.));
#16743=DIRECTION('center_axis',(-1.,-6.12323399573675E-17,-3.13467930853623E-16));
#16744=DIRECTION('ref_axis',(-3.13467930853623E-16,-6.10622663543836E-16,
1.));
#25857=CARTESIAN_POINT('',(0.,0.,0.));
#25858=CARTESIAN_POINT('Origin',(38.0492,-76.2,-180.));
#25859=CARTESIAN_POINT('',(0.,-76.2,180.));
#25860=CARTESIAN_POINT('',(38.0492,-76.2,180.));
#25861=CARTESIAN_POINT('',(38.0492,-76.2,180.));
#25862=CARTESIAN_POINT('',(0.,-76.2,-180.));
#25863=CARTESIAN_POINT('',(0.,-76.2,-180.));
#25864=CARTESIAN_POINT('',(38.0492,-76.2,-180.));
#25865=CARTESIAN_POINT('',(38.0492,-76.2,-180.));
#25866=CARTESIAN_POINT('',(38.0492,-76.2,-180.));
#25867=CARTESIAN_POINT('Origin',(0.,-76.2,-180.));
#25868=CARTESIAN_POINT('',(0.,-74.042335135838,180.));
#25869=CARTESIAN_POINT('',(0.,-76.2,180.));
#25870=CARTESIAN_POINT('',(0.,-74.042335135838,-180.));
#25871=CARTESIAN_POINT('',(0.,-74.042335135838,-180.));
#25872=CARTESIAN_POINT('',(0.,-76.2,-180.));
#25873=CARTESIAN_POINT('Origin',(2.54,-74.042335135838,-180.));
#25874=CARTESIAN_POINT('',(2.12239693365934,-71.5368995092487,180.));
#25875=CARTESIAN_POINT('Origin',(2.54,-74.042335135838,180.));
#25876=CARTESIAN_POINT('',(2.12239693365934,-71.5368995092487,-180.));
#25877=CARTESIAN_POINT('',(2.12239693365934,-71.5368995092487,-180.));
#25878=CARTESIAN_POINT('Origin',(2.54,-74.042335135838,-180.));
#25879=CARTESIAN_POINT('Origin',(25.7655282791198,-67.5960901573836,-180.));
#25880=CARTESIAN_POINT('',(25.7655282791198,-67.5960901573836,180.));
#25881=CARTESIAN_POINT('',(25.7655282791198,-67.5960901573836,180.));
#25882=CARTESIAN_POINT('',(25.7655282791198,-67.5960901573836,-180.));
#25883=CARTESIAN_POINT('',(25.7655282791198,-67.5960901573836,-180.));
#25884=CARTESIAN_POINT('',(25.7655282791198,-67.5960901573836,-180.));
#25885=CARTESIAN_POINT('Origin',(24.638,-60.8314139655925,-180.));
#25886=CARTESIAN_POINT('',(31.496,-60.8314139655925,180.));
#25887=CARTESIAN_POINT('Origin',(24.638,-60.8314139655925,180.));
#25888=CARTESIAN_POINT('',(31.496,-60.8314139655925,-180.));
#25889=CARTESIAN_POINT('',(31.496,-60.8314139655925,-180.));
#25890=CARTESIAN_POINT('Origin',(24.638,-60.8314139655925,-180.));
#25891=CARTESIAN_POINT('Origin',(31.496,-15.3685860344075,-180.));
#25892=CARTESIAN_POINT('',(31.496,-15.3685860344075,180.));
#25893=CARTESIAN_POINT('',(31.496,-15.3685860344075,180.));
#25894=CARTESIAN_POINT('',(31.496,-15.3685860344075,-180.));
#25895=CARTESIAN_POINT('',(31.496,-15.3685860344075,-180.));
#25896=CARTESIAN_POINT('',(31.496,-15.3685860344075,-180.));
#25897=CARTESIAN_POINT('Origin',(24.638,-15.3685860344075,-180.));
#25898=CARTESIAN_POINT('',(25.7655282791198,-8.60390984261643,180.));
#25899=CARTESIAN_POINT('Origin',(24.638,-15.3685860344075,180.));
#25900=CARTESIAN_POINT('',(25.7655282791198,-8.60390984261643,-180.));
#25901=CARTESIAN_POINT('',(25.7655282791198,-8.60390984261643,-180.));
#25902=CARTESIAN_POINT('Origin',(24.638,-15.3685860344075,-180.));
#25903=CARTESIAN_POINT('Origin',(25.7655282791198,-8.60390984261643,-180.));
#25904=CARTESIAN_POINT('',(2.12239693365934,-4.66310049075127,180.));
#25905=CARTESIAN_POINT('',(25.7655282791198,-8.60390984261642,180.));
#25906=CARTESIAN_POINT('',(2.12239693365934,-4.66310049075127,-180.));
#25907=CARTESIAN_POINT('',(2.12239693365934,-4.66310049075127,-180.));
#25908=CARTESIAN_POINT('',(25.7655282791198,-8.60390984261643,-180.));
#25909=CARTESIAN_POINT('Origin',(2.54,-2.15766486416198,-180.));
#25910=CARTESIAN_POINT('',(0.,-2.15766486416198,180.));
#25911=CARTESIAN_POINT('Origin',(2.54,-2.15766486416198,180.));
#25912=CARTESIAN_POINT('',(0.,-2.15766486416198,-180.));
#25913=CARTESIAN_POINT('',(0.,-2.15766486416198,-180.));
#25914=CARTESIAN_POINT('Origin',(2.54,-2.15766486416198,-180.));
#25915=CARTESIAN_POINT('Origin',(0.,0.,-180.));
#25916=CARTESIAN_POINT('',(0.,0.,180.));
#25917=CARTESIAN_POINT('',(0.,0.,180.));
#25918=CARTESIAN_POINT('',(0.,0.,-180.));
#25919=CARTESIAN_POINT('',(0.,0.,-180.));
#25920=CARTESIAN_POINT('',(0.,0.,-180.));
#25921=CARTESIAN_POINT('Origin',(38.0492,0.,-180.));
#25922=CARTESIAN_POINT('',(38.0492,0.,180.));
#25923=CARTESIAN_POINT('',(38.0492,0.,180.));
#25924=CARTESIAN_POINT('',(38.0492,0.,-180.));
#25925=CARTESIAN_POINT('',(38.0492,0.,-180.));
#25926=CARTESIAN_POINT('',(38.0492,0.,-180.));
#25927=CARTESIAN_POINT('Origin',(38.0492,-76.2,-180.));
#25928=CARTESIAN_POINT('',(38.0492,-76.2,180.));
#25929=CARTESIAN_POINT('',(38.0492,-76.2,-180.));
#25930=CARTESIAN_POINT('Origin',(0.,-76.2,-180.));
#25931=CARTESIAN_POINT('Origin',(-3.46944695195361E-15,0.,180.));
#25932=CARTESIAN_POINT('Origin',(38.0491999999999,-76.2,-180.));
#25933=CARTESIAN_POINT('',(38.0491999999999,-76.2,180.));
#25934=CARTESIAN_POINT('',(38.0491999999999,-74.042335135838,180.));
#25935=CARTESIAN_POINT('',(38.0491999999999,-76.2,180.));
#25936=CARTESIAN_POINT('',(38.0491999999999,-71.5368995092488,177.877603066341));
#25937=CARTESIAN_POINT('Origin',(38.0491999999999,-74.042335135838,177.46));
#25938=CARTESIAN_POINT('',(38.0491999999999,-67.5960901573836,154.23447172088));
#25939=CARTESIAN_POINT('',(38.0491999999999,-67.5960901573836,154.23447172088));
#25940=CARTESIAN_POINT('',(38.0491999999999,-60.8314139655925,148.504));
#25941=CARTESIAN_POINT('Origin',(38.0491999999999,-60.8314139655925,155.362));
#25942=CARTESIAN_POINT('',(38.0491999999999,-15.3685860344075,148.504));
#25943=CARTESIAN_POINT('',(38.0491999999999,-15.3685860344075,148.504));
#25944=CARTESIAN_POINT('',(38.0491999999999,-8.6039098426164,154.23447172088));
#25945=CARTESIAN_POINT('Origin',(38.0491999999999,-15.3685860344075,155.362));
#25946=CARTESIAN_POINT('',(38.0491999999999,-4.66310049075123,177.877603066341));
#25947=CARTESIAN_POINT('',(38.0491999999999,-8.6039098426164,154.23447172088));
#25948=CARTESIAN_POINT('',(38.0491999999999,-2.15766486416195,180.));
#25949=CARTESIAN_POINT('Origin',(38.0491999999999,-2.15766486416195,177.46));
#25950=CARTESIAN_POINT('',(38.0491999999999,3.46944695195361E-14,180.));
#25951=CARTESIAN_POINT('',(38.0491999999999,3.46944695195361E-14,180.));
#25952=CARTESIAN_POINT('',(38.0491999999999,2.08166817117217E-14,141.9508));
#25953=CARTESIAN_POINT('',(38.0491999999999,2.08166817117217E-14,-180.));
#25954=CARTESIAN_POINT('',(38.0491999999999,-76.2,141.9508));
#25955=CARTESIAN_POINT('',(38.0491999999999,-76.2,141.9508));
#25956=CARTESIAN_POINT('',(38.0491999999999,-76.2,-180.));
#25957=CARTESIAN_POINT('Origin',(-1.38777878078145E-13,-76.2,141.9508));
#25958=CARTESIAN_POINT('',(332.282278663992,1.38777878078145E-14,141.9508));
#25959=CARTESIAN_POINT('',(-8.32667268468867E-14,3.46944695195361E-14,141.9508));
#25960=CARTESIAN_POINT('',(332.282278663992,-76.2,141.9508));
#25961=CARTESIAN_POINT('',(332.282278663992,-76.2,141.9508));
#25962=CARTESIAN_POINT('',(-1.38777878078145E-13,-76.2,141.9508));
#25963=CARTESIAN_POINT('Origin',(-8.32667268468867E-14,3.46944695195361E-14,
141.9508));
#25964=CARTESIAN_POINT('',(340.,3.46944695195361E-14,180.));
#25965=CARTESIAN_POINT('',(-1.11022302462516E-13,4.16333634234434E-14,180.));
#25966=CARTESIAN_POINT('',(319.151687711983,2.77555756156289E-14,77.2155679930824));
#25967=CARTESIAN_POINT('Origin',(-1.11022302462516E-13,4.16333634234434E-14,
180.));
#25968=CARTESIAN_POINT('',(340.,-2.15766486416195,180.));
#25969=CARTESIAN_POINT('',(-1.38777878078145E-13,-2.15766486416193,180.));
#25970=CARTESIAN_POINT('',(340.,3.46944695195361E-14,180.));
#25971=CARTESIAN_POINT('Origin',(-1.66533453693773E-13,-2.15766486416194,
177.46));
#25972=CARTESIAN_POINT('',(339.569502956741,-4.66310049075124,177.877603066341));
#25973=CARTESIAN_POINT('',(-1.66533453693773E-13,-4.66310049075123,177.877603066341));
#25974=CARTESIAN_POINT('Origin',(339.484798308677,-2.15766486416141,177.459999999999));
#25975=CARTESIAN_POINT('Origin',(-1.66533453693773E-13,-8.6039098426164,
154.23447172088));
#25976=CARTESIAN_POINT('',(334.773841044403,-8.60390984261639,154.23447172088));
#25977=CARTESIAN_POINT('',(-1.66533453693773E-13,-8.6039098426164,154.23447172088));
#25978=CARTESIAN_POINT('',(321.888621689571,-19.1922694606555,90.7089481977025));
#25979=CARTESIAN_POINT('Origin',(-1.11022302462516E-13,-15.3685860344075,
155.362));
#25980=CARTESIAN_POINT('',(333.611499027604,-15.3685860344075,148.504));
#25981=CARTESIAN_POINT('',(-1.11022302462516E-13,-15.3685860344075,148.504));
#25982=CARTESIAN_POINT('Origin',(335.002543594174,-15.3685860344077,155.362));
#25983=CARTESIAN_POINT('Origin',(-1.11022302462516E-13,-15.3685860344075,
148.504));
#25984=CARTESIAN_POINT('',(333.611499027604,-60.8314139655925,148.504));
#25985=CARTESIAN_POINT('',(-2.77555756156289E-14,-60.8314139655925,148.504));
#25986=CARTESIAN_POINT('',(333.611499027604,-15.3685860344075,148.504));
#25987=CARTESIAN_POINT('Origin',(-1.38777878078145E-13,-60.8314139655925,
155.362));
#25988=CARTESIAN_POINT('',(334.773841044404,-67.5960901573836,154.23447172088));
#25989=CARTESIAN_POINT('',(-1.94289029309402E-13,-67.5960901573836,154.23447172088));
#25990=CARTESIAN_POINT('Origin',(335.002543594174,-60.8314139655902,155.362000000003));
#25991=CARTESIAN_POINT('Origin',(-1.94289029309402E-13,-67.5960901573836,
154.23447172088));
#25992=CARTESIAN_POINT('',(339.569502956741,-71.5368995092488,177.877603066341));
#25993=CARTESIAN_POINT('',(-1.66533453693773E-13,-71.5368995092487,177.877603066341));
#25994=CARTESIAN_POINT('',(321.888621689571,-57.0077305393445,90.7089481977025));
#25995=CARTESIAN_POINT('Origin',(-8.32667268468867E-14,-74.042335135838,
177.46));
#25996=CARTESIAN_POINT('',(340.,-74.042335135838,180.));
#25997=CARTESIAN_POINT('',(-8.32667268468867E-14,-74.042335135838,180.));
#25998=CARTESIAN_POINT('Origin',(339.484798308678,-74.0423351358383,177.46));
#25999=CARTESIAN_POINT('Origin',(-1.38777878078145E-13,-76.2,180.));
#26000=CARTESIAN_POINT('',(340.,-76.2,180.));
#26001=CARTESIAN_POINT('',(-1.38777878078145E-13,-76.2,180.));
#26002=CARTESIAN_POINT('',(340.,-76.2,180.));
#26003=CARTESIAN_POINT('Origin',(-1.38777878078145E-13,-76.2,141.9508));
#26004=CARTESIAN_POINT('',(319.151687711983,-76.2,77.2155679930824));
#26005=CARTESIAN_POINT('Origin',(334.54009041727,-38.0999999999999,153.08205587497));
#26006=CARTESIAN_POINT('Origin',(334.54009041727,-38.0999999999999,153.08205587497));
#26007=CARTESIAN_POINT('',(340.,-2.15766486416197,180.));
#26008=CARTESIAN_POINT('',(340.,-2.77555756156289E-14,180.));
#26009=CARTESIAN_POINT('',(340.,-3.67761376907083E-13,180.));
#26010=CARTESIAN_POINT('',(332.282278663992,2.42861286636753E-13,141.9508));
#26011=CARTESIAN_POINT('',(327.009283962862,4.16333634234434E-13,115.954366435321));
#26012=CARTESIAN_POINT('',(332.282278663992,-76.1999999999997,141.9508));
#26013=CARTESIAN_POINT('',(332.282278663992,4.85722573273506E-14,141.9508));
#26014=CARTESIAN_POINT('',(340.,-76.2,180.));
#26015=CARTESIAN_POINT('',(327.009283962862,-76.1999999999995,115.954366435321));
#26016=CARTESIAN_POINT('',(340.,-74.042335135838,180.));
#26017=CARTESIAN_POINT('',(340.,-76.2,180.));
#26018=CARTESIAN_POINT('',(339.56950295674,-71.5368995092487,177.87760306634));
#26019=CARTESIAN_POINT('Origin',(339.484798308677,-74.0423351358391,177.459999999999));
#26020=CARTESIAN_POINT('',(334.773841044403,-67.5960901573834,154.23447172088));
#26021=CARTESIAN_POINT('',(329.541995367165,-63.2968491455564,128.44090728968));
#26022=CARTESIAN_POINT('',(333.611499027603,-60.8314139655923,148.504));
#26023=CARTESIAN_POINT('Origin',(335.002543594174,-60.831413965591,155.362000000001));
#26024=CARTESIAN_POINT('',(333.611499027603,-15.3685860344073,148.504));
#26025=CARTESIAN_POINT('',(333.611499027603,-60.8314139655925,148.504));
#26026=CARTESIAN_POINT('',(334.773841044403,-8.60390984261626,154.23447172088));
#26027=CARTESIAN_POINT('Origin',(335.002543594174,-15.3685860344086,155.362000000001));
#26028=CARTESIAN_POINT('',(339.56950295674,-4.66310049075126,177.877603066341));
#26029=CARTESIAN_POINT('',(329.541995367166,-12.9031508544429,128.44090728968));
#26030=CARTESIAN_POINT('Origin',(339.484798308676,-2.1576648641567,177.459999999994));
#26031=CARTESIAN_POINT('Origin',(455.174510060656,2.4980018054066E-13,89.9579328706422));
#26032=CARTESIAN_POINT('',(462.282278663992,2.56739074444567E-13,86.9508));
#26033=CARTESIAN_POINT('',(455.174510060656,2.4980018054066E-13,89.9579328706422));
#26034=CARTESIAN_POINT('',(462.282278663992,-76.1999999999997,86.9507999999995));
#26035=CARTESIAN_POINT('',(462.282278663992,2.70616862252382E-13,86.9508));
#26036=CARTESIAN_POINT('',(455.174510060656,-76.1999999999997,89.9579328706417));
#26037=CARTESIAN_POINT('Origin',(455.174510060656,-76.1999999999997,89.9579328706417));
#26038=CARTESIAN_POINT('',(470.,-76.2,125.));
#26039=CARTESIAN_POINT('',(462.587255030328,-76.1999999999997,88.4543664353206));
#26040=CARTESIAN_POINT('',(470.,-76.2,125.));
#26041=CARTESIAN_POINT('Origin',(470.,-76.2,125.));
#26042=CARTESIAN_POINT('',(470.,-74.042335135838,125.));
#26043=CARTESIAN_POINT('',(470.,-76.2,125.));
#26044=CARTESIAN_POINT('',(470.,-74.042335135838,125.));
#26045=CARTESIAN_POINT('Origin',(469.010314423275,-74.042335135838,122.660743182285));
#26046=CARTESIAN_POINT('',(469.569502956741,-71.5368995092487,122.87760306634));
#26047=CARTESIAN_POINT('Origin',(469.484798308677,-74.0423351358414,122.459999999996));
#26048=CARTESIAN_POINT('',(469.173029278217,-71.5368995092487,123.045341930331));
#26049=CARTESIAN_POINT('Origin',(459.960719797421,-67.5960901573834,101.270792248449));
#26050=CARTESIAN_POINT('',(464.773841044404,-67.5960901573834,99.2344717208798));
#26051=CARTESIAN_POINT('',(464.974992377841,-67.7613851824375,100.226169526879));
#26052=CARTESIAN_POINT('',(459.960719797421,-67.5960901573834,101.270792248449));
#26053=CARTESIAN_POINT('Origin',(460.400049905765,-60.8314139655923,102.309208868173));
#26054=CARTESIAN_POINT('',(463.611499027604,-60.8314139655922,93.5039999999996));
#26055=CARTESIAN_POINT('Origin',(465.002543594174,-60.8314139655914,100.362000000001));
#26056=CARTESIAN_POINT('',(457.727898848607,-60.8314139655922,95.9932154603443));
#26057=CARTESIAN_POINT('Origin',(457.727898848607,-60.8314139655922,95.9932154603443));
#26058=CARTESIAN_POINT('',(463.611499027604,-15.3685860344073,93.5039999999999));
#26059=CARTESIAN_POINT('',(463.611499027604,-60.8314139655922,93.5039999999996));
#26060=CARTESIAN_POINT('',(457.727898848607,-15.3685860344073,95.9932154603446));
#26061=CARTESIAN_POINT('Origin',(460.400049905766,-15.3685860344074,102.309208868173));
#26062=CARTESIAN_POINT('',(464.773841044404,-8.60390984261627,99.2344717208802));
#26063=CARTESIAN_POINT('Origin',(465.002543594175,-15.3685860344111,100.362000000004));
#26064=CARTESIAN_POINT('',(459.960719797421,-8.60390984261627,101.27079224845));
#26065=CARTESIAN_POINT('Origin',(459.960719797421,-8.60390984261625,101.27079224845));
#26066=CARTESIAN_POINT('',(469.569502956741,-4.66310049075126,122.877603066341));
#26067=CARTESIAN_POINT('',(464.974992377841,-8.43861481756216,100.226169526879));
#26068=CARTESIAN_POINT('',(469.173029278217,-4.66310049075127,123.045341930331));
#26069=CARTESIAN_POINT('Origin',(469.010314423275,-2.15766486416197,122.660743182286));
#26070=CARTESIAN_POINT('',(470.,-2.15766486416197,125.));
#26071=CARTESIAN_POINT('Origin',(469.484798308679,-2.15766486416684,122.460000000005));
#26072=CARTESIAN_POINT('',(470.,-2.15766486416197,125.));
#26073=CARTESIAN_POINT('Origin',(470.,6.93889390390723E-15,125.));
#26074=CARTESIAN_POINT('',(470.,6.93889390390723E-15,125.));
#26075=CARTESIAN_POINT('',(470.,6.93889390390723E-15,125.));
#26076=CARTESIAN_POINT('',(470.,6.93889390390723E-15,125.));
#26077=CARTESIAN_POINT('Origin',(455.174510060656,2.4980018054066E-13,89.9579328706422));
#26078=CARTESIAN_POINT('',(462.587255030328,2.35922392732846E-13,88.4543664353211));
#26079=CARTESIAN_POINT('Origin',(464.54009041727,-38.0999999999998,98.0820558749701));
#26080=CARTESIAN_POINT('Origin',(720.,2.70616862252382E-13,86.9508));
#26081=CARTESIAN_POINT('',(681.9508,1.38777878078145E-14,125.));
#26082=CARTESIAN_POINT('',(681.9508,1.38777878078145E-14,86.9507999999998));
#26083=CARTESIAN_POINT('',(681.9508,1.38777878078145E-14,125.));
#26084=CARTESIAN_POINT('',(462.282278663992,2.70616862252382E-13,86.9508));
#26085=CARTESIAN_POINT('',(720.,2.70616862252382E-13,86.9508));
#26086=CARTESIAN_POINT('',(470.,1.38777878078145E-14,125.));
#26087=CARTESIAN_POINT('',(472.466348646758,-6.93889390390723E-14,137.159365289908));
#26088=CARTESIAN_POINT('',(720.,1.38777878078145E-14,125.));
#26089=CARTESIAN_POINT('Origin',(720.,1.38777878078145E-14,125.));
#26090=CARTESIAN_POINT('',(681.9508,-2.15766486416195,125.));
#26091=CARTESIAN_POINT('',(681.9508,1.38777878078145E-14,125.));
#26092=CARTESIAN_POINT('',(470.,-2.15766486416195,125.));
#26093=CARTESIAN_POINT('',(470.,6.17561557447743E-13,125.));
#26094=CARTESIAN_POINT('',(720.,-2.15766486416194,125.));
#26095=CARTESIAN_POINT('Origin',(720.,-2.15766486416195,122.46));
#26096=CARTESIAN_POINT('',(681.9508,-4.66310049075124,122.877603066341));
#26097=CARTESIAN_POINT('Origin',(681.9508,-2.15766486416194,122.46));
#26098=CARTESIAN_POINT('',(469.569502956741,-4.66310049075123,122.877603066341));
#26099=CARTESIAN_POINT('Origin',(469.484798308678,-2.15766486416211,122.46));
#26100=CARTESIAN_POINT('',(720.,-4.66310049075125,122.877603066341));
#26101=CARTESIAN_POINT('Origin',(720.,-8.60390984261621,99.2344717208803));
#26102=CARTESIAN_POINT('',(681.9508,-8.60390984261625,99.2344717208803));
#26103=CARTESIAN_POINT('',(681.9508,-8.60390984261622,99.2344717208803));
#26104=CARTESIAN_POINT('',(464.773841044404,-8.60390984261625,99.2344717208803));
#26105=CARTESIAN_POINT('',(474.597323766275,-0.531515815288028,147.665302857156));
#26106=CARTESIAN_POINT('',(720.,-8.60390984261624,99.2344717208803));
#26107=CARTESIAN_POINT('Origin',(720.,-15.3685860344074,100.362));
#26108=CARTESIAN_POINT('',(681.9508,-15.3685860344073,93.504));
#26109=CARTESIAN_POINT('Origin',(681.9508,-15.3685860344074,100.362));
#26110=CARTESIAN_POINT('',(463.611499027604,-15.3685860344073,93.504));
#26111=CARTESIAN_POINT('Origin',(465.002543594174,-15.368586034407,100.362));
#26112=CARTESIAN_POINT('',(720.,-15.3685860344073,93.504));
#26113=CARTESIAN_POINT('Origin',(720.,-60.8314139655922,93.5039999999996));
#26114=CARTESIAN_POINT('',(681.9508,-60.8314139655923,93.5039999999997));
#26115=CARTESIAN_POINT('',(681.9508,-60.8314139655923,93.5039999999996));
#26116=CARTESIAN_POINT('',(463.611499027604,-60.8314139655923,93.5039999999996));
#26117=CARTESIAN_POINT('',(463.611499027604,-60.8314139655919,93.5039999999996));
#26118=CARTESIAN_POINT('',(720.,-60.8314139655922,93.5039999999996));
#26119=CARTESIAN_POINT('Origin',(720.,-60.8314139655923,100.362));
#26120=CARTESIAN_POINT('',(681.9508,-67.5960901573835,99.2344717208798));
#26121=CARTESIAN_POINT('Origin',(681.9508,-60.8314139655923,100.362));
#26122=CARTESIAN_POINT('',(464.773841044404,-67.5960901573835,99.2344717208798));
#26123=CARTESIAN_POINT('Origin',(465.002543594175,-60.8314139655898,100.362000000003));
#26124=CARTESIAN_POINT('',(720.,-67.5960901573835,99.2344717208798));
#26125=CARTESIAN_POINT('Origin',(720.,-67.5960901573835,99.2344717208798));
#26126=CARTESIAN_POINT('',(681.9508,-71.5368995092487,122.87760306634));
#26127=CARTESIAN_POINT('',(681.9508,-67.5960901573835,99.2344717208798));
#26128=CARTESIAN_POINT('',(469.569502956741,-71.5368995092487,122.87760306634));
#26129=CARTESIAN_POINT('',(474.597323766275,-75.6684841847123,147.665302857156));
#26130=CARTESIAN_POINT('',(720.,-71.5368995092487,122.87760306634));
#26131=CARTESIAN_POINT('Origin',(720.,-74.0423351358381,122.46));
#26132=CARTESIAN_POINT('',(681.9508,-74.042335135838,125.));
#26133=CARTESIAN_POINT('Origin',(681.9508,-74.042335135838,122.46));
#26134=CARTESIAN_POINT('',(470.,-74.042335135838,125.));
#26135=CARTESIAN_POINT('Origin',(469.484798308678,-74.042335135835,122.460000000003));
#26136=CARTESIAN_POINT('',(720.,-74.042335135838,125.));
#26137=CARTESIAN_POINT('Origin',(720.,-76.2,125.));
#26138=CARTESIAN_POINT('',(681.9508,-76.2,125.));
#26139=CARTESIAN_POINT('',(681.9508,-76.2,125.));
#26140=CARTESIAN_POINT('',(470.,-76.2,125.));
#26141=CARTESIAN_POINT('',(470.,-76.2,125.));
#26142=CARTESIAN_POINT('',(720.,-76.2,125.));
#26143=CARTESIAN_POINT('Origin',(720.,-76.1999999999998,86.9507999999995));
#26144=CARTESIAN_POINT('',(681.9508,-76.1999999999997,86.9507999999995));
#26145=CARTESIAN_POINT('',(681.9508,-76.2,125.));
#26146=CARTESIAN_POINT('',(462.282278663992,-76.1999999999997,86.9507999999995));
#26147=CARTESIAN_POINT('',(472.466348646758,-76.2000000000001,137.159365289908));
#26148=CARTESIAN_POINT('',(720.,-76.1999999999998,86.9507999999995));
#26149=CARTESIAN_POINT('Origin',(720.,2.70616862252382E-13,86.9508));
#26150=CARTESIAN_POINT('',(681.9508,2.77555756156289E-13,86.9508));
#26151=CARTESIAN_POINT('',(462.282278663992,6.45317133063372E-13,86.9508));
#26152=CARTESIAN_POINT('Origin',(464.54009041727,-38.0999999999998,98.0820558749701));
#26153=CARTESIAN_POINT('Origin',(681.9508,-76.2,125.));
#26154=CARTESIAN_POINT('Origin',(681.9508,-76.2,125.));
#26155=CARTESIAN_POINT('',(720.,-76.2,-125.));
#26156=CARTESIAN_POINT('',(681.9508,-76.2,-125.));
#26157=CARTESIAN_POINT('',(681.9508,-76.2,-125.));
#26158=CARTESIAN_POINT('',(720.,-76.2,125.));
#26159=CARTESIAN_POINT('',(720.,-76.2,125.));
#26160=CARTESIAN_POINT('',(681.9508,-76.2,125.));
#26161=CARTESIAN_POINT('',(681.9508,-76.2,125.));
#26162=CARTESIAN_POINT('',(681.9508,-76.2,125.));
#26163=CARTESIAN_POINT('Origin',(720.,-76.2,125.));
#26164=CARTESIAN_POINT('',(720.,-74.042335135838,-125.));
#26165=CARTESIAN_POINT('',(720.,-76.2,-125.));
#26166=CARTESIAN_POINT('',(720.,-74.042335135838,125.));
#26167=CARTESIAN_POINT('',(720.,-74.042335135838,125.));
#26168=CARTESIAN_POINT('',(720.,-76.2,125.));
#26169=CARTESIAN_POINT('Origin',(717.46,-74.042335135838,125.));
#26170=CARTESIAN_POINT('',(717.877603066341,-71.5368995092487,-125.));
#26171=CARTESIAN_POINT('Origin',(717.46,-74.042335135838,-125.));
#26172=CARTESIAN_POINT('',(717.877603066341,-71.5368995092487,125.));
#26173=CARTESIAN_POINT('',(717.877603066341,-71.5368995092487,125.));
#26174=CARTESIAN_POINT('Origin',(717.46,-74.042335135838,125.));
#26175=CARTESIAN_POINT('Origin',(694.23447172088,-67.5960901573836,125.));
#26176=CARTESIAN_POINT('',(694.23447172088,-67.5960901573835,-125.));
#26177=CARTESIAN_POINT('',(694.23447172088,-67.5960901573836,-125.));
#26178=CARTESIAN_POINT('',(694.23447172088,-67.5960901573835,125.));
#26179=CARTESIAN_POINT('',(694.23447172088,-67.5960901573835,125.));
#26180=CARTESIAN_POINT('',(694.23447172088,-67.5960901573836,125.));
#26181=CARTESIAN_POINT('Origin',(695.362,-60.8314139655925,125.));
#26182=CARTESIAN_POINT('',(688.504,-60.8314139655925,-125.));
#26183=CARTESIAN_POINT('Origin',(695.362,-60.8314139655925,-125.));
#26184=CARTESIAN_POINT('',(688.504,-60.8314139655925,125.));
#26185=CARTESIAN_POINT('',(688.504,-60.8314139655925,125.));
#26186=CARTESIAN_POINT('Origin',(695.362,-60.8314139655925,125.));
#26187=CARTESIAN_POINT('Origin',(688.504,-15.3685860344075,125.));
#26188=CARTESIAN_POINT('',(688.504,-15.3685860344075,-125.));
#26189=CARTESIAN_POINT('',(688.504,-15.3685860344075,-125.));
#26190=CARTESIAN_POINT('',(688.504,-15.3685860344075,125.));
#26191=CARTESIAN_POINT('',(688.504,-15.3685860344075,125.));
#26192=CARTESIAN_POINT('',(688.504,-15.3685860344075,125.));
#26193=CARTESIAN_POINT('Origin',(695.362,-15.3685860344075,125.));
#26194=CARTESIAN_POINT('',(694.23447172088,-8.60390984261643,-125.));
#26195=CARTESIAN_POINT('Origin',(695.362,-15.3685860344075,-125.));
#26196=CARTESIAN_POINT('',(694.23447172088,-8.60390984261643,125.));
#26197=CARTESIAN_POINT('',(694.23447172088,-8.60390984261643,125.));
#26198=CARTESIAN_POINT('Origin',(695.362,-15.3685860344075,125.));
#26199=CARTESIAN_POINT('Origin',(694.23447172088,-8.60390984261643,125.));
#26200=CARTESIAN_POINT('',(717.877603066341,-4.66310049075127,-125.));
#26201=CARTESIAN_POINT('',(694.23447172088,-8.60390984261643,-125.));
#26202=CARTESIAN_POINT('',(717.877603066341,-4.66310049075127,125.));
#26203=CARTESIAN_POINT('',(717.877603066341,-4.66310049075127,125.));
#26204=CARTESIAN_POINT('',(694.23447172088,-8.60390984261643,125.));
#26205=CARTESIAN_POINT('Origin',(717.46,-2.15766486416198,125.));
#26206=CARTESIAN_POINT('',(720.,-2.15766486416198,-125.));
#26207=CARTESIAN_POINT('Origin',(717.46,-2.15766486416198,-125.));
#26208=CARTESIAN_POINT('',(720.,-2.15766486416198,125.));
#26209=CARTESIAN_POINT('',(720.,-2.15766486416198,125.));
#26210=CARTESIAN_POINT('Origin',(717.46,-2.15766486416198,125.));
#26211=CARTESIAN_POINT('Origin',(720.,0.,125.));
#26212=CARTESIAN_POINT('',(720.,0.,-125.));
#26213=CARTESIAN_POINT('',(720.,0.,-125.));
#26214=CARTESIAN_POINT('',(720.,0.,125.));
#26215=CARTESIAN_POINT('',(720.,0.,125.));
#26216=CARTESIAN_POINT('',(720.,0.,125.));
#26217=CARTESIAN_POINT('Origin',(681.9508,0.,125.));
#26218=CARTESIAN_POINT('',(681.9508,0.,-125.));
#26219=CARTESIAN_POINT('',(681.9508,0.,-125.));
#26220=CARTESIAN_POINT('',(681.9508,0.,125.));
#26221=CARTESIAN_POINT('',(681.9508,0.,125.));
#26222=CARTESIAN_POINT('',(681.9508,0.,125.));
#26223=CARTESIAN_POINT('Origin',(681.9508,-76.2,125.));
#26224=CARTESIAN_POINT('',(681.9508,-76.2,-125.));
#26225=CARTESIAN_POINT('',(681.9508,-76.2,125.));
#26226=CARTESIAN_POINT('Origin',(720.,-76.2,125.));
#26227=CARTESIAN_POINT('Origin',(720.,0.,-125.));
#26228=CARTESIAN_POINT('Origin',(38.0491999999999,-76.2,-180.));
#26229=CARTESIAN_POINT('',(38.0491999999999,-74.042335135838,-180.));
#26230=CARTESIAN_POINT('',(38.0491999999999,-76.2,-180.));
#26231=CARTESIAN_POINT('',(38.0491999999999,-76.2,-180.));
#26232=CARTESIAN_POINT('',(38.0492,-76.2,-141.9508));
#26233=CARTESIAN_POINT('',(38.0491999999999,-76.2,-180.));
#26234=CARTESIAN_POINT('',(38.0491999999999,-1.38777878078145E-14,-141.9508));
#26235=CARTESIAN_POINT('',(38.0492,-76.2,-141.9508));
#26236=CARTESIAN_POINT('',(38.0491999999999,-6.93889390390723E-15,-180.));
#26237=CARTESIAN_POINT('',(38.0491999999999,-6.93889390390723E-15,-180.));
#26238=CARTESIAN_POINT('',(38.0491999999999,-2.15766486416197,-180.));
#26239=CARTESIAN_POINT('',(38.0491999999999,-6.93889390390723E-15,-180.));
#26240=CARTESIAN_POINT('',(38.0491999999999,-4.66310049075126,-177.877603066341));
#26241=CARTESIAN_POINT('Origin',(38.0491999999999,-2.15766486416196,-177.46));
#26242=CARTESIAN_POINT('',(38.0491999999999,-8.60390984261643,-154.23447172088));
#26243=CARTESIAN_POINT('',(38.0491999999999,-8.60390984261643,-154.23447172088));
#26244=CARTESIAN_POINT('',(38.0491999999999,-15.3685860344075,-148.504));
#26245=CARTESIAN_POINT('Origin',(38.0491999999998,-15.3685860344075,-155.362));
#26246=CARTESIAN_POINT('',(38.0492,-60.8314139655925,-148.504));
#26247=CARTESIAN_POINT('',(38.0491999999999,-15.3685860344075,-148.504));
#26248=CARTESIAN_POINT('',(38.0491999999999,-67.5960901573835,-154.23447172088));
#26249=CARTESIAN_POINT('Origin',(38.0491999999998,-60.8314139655925,-155.362));
#26250=CARTESIAN_POINT('',(38.0491999999999,-71.5368995092487,-177.877603066341));
#26251=CARTESIAN_POINT('',(38.0491999999999,-67.5960901573836,-154.23447172088));
#26252=CARTESIAN_POINT('Origin',(38.0491999999999,-74.042335135838,-177.46));
#26253=CARTESIAN_POINT('Origin',(340.,-76.2,-141.9508));
#26254=CARTESIAN_POINT('',(332.282278663993,-76.2,-141.9508));
#26255=CARTESIAN_POINT('',(340.,-76.2,-141.9508));
#26256=CARTESIAN_POINT('',(332.282278663993,0.,-141.9508));
#26257=CARTESIAN_POINT('',(332.282278663993,-76.2,-141.9508));
#26258=CARTESIAN_POINT('',(340.,-6.93889390390723E-15,-141.9508));
#26259=CARTESIAN_POINT('Origin',(340.,-6.93889390390723E-15,-141.9508));
#26260=CARTESIAN_POINT('',(340.,-6.93889390390723E-15,-180.));
#26261=CARTESIAN_POINT('',(332.587255030328,-6.93889390390723E-15,-143.454366435321));
#26262=CARTESIAN_POINT('',(340.,-6.93889390390723E-15,-180.));
#26263=CARTESIAN_POINT('Origin',(340.,-6.93889390390723E-15,-180.));
#26264=CARTESIAN_POINT('',(340.,-2.15766486416197,-180.));
#26265=CARTESIAN_POINT('',(340.,-6.93889390390723E-15,-180.));
#26266=CARTESIAN_POINT('',(340.,-2.15766486416197,-180.));
#26267=CARTESIAN_POINT('Origin',(340.,-2.15766486416197,-177.46));
#26268=CARTESIAN_POINT('',(339.569502956741,-4.66310049075126,-177.877603066341));
#26269=CARTESIAN_POINT('Origin',(339.484798308677,-2.15766486416006,-177.459999999998));
#26270=CARTESIAN_POINT('',(340.,-4.66310049075127,-177.877603066341));
#26271=CARTESIAN_POINT('Origin',(340.,-8.60390984261644,-154.23447172088));
#26272=CARTESIAN_POINT('',(334.773841044404,-8.60390984261644,-154.23447172088));
#26273=CARTESIAN_POINT('',(334.974992377842,-8.43861481756234,-155.226169526879));
#26274=CARTESIAN_POINT('',(340.,-8.60390984261644,-154.23447172088));
#26275=CARTESIAN_POINT('Origin',(340.,-15.3685860344075,-155.362));
#26276=CARTESIAN_POINT('',(333.611499027604,-15.3685860344075,-148.504));
#26277=CARTESIAN_POINT('Origin',(335.002543594174,-15.3685860344061,-155.361999999998));
#26278=CARTESIAN_POINT('',(340.,-15.3685860344075,-148.504));
#26279=CARTESIAN_POINT('Origin',(340.,-15.3685860344075,-148.504));
#26280=CARTESIAN_POINT('',(333.611499027604,-60.8314139655925,-148.504));
#26281=CARTESIAN_POINT('',(333.611499027604,-15.3685860344075,-148.504));
#26282=CARTESIAN_POINT('',(340.,-60.8314139655925,-148.504));
#26283=CARTESIAN_POINT('Origin',(340.,-60.8314139655925,-155.362));
#26284=CARTESIAN_POINT('',(334.773841044404,-67.5960901573836,-154.23447172088));
#26285=CARTESIAN_POINT('Origin',(335.002543594176,-60.8314139655898,-155.362000000003));
#26286=CARTESIAN_POINT('',(340.,-67.5960901573836,-154.23447172088));
#26287=CARTESIAN_POINT('Origin',(340.,-67.5960901573836,-154.23447172088));
#26288=CARTESIAN_POINT('',(339.569502956741,-71.5368995092487,-177.877603066341));
#26289=CARTESIAN_POINT('',(334.974992377842,-67.7613851824377,-155.226169526879));
#26290=CARTESIAN_POINT('',(340.,-71.5368995092487,-177.877603066341));
#26291=CARTESIAN_POINT('Origin',(340.,-74.042335135838,-177.46));
#26292=CARTESIAN_POINT('',(340.,-74.042335135838,-180.));
#26293=CARTESIAN_POINT('Origin',(339.484798308678,-74.0423351358367,-177.460000000001));
#26294=CARTESIAN_POINT('',(340.,-74.042335135838,-180.));
#26295=CARTESIAN_POINT('Origin',(340.,-76.2,-180.));
#26296=CARTESIAN_POINT('',(340.,-76.2,-180.));
#26297=CARTESIAN_POINT('',(340.,-76.2,-180.));
#26298=CARTESIAN_POINT('',(340.,-76.2,-180.));
#26299=CARTESIAN_POINT('Origin',(340.,-76.2,-141.9508));
#26300=CARTESIAN_POINT('',(332.587255030328,-76.2,-143.454366435321));
#26301=CARTESIAN_POINT('Origin',(334.540090417271,-38.1,-153.08205587497));
#26302=CARTESIAN_POINT('Origin',(720.,-76.2,-86.9508));
#26303=CARTESIAN_POINT('',(470.,-76.2,-125.));
#26304=CARTESIAN_POINT('',(462.282278663992,-76.2,-86.9508));
#26305=CARTESIAN_POINT('',(472.466348646758,-76.2000000000001,-137.159365289908));
#26306=CARTESIAN_POINT('',(681.9508,-76.2,-125.));
#26307=CARTESIAN_POINT('',(720.,-76.2,-125.));
#26308=CARTESIAN_POINT('',(681.9508,-76.2,-86.9508));
#26309=CARTESIAN_POINT('',(681.9508,-76.2,125.));
#26310=CARTESIAN_POINT('',(720.,-76.2,-86.9508));
#26311=CARTESIAN_POINT('Origin',(720.,-76.2,-125.));
#26312=CARTESIAN_POINT('',(470.,-74.0423351358381,-125.));
#26313=CARTESIAN_POINT('',(470.,-76.2,-125.));
#26314=CARTESIAN_POINT('',(681.9508,-74.0423351358381,-125.));
#26315=CARTESIAN_POINT('',(720.,-74.0423351358381,-125.));
#26316=CARTESIAN_POINT('',(681.9508,-76.2,-125.));
#26317=CARTESIAN_POINT('Origin',(720.,-74.0423351358381,-122.46));
#26318=CARTESIAN_POINT('',(469.569502956741,-71.5368995092488,-122.877603066341));
#26319=CARTESIAN_POINT('Origin',(469.484798308677,-74.0423351358409,-122.459999999996));
#26320=CARTESIAN_POINT('',(681.9508,-71.5368995092488,-122.877603066341));
#26321=CARTESIAN_POINT('',(720.,-71.5368995092488,-122.877603066341));
#26322=CARTESIAN_POINT('Origin',(681.9508,-74.0423351358381,-122.46));
#26323=CARTESIAN_POINT('Origin',(720.,-67.5960901573836,-99.2344717208803));
#26324=CARTESIAN_POINT('',(464.773841044404,-67.5960901573836,-99.2344717208803));
#26325=CARTESIAN_POINT('',(474.597323766275,-75.6684841847121,-147.665302857156));
#26326=CARTESIAN_POINT('',(681.9508,-67.5960901573836,-99.2344717208803));
#26327=CARTESIAN_POINT('',(720.,-67.5960901573836,-99.2344717208803));
#26328=CARTESIAN_POINT('',(681.9508,-67.5960901573836,-99.2344717208803));
#26329=CARTESIAN_POINT('Origin',(720.,-60.8314139655925,-100.362));
#26330=CARTESIAN_POINT('',(463.611499027604,-60.8314139655925,-93.504));
#26331=CARTESIAN_POINT('Origin',(465.002543594174,-60.8314139655921,-100.362));
#26332=CARTESIAN_POINT('',(681.9508,-60.8314139655925,-93.504));
#26333=CARTESIAN_POINT('',(720.,-60.8314139655925,-93.504));
#26334=CARTESIAN_POINT('Origin',(681.9508,-60.8314139655925,-100.362));
#26335=CARTESIAN_POINT('Origin',(720.,-15.3685860344075,-93.504));
#26336=CARTESIAN_POINT('',(463.611499027604,-15.3685860344075,-93.504));
#26337=CARTESIAN_POINT('',(463.611499027604,-15.3685860344075,-93.504));
#26338=CARTESIAN_POINT('',(681.9508,-15.3685860344075,-93.504));
#26339=CARTESIAN_POINT('',(720.,-15.3685860344075,-93.504));
#26340=CARTESIAN_POINT('',(681.9508,-15.3685860344075,-93.504));
#26341=CARTESIAN_POINT('Origin',(720.,-15.3685860344075,-100.362));
#26342=CARTESIAN_POINT('',(464.773841044404,-8.60390984261638,-99.2344717208803));
#26343=CARTESIAN_POINT('Origin',(465.002543594173,-15.3685860344047,-100.361999999996));
#26344=CARTESIAN_POINT('',(681.9508,-8.60390984261638,-99.2344717208803));
#26345=CARTESIAN_POINT('',(720.,-8.60390984261638,-99.2344717208803));
#26346=CARTESIAN_POINT('Origin',(681.9508,-15.3685860344075,-100.362));
#26347=CARTESIAN_POINT('Origin',(720.,-8.60390984261638,-99.2344717208803));
#26348=CARTESIAN_POINT('',(469.569502956741,-4.66310049075124,-122.877603066341));
#26349=CARTESIAN_POINT('',(474.597323766275,-0.531515815287868,-147.665302857156));
#26350=CARTESIAN_POINT('',(681.9508,-4.66310049075121,-122.877603066341));
#26351=CARTESIAN_POINT('',(720.,-4.66310049075124,-122.877603066341));
#26352=CARTESIAN_POINT('',(681.9508,-8.60390984261638,-99.2344717208803));
#26353=CARTESIAN_POINT('Origin',(720.,-2.15766486416195,-122.46));
#26354=CARTESIAN_POINT('',(470.,-2.15766486416193,-125.));
#26355=CARTESIAN_POINT('Origin',(469.484798308679,-2.15766486416409,-122.460000000003));
#26356=CARTESIAN_POINT('',(681.9508,-2.15766486416192,-125.));
#26357=CARTESIAN_POINT('',(720.,-2.15766486416193,-125.));
#26358=CARTESIAN_POINT('Origin',(681.9508,-2.15766486416193,-122.46));
#26359=CARTESIAN_POINT('Origin',(720.,3.46944695195361E-14,-125.));
#26360=CARTESIAN_POINT('',(470.,2.08166817117217E-14,-125.));
#26361=CARTESIAN_POINT('',(470.,2.08166817117217E-14,-125.));
#26362=CARTESIAN_POINT('',(681.9508,4.16333634234434E-14,-125.));
#26363=CARTESIAN_POINT('',(720.,3.46944695195361E-14,-125.));
#26364=CARTESIAN_POINT('',(681.9508,4.16333634234434E-14,-125.));
#26365=CARTESIAN_POINT('Origin',(720.,2.77555756156289E-14,-86.9508));
#26366=CARTESIAN_POINT('',(462.282278663992,3.46944695195361E-14,-86.9508));
#26367=CARTESIAN_POINT('',(472.466348646758,2.77555756156289E-14,-137.159365289909));
#26368=CARTESIAN_POINT('',(681.9508,3.46944695195361E-14,-86.9508));
#26369=CARTESIAN_POINT('',(720.,2.77555756156289E-14,-86.9508));
#26370=CARTESIAN_POINT('',(681.9508,4.16333634234434E-14,125.));
#26371=CARTESIAN_POINT('Origin',(720.,-76.2,-86.9508));
#26372=CARTESIAN_POINT('',(462.282278663992,-76.2,-86.9508));
#26373=CARTESIAN_POINT('',(681.9508,-76.2,-86.9508));
#26374=CARTESIAN_POINT('Origin',(681.9508,-76.2,125.));
#26375=CARTESIAN_POINT('Origin',(464.54009041727,-38.1,-98.0820558749705));
#26376=CARTESIAN_POINT('Origin',(334.54009041727,-38.1,-153.08205587497));
#26377=CARTESIAN_POINT('',(340.,-74.042335135838,-180.));
#26378=CARTESIAN_POINT('',(340.,-76.2,-180.));
#26379=CARTESIAN_POINT('',(340.,-76.2,-180.));
#26380=CARTESIAN_POINT('',(332.282278663993,-76.2,-141.9508));
#26381=CARTESIAN_POINT('',(327.009283962863,-76.2,-115.954366435321));
#26382=CARTESIAN_POINT('',(332.282278663993,0.,-141.9508));
#26383=CARTESIAN_POINT('',(332.282278663993,-76.2,-141.9508));
#26384=CARTESIAN_POINT('',(340.,0.,-180.));
#26385=CARTESIAN_POINT('',(327.009283962863,6.93889390390723E-15,-115.954366435321));
#26386=CARTESIAN_POINT('',(340.,-2.15766486416199,-180.));
#26387=CARTESIAN_POINT('',(340.,0.,-180.));
#26388=CARTESIAN_POINT('',(339.569502956741,-4.66310049075126,-177.877603066341));
#26389=CARTESIAN_POINT('Origin',(339.484798308678,-2.15766486416058,-177.459999999999));
#26390=CARTESIAN_POINT('',(334.773841044404,-8.60390984261643,-154.23447172088));
#26391=CARTESIAN_POINT('',(329.541995367166,-12.9031508544432,-128.44090728968));
#26392=CARTESIAN_POINT('',(333.611499027604,-15.3685860344076,-148.504));
#26393=CARTESIAN_POINT('Origin',(335.002543594175,-15.3685860344113,-155.362000000004));
#26394=CARTESIAN_POINT('',(333.611499027604,-60.8314139655925,-148.504));
#26395=CARTESIAN_POINT('',(333.611499027604,-15.3685860344076,-148.504));
#26396=CARTESIAN_POINT('',(334.773841044404,-67.5960901573836,-154.23447172088));
#26397=CARTESIAN_POINT('Origin',(335.002543594174,-60.8314139655924,-155.362));
#26398=CARTESIAN_POINT('',(339.569502956741,-71.5368995092487,-177.877603066341));
#26399=CARTESIAN_POINT('',(329.541995367166,-63.2968491455568,-128.44090728968));
#26400=CARTESIAN_POINT('Origin',(339.484798308678,-74.0423351358371,-177.460000000001));
#26401=CARTESIAN_POINT('Origin',(455.174510060656,-76.2,-89.9579328706422));
#26402=CARTESIAN_POINT('',(462.282278663992,-76.2,-86.9508));
#26403=CARTESIAN_POINT('',(455.174510060656,-76.2,-89.9579328706422));
#26404=CARTESIAN_POINT('',(462.282278663992,6.93889390390723E-15,-86.9508));
#26405=CARTESIAN_POINT('',(462.282278663992,-76.2,-86.9508));
#26406=CARTESIAN_POINT('',(455.174510060656,1.38777878078145E-14,-89.9579328706422));
#26407=CARTESIAN_POINT('Origin',(455.174510060656,1.38777878078145E-14,
-89.9579328706422));
#26408=CARTESIAN_POINT('',(470.,6.93889390390723E-15,-125.));
#26409=CARTESIAN_POINT('',(462.587255030328,0.,-88.4543664353211));
#26410=CARTESIAN_POINT('',(470.,6.93889390390723E-15,-125.));
#26411=CARTESIAN_POINT('Origin',(470.,6.93889390390723E-15,-125.));
#26412=CARTESIAN_POINT('',(470.,-2.15766486416199,-125.));
#26413=CARTESIAN_POINT('',(470.,6.93889390390723E-15,-125.));
#26414=CARTESIAN_POINT('',(470.,-2.15766486416199,-125.));
#26415=CARTESIAN_POINT('Origin',(469.010314423275,-2.15766486416197,-122.660743182286));
#26416=CARTESIAN_POINT('',(469.569502956741,-4.66310049075125,-122.877603066341));
#26417=CARTESIAN_POINT('Origin',(469.484798308679,-2.15766486416551,-122.460000000004));
#26418=CARTESIAN_POINT('',(469.173029278217,-4.66310049075125,-123.045341930331));
#26419=CARTESIAN_POINT('Origin',(459.960719797421,-8.60390984261642,-101.27079224845));
#26420=CARTESIAN_POINT('',(464.773841044404,-8.60390984261643,-99.2344717208803));
#26421=CARTESIAN_POINT('',(464.974992377841,-8.43861481756233,-100.226169526879));
#26422=CARTESIAN_POINT('',(459.960719797421,-8.60390984261642,-101.27079224845));
#26423=CARTESIAN_POINT('Origin',(460.400049905766,-15.3685860344075,-102.309208868173));
#26424=CARTESIAN_POINT('',(463.611499027604,-15.3685860344075,-93.504));
#26425=CARTESIAN_POINT('Origin',(465.002543594175,-15.3685860344098,-100.362000000003));
#26426=CARTESIAN_POINT('',(457.727898848607,-15.3685860344076,-95.9932154603446));
#26427=CARTESIAN_POINT('Origin',(457.727898848607,-15.3685860344076,-95.9932154603447));
#26428=CARTESIAN_POINT('',(463.611499027604,-60.8314139655925,-93.504));
#26429=CARTESIAN_POINT('',(463.611499027604,-15.3685860344075,-93.504));
#26430=CARTESIAN_POINT('',(457.727898848607,-60.8314139655924,-95.9932154603447));
#26431=CARTESIAN_POINT('Origin',(460.400049905766,-60.8314139655924,-102.309208868173));
#26432=CARTESIAN_POINT('',(464.773841044404,-67.5960901573836,-99.2344717208803));
#26433=CARTESIAN_POINT('Origin',(465.002543594174,-60.8314139655918,-100.362000000001));
#26434=CARTESIAN_POINT('',(459.960719797421,-67.5960901573836,-101.27079224845));
#26435=CARTESIAN_POINT('Origin',(459.960719797421,-67.5960901573836,-101.27079224845));
#26436=CARTESIAN_POINT('',(469.569502956741,-71.5368995092487,-122.877603066341));
#26437=CARTESIAN_POINT('',(464.974992377841,-67.7613851824377,-100.226169526879));
#26438=CARTESIAN_POINT('',(469.173029278217,-71.5368995092487,-123.045341930331));
#26439=CARTESIAN_POINT('Origin',(469.010314423275,-74.042335135838,-122.660743182286));
#26440=CARTESIAN_POINT('',(470.,-74.042335135838,-125.));
#26441=CARTESIAN_POINT('Origin',(469.484798308679,-74.0423351358312,-122.460000000008));
#26442=CARTESIAN_POINT('',(470.,-74.042335135838,-125.));
#26443=CARTESIAN_POINT('Origin',(470.,-76.2,-125.));
#26444=CARTESIAN_POINT('',(470.,-76.2,-125.));
#26445=CARTESIAN_POINT('',(470.,-76.2,-125.));
#26446=CARTESIAN_POINT('',(470.,-76.2,-125.));
#26447=CARTESIAN_POINT('Origin',(455.174510060656,-76.2,-89.9579328706422));
#26448=CARTESIAN_POINT('',(462.587255030328,-76.2,-88.4543664353211));
#26449=CARTESIAN_POINT('Origin',(464.54009041727,-38.1,-98.0820558749704));
#26450=CARTESIAN_POINT('Origin',(254.057664864162,-9.71445146547012E-14,
144.4908));
#26451=CARTESIAN_POINT('',(251.9,-1.38777878078145E-13,180.));
#26452=CARTESIAN_POINT('',(251.9,-1.11022302462516E-13,141.9508));
#26453=CARTESIAN_POINT('',(251.9,-1.38777878078145E-13,180.));
#26454=CARTESIAN_POINT('',(254.057664864162,-8.32667268468867E-14,141.9508));
#26455=CARTESIAN_POINT('',(251.9,-1.11022302462516E-13,141.9508));
#26456=CARTESIAN_POINT('',(256.563100490752,-9.71445146547012E-14,144.073196933659));
#26457=CARTESIAN_POINT('Origin',(254.057664864162,-9.71445146547012E-14,
144.4908));
#26458=CARTESIAN_POINT('',(260.503909842617,-9.71445146547012E-14,167.716328279119));
#26459=CARTESIAN_POINT('',(260.503909842617,-9.71445146547012E-14,167.716328279119));
#26460=CARTESIAN_POINT('',(267.268586034408,-8.32667268468867E-14,173.4468));
#26461=CARTESIAN_POINT('Origin',(267.268586034408,-1.11022302462516E-13,
166.5888));
#26462=CARTESIAN_POINT('',(312.731413965592,-1.11022302462516E-13,173.4468));
#26463=CARTESIAN_POINT('',(312.731413965592,-1.11022302462516E-13,173.4468));
#26464=CARTESIAN_POINT('',(319.496090157384,-8.32667268468867E-14,167.71632827912));
#26465=CARTESIAN_POINT('Origin',(312.731413965593,-5.55111512312578E-14,
166.5888));
#26466=CARTESIAN_POINT('',(323.436899509249,-9.71445146547012E-14,144.07319693366));
#26467=CARTESIAN_POINT('',(319.496090157384,-8.32667268468867E-14,167.71632827912));
#26468=CARTESIAN_POINT('',(325.942335135838,-1.11022302462516E-13,141.9508));
#26469=CARTESIAN_POINT('Origin',(325.942335135838,-8.32667268468867E-14,
144.4908));
#26470=CARTESIAN_POINT('',(328.1,-9.71445146547012E-14,141.9508));
#26471=CARTESIAN_POINT('',(328.1,-9.71445146547012E-14,141.9508));
#26472=CARTESIAN_POINT('',(328.1,-1.11022302462516E-13,180.));
#26473=CARTESIAN_POINT('',(328.1,-1.11022302462516E-13,180.));
#26474=CARTESIAN_POINT('',(251.9,-1.38777878078145E-13,180.));
#26475=CARTESIAN_POINT('Origin',(251.9,-1.38777878078145E-13,180.));
#26476=CARTESIAN_POINT('',(328.1,150.200000000001,180.));
#26477=CARTESIAN_POINT('',(328.1,-1.11022302462516E-13,180.));
#26478=CARTESIAN_POINT('',(251.9,150.2,180.));
#26479=CARTESIAN_POINT('',(251.899999999998,150.2,180.));
#26480=CARTESIAN_POINT('',(251.9,-1.38777878078145E-13,180.));
#26481=CARTESIAN_POINT('Origin',(328.1,-1.11022302462516E-13,180.));
#26482=CARTESIAN_POINT('',(328.1,112.1508,141.9508));
#26483=CARTESIAN_POINT('',(328.1,-9.71445146547012E-14,141.9508));
#26484=CARTESIAN_POINT('',(328.100000000001,75.1000000000002,104.9));
#26485=CARTESIAN_POINT('Origin',(328.1,-9.71445146547012E-14,141.9508));
#26486=CARTESIAN_POINT('',(325.942335135838,112.1508,141.9508));
#26487=CARTESIAN_POINT('',(325.942335135838,-1.11022302462516E-13,141.9508));
#26488=CARTESIAN_POINT('',(328.1,112.1508,141.9508));
#26489=CARTESIAN_POINT('Origin',(325.942335135838,-8.32667268468867E-14,
144.4908));
#26490=CARTESIAN_POINT('',(323.436899509249,114.27319693366,144.07319693366));
#26491=CARTESIAN_POINT('',(323.436899509249,-9.71445146547012E-14,144.07319693366));
#26492=CARTESIAN_POINT('Origin',(325.94233513584,114.690800000002,144.490800000002));
#26493=CARTESIAN_POINT('Origin',(319.496090157384,-8.32667268468867E-14,
167.71632827912));
#26494=CARTESIAN_POINT('',(319.496090157384,137.91632827912,167.71632827912));
#26495=CARTESIAN_POINT('',(319.496090157384,-8.32667268468867E-14,167.71632827912));
#26496=CARTESIAN_POINT('',(330.832483055846,69.9029324635591,99.7029324635591));
#26497=CARTESIAN_POINT('Origin',(312.731413965593,-5.55111512312578E-14,
166.5888));
#26498=CARTESIAN_POINT('',(312.731413965592,143.6468,173.4468));
#26499=CARTESIAN_POINT('',(312.731413965592,-1.11022302462516E-13,173.4468));
#26500=CARTESIAN_POINT('Origin',(312.731413965592,136.788799999999,166.588799999999));
#26501=CARTESIAN_POINT('Origin',(312.731413965592,-1.11022302462516E-13,
173.4468));
#26502=CARTESIAN_POINT('',(267.268586034408,143.6468,173.4468));
#26503=CARTESIAN_POINT('',(267.268586034408,-8.32667268468867E-14,173.4468));
#26504=CARTESIAN_POINT('',(312.731413965591,143.6468,173.4468));
#26505=CARTESIAN_POINT('Origin',(267.268586034408,-1.11022302462516E-13,
166.5888));
#26506=CARTESIAN_POINT('',(260.503909842617,137.91632827912,167.716328279119));
#26507=CARTESIAN_POINT('',(260.503909842617,-9.71445146547012E-14,167.716328279119));
#26508=CARTESIAN_POINT('Origin',(267.268586034407,136.788800000001,166.5888));
#26509=CARTESIAN_POINT('Origin',(260.503909842617,-9.71445146547012E-14,
167.716328279119));
#26510=CARTESIAN_POINT('',(256.563100490752,114.273196933659,144.073196933659));
#26511=CARTESIAN_POINT('',(256.563100490752,-9.71445146547012E-14,144.073196933659));
#26512=CARTESIAN_POINT('',(249.167516944156,69.9029324635586,99.7029324635585));
#26513=CARTESIAN_POINT('Origin',(254.057664864162,-9.71445146547012E-14,
144.4908));
#26514=CARTESIAN_POINT('',(254.057664864162,112.1508,141.9508));
#26515=CARTESIAN_POINT('',(254.057664864162,-8.32667268468867E-14,141.9508));
#26516=CARTESIAN_POINT('Origin',(254.057664864162,114.6908,144.4908));
#26517=CARTESIAN_POINT('Origin',(251.9,-1.11022302462516E-13,141.9508));
#26518=CARTESIAN_POINT('',(251.9,112.1508,141.9508));
#26519=CARTESIAN_POINT('',(251.9,-1.11022302462516E-13,141.9508));
#26520=CARTESIAN_POINT('',(251.9,112.1508,141.9508));
#26521=CARTESIAN_POINT('Origin',(251.9,-1.38777878078145E-13,180.));
#26522=CARTESIAN_POINT('',(251.900000000001,75.0999999999998,104.9));
#26523=CARTESIAN_POINT('Origin',(290.,139.06874412503,168.86874412503));
#26524=CARTESIAN_POINT('Origin',(254.057664864162,-6.93889390390723E-14,
-144.4908));
#26525=CARTESIAN_POINT('',(251.9,-6.93889390390723E-14,-180.));
#26526=CARTESIAN_POINT('',(251.9,-6.93889390390723E-14,-141.9508));
#26527=CARTESIAN_POINT('',(251.9,-6.93889390390723E-14,-180.));
#26528=CARTESIAN_POINT('',(328.1,-2.77555756156289E-14,-180.));
#26529=CARTESIAN_POINT('',(251.9,-6.93889390390723E-14,-180.));
#26530=CARTESIAN_POINT('',(328.100000000001,-2.77555756156289E-14,-141.9508));
#26531=CARTESIAN_POINT('',(328.1,-2.77555756156289E-14,-180.));
#26532=CARTESIAN_POINT('',(325.942335135839,-8.32667268468867E-14,-141.9508));
#26533=CARTESIAN_POINT('',(328.100000000001,-2.77555756156289E-14,-141.9508));
#26534=CARTESIAN_POINT('',(323.436899509249,-2.77555756156289E-14,-144.07319693366));
#26535=CARTESIAN_POINT('Origin',(325.942335135839,-5.55111512312578E-14,
-144.4908));
#26536=CARTESIAN_POINT('',(319.496090157384,-5.55111512312578E-14,-167.71632827912));
#26537=CARTESIAN_POINT('',(319.496090157384,-5.55111512312578E-14,-167.71632827912));
#26538=CARTESIAN_POINT('',(312.731413965593,-4.16333634234434E-14,-173.4468));
#26539=CARTESIAN_POINT('Origin',(312.731413965593,-5.55111512312578E-14,
-166.5888));
#26540=CARTESIAN_POINT('',(267.268586034408,-1.38777878078145E-14,-173.4468));
#26541=CARTESIAN_POINT('',(312.731413965593,-4.16333634234434E-14,-173.4468));
#26542=CARTESIAN_POINT('',(260.503909842617,-1.38777878078145E-14,-167.71632827912));
#26543=CARTESIAN_POINT('Origin',(267.268586034408,-5.55111512312578E-14,
-166.5888));
#26544=CARTESIAN_POINT('',(256.563100490752,-8.32667268468867E-14,-144.073196933659));
#26545=CARTESIAN_POINT('',(260.503909842617,-1.38777878078145E-14,-167.71632827912));
#26546=CARTESIAN_POINT('',(254.057664864163,-4.16333634234434E-14,-141.9508));
#26547=CARTESIAN_POINT('Origin',(254.057664864162,-6.93889390390723E-14,
-144.4908));
#26548=CARTESIAN_POINT('',(251.9,-6.93889390390723E-14,-141.9508));
#26549=CARTESIAN_POINT('Origin',(251.9,150.2,-180.));
#26550=CARTESIAN_POINT('',(251.9,150.2,-180.));
#26551=CARTESIAN_POINT('',(251.9,150.2,-180.));
#26552=CARTESIAN_POINT('',(328.1,150.2,-180.));
#26553=CARTESIAN_POINT('',(251.9,150.2,-180.));
#26554=CARTESIAN_POINT('',(328.1,150.2,-180.));
#26555=CARTESIAN_POINT('Origin',(328.1,150.2,-180.));
#26556=CARTESIAN_POINT('',(328.100000000001,112.1508,-141.9508));
#26557=CARTESIAN_POINT('',(328.1,150.2,-180.));
#26558=CARTESIAN_POINT('',(328.100000000001,150.2,-141.9508));
#26559=CARTESIAN_POINT('Origin',(328.100000000001,150.2,-141.9508));
#26560=CARTESIAN_POINT('',(325.942335135839,112.1508,-141.9508));
#26561=CARTESIAN_POINT('',(328.100000000001,112.1508,-141.9508));
#26562=CARTESIAN_POINT('',(325.942335135839,150.2,-141.9508));
#26563=CARTESIAN_POINT('Origin',(325.942335135839,150.2,-144.4908));
#26564=CARTESIAN_POINT('',(323.436899509249,114.27319693366,-144.07319693366));
#26565=CARTESIAN_POINT('Origin',(325.942335135836,114.690799999997,-144.490799999997));
#26566=CARTESIAN_POINT('',(323.436899509249,150.2,-144.07319693366));
#26567=CARTESIAN_POINT('Origin',(319.496090157384,150.2,-167.71632827912));
#26568=CARTESIAN_POINT('',(319.496090157384,137.91632827912,-167.71632827912));
#26569=CARTESIAN_POINT('',(318.48640167016,143.974017294229,-173.774017294229));
#26570=CARTESIAN_POINT('',(319.496090157384,150.2,-167.71632827912));
#26571=CARTESIAN_POINT('Origin',(312.731413965593,150.2,-166.5888));
#26572=CARTESIAN_POINT('',(312.731413965593,143.6468,-173.4468));
#26573=CARTESIAN_POINT('Origin',(312.7314139656,136.788800000009,-166.588800000009));
#26574=CARTESIAN_POINT('',(312.731413965593,150.2,-173.4468));
#26575=CARTESIAN_POINT('Origin',(312.731413965593,150.2,-173.4468));
#26576=CARTESIAN_POINT('',(267.268586034408,143.6468,-173.4468));
#26577=CARTESIAN_POINT('',(312.731413965593,143.6468,-173.4468));
#26578=CARTESIAN_POINT('',(267.268586034408,150.2,-173.4468));
#26579=CARTESIAN_POINT('Origin',(267.268586034408,150.2,-166.5888));
#26580=CARTESIAN_POINT('',(260.503909842617,137.916328279119,-167.71632827912));
#26581=CARTESIAN_POINT('Origin',(267.268586034409,136.788799999999,-166.588799999999));
#26582=CARTESIAN_POINT('',(260.503909842617,150.2,-167.71632827912));
#26583=CARTESIAN_POINT('Origin',(260.503909842617,150.2,-167.71632827912));
#26584=CARTESIAN_POINT('',(256.563100490752,114.273196933659,-144.073196933659));
#26585=CARTESIAN_POINT('',(261.51359832984,143.974017294229,-173.774017294229));
#26586=CARTESIAN_POINT('',(256.563100490752,150.2,-144.073196933659));
#26587=CARTESIAN_POINT('Origin',(254.057664864162,150.2,-144.4908));
#26588=CARTESIAN_POINT('',(254.057664864163,112.1508,-141.9508));
#26589=CARTESIAN_POINT('Origin',(254.057664864164,114.690799999997,-144.490799999997));
#26590=CARTESIAN_POINT('',(254.057664864163,150.2,-141.9508));
#26591=CARTESIAN_POINT('Origin',(251.9,150.2,-141.9508));
#26592=CARTESIAN_POINT('',(251.9,112.1508,-141.9508));
#26593=CARTESIAN_POINT('',(251.9,112.1508,-141.9508));
#26594=CARTESIAN_POINT('',(251.9,150.2,-141.9508));
#26595=CARTESIAN_POINT('Origin',(251.9,150.2,-180.));
#26596=CARTESIAN_POINT('',(251.9,150.2,-180.));
#26597=CARTESIAN_POINT('Origin',(290.,139.06874412503,-168.86874412503));
#26598=CARTESIAN_POINT('Origin',(9.99492,80.,180.));
#26599=CARTESIAN_POINT('',(9.99491999999973,-6.93889390390723E-15,154.6));
#26600=CARTESIAN_POINT('',(9.99491999999999,6.93889390390723E-15,180.));
#26601=CARTESIAN_POINT('',(9.99491999999999,6.93889390390723E-15,180.));
#26602=CARTESIAN_POINT('',(9.99492,80.,180.));
#26603=CARTESIAN_POINT('',(9.99492,80.,180.));
#26604=CARTESIAN_POINT('',(9.99491999999973,80.,154.6));
#26605=CARTESIAN_POINT('',(9.99492,80.,180.));
#26606=CARTESIAN_POINT('',(9.99491999999973,80.,154.6));
#26607=CARTESIAN_POINT('Origin',(10.,80.,180.));
#26608=CARTESIAN_POINT('',(10.,6.93889390390723E-15,180.));
#26609=CARTESIAN_POINT('',(10.,6.93889390390723E-15,180.));
#26610=CARTESIAN_POINT('',(10.,80.,180.));
#26611=CARTESIAN_POINT('',(10.,80.,180.));
#26612=CARTESIAN_POINT('',(10.,80.,180.));
#26613=CARTESIAN_POINT('Origin',(9.99999999999996,80.,176.83008));
#26614=CARTESIAN_POINT('',(13.16992,-1.38777878078145E-14,176.83008));
#26615=CARTESIAN_POINT('Origin',(9.99999999999996,-1.38777878078145E-14,
176.83008));
#26616=CARTESIAN_POINT('',(13.16992,80.,176.83008));
#26617=CARTESIAN_POINT('',(13.16992,80.,176.83008));
#26618=CARTESIAN_POINT('Origin',(9.99999999999996,80.,176.83008));
#26619=CARTESIAN_POINT('Origin',(13.1699199999998,80.,162.5375));
#26620=CARTESIAN_POINT('',(13.1699199999998,-6.93889390390723E-15,162.5375));
#26621=CARTESIAN_POINT('',(13.1699199999998,-6.93889390390723E-15,162.5375));
#26622=CARTESIAN_POINT('',(13.1699199999998,80.,162.5375));
#26623=CARTESIAN_POINT('',(13.1699199999998,80.,162.5375));
#26624=CARTESIAN_POINT('',(13.1699199999998,80.,162.5375));
#26625=CARTESIAN_POINT('Origin',(17.9324199999998,80.,162.5375));
#26626=CARTESIAN_POINT('',(17.9324199999998,-6.93889390390723E-15,157.775));
#26627=CARTESIAN_POINT('Origin',(17.9324199999998,-6.93889390390723E-15,
162.5375));
#26628=CARTESIAN_POINT('',(17.9324199999998,80.,157.775));
#26629=CARTESIAN_POINT('',(17.9324199999998,80.,157.775));
#26630=CARTESIAN_POINT('Origin',(17.9324199999998,80.,162.5375));
#26631=CARTESIAN_POINT('Origin',(32.2249999999998,80.,157.775));
#26632=CARTESIAN_POINT('',(32.2249999999998,-6.93889390390723E-15,157.775));
#26633=CARTESIAN_POINT('',(32.2249999999998,-6.93889390390723E-15,157.775));
#26634=CARTESIAN_POINT('',(32.2249999999998,80.,157.775));
#26635=CARTESIAN_POINT('',(32.2249999999998,80.,157.775));
#26636=CARTESIAN_POINT('',(32.2249999999998,80.,157.775));
#26637=CARTESIAN_POINT('Origin',(32.2249999999997,80.,154.60508));
#26638=CARTESIAN_POINT('',(35.3949199999997,-2.08166817117217E-14,154.60508));
#26639=CARTESIAN_POINT('Origin',(32.2249999999997,-1.38777878078145E-14,
154.60508));
#26640=CARTESIAN_POINT('',(35.3949199999997,80.,154.60508));
#26641=CARTESIAN_POINT('',(35.3949199999997,80.,154.60508));
#26642=CARTESIAN_POINT('Origin',(32.2249999999997,80.,154.60508));
#26643=CARTESIAN_POINT('Origin',(35.3949199999997,80.,154.6));
#26644=CARTESIAN_POINT('',(35.3949199999997,-2.08166817117217E-14,154.6));
#26645=CARTESIAN_POINT('',(35.3949199999997,-2.08166817117217E-14,154.6));
#26646=CARTESIAN_POINT('',(35.3949199999997,80.,154.6));
#26647=CARTESIAN_POINT('',(35.3949199999997,80.,154.6));
#26648=CARTESIAN_POINT('',(35.3949199999997,80.,154.6));
#26649=CARTESIAN_POINT('Origin',(9.99491999999973,80.,154.6));
#26650=CARTESIAN_POINT('',(9.99491999999973,-6.93889390390723E-15,154.6));
#26651=CARTESIAN_POINT('',(9.99491999999973,80.,154.6));
#26652=CARTESIAN_POINT('Origin',(32.2249999999997,80.,154.60508));
#26653=CARTESIAN_POINT('Origin',(32.2249999999997,-1.38777878078145E-14,
154.60508));
#26654=CARTESIAN_POINT('Origin',(210.00508,4.16333634234434E-14,180.));
#26655=CARTESIAN_POINT('',(210.00508,80.,154.6));
#26656=CARTESIAN_POINT('',(210.00508,80.0000000000001,180.));
#26657=CARTESIAN_POINT('',(210.00508,80.0000000000001,180.));
#26658=CARTESIAN_POINT('',(210.00508,4.16333634234434E-14,180.));
#26659=CARTESIAN_POINT('',(210.00508,4.16333634234434E-14,180.));
#26660=CARTESIAN_POINT('',(210.00508,1.38777878078145E-14,154.6));
#26661=CARTESIAN_POINT('',(210.00508,4.16333634234434E-14,180.));
#26662=CARTESIAN_POINT('',(210.00508,1.38777878078145E-14,154.6));
#26663=CARTESIAN_POINT('Origin',(210.,4.16333634234434E-14,180.));
#26664=CARTESIAN_POINT('',(210.,80.0000000000001,180.));
#26665=CARTESIAN_POINT('',(210.,80.0000000000001,180.));
#26666=CARTESIAN_POINT('',(210.,4.16333634234434E-14,180.));
#26667=CARTESIAN_POINT('',(210.,4.16333634234434E-14,180.));
#26668=CARTESIAN_POINT('',(210.,4.16333634234434E-14,180.));
#26669=CARTESIAN_POINT('Origin',(210.,2.08166817117217E-14,176.83008));
#26670=CARTESIAN_POINT('',(206.83008,80.0000000000001,176.83008));
#26671=CARTESIAN_POINT('Origin',(210.,80.,176.83008));
#26672=CARTESIAN_POINT('',(206.83008,4.85722573273506E-14,176.83008));
#26673=CARTESIAN_POINT('',(206.83008,4.85722573273506E-14,176.83008));
#26674=CARTESIAN_POINT('Origin',(210.,2.08166817117217E-14,176.83008));
#26675=CARTESIAN_POINT('Origin',(206.83008,2.77555756156289E-14,162.5375));
#26676=CARTESIAN_POINT('',(206.83008,80.,162.5375));
#26677=CARTESIAN_POINT('',(206.83008,80.,162.5375));
#26678=CARTESIAN_POINT('',(206.83008,2.77555756156289E-14,162.5375));
#26679=CARTESIAN_POINT('',(206.83008,2.77555756156289E-14,162.5375));
#26680=CARTESIAN_POINT('',(206.83008,2.77555756156289E-14,162.5375));
#26681=CARTESIAN_POINT('Origin',(202.06758,2.77555756156289E-14,162.5375));
#26682=CARTESIAN_POINT('',(202.06758,80.,157.775));
#26683=CARTESIAN_POINT('Origin',(202.06758,80.,162.5375));
#26684=CARTESIAN_POINT('',(202.06758,2.77555756156289E-14,157.775));
#26685=CARTESIAN_POINT('',(202.06758,2.77555756156289E-14,157.775));
#26686=CARTESIAN_POINT('Origin',(202.06758,2.77555756156289E-14,162.5375));
#26687=CARTESIAN_POINT('Origin',(187.775,2.77555756156289E-14,157.775));
#26688=CARTESIAN_POINT('',(187.775,80.,157.775));
#26689=CARTESIAN_POINT('',(187.775,80.,157.775));
#26690=CARTESIAN_POINT('',(187.775,2.77555756156289E-14,157.775));
#26691=CARTESIAN_POINT('',(187.775,2.77555756156289E-14,157.775));
#26692=CARTESIAN_POINT('',(187.775,2.77555756156289E-14,157.775));
#26693=CARTESIAN_POINT('Origin',(187.775,1.38777878078145E-14,154.60508));
#26694=CARTESIAN_POINT('',(184.60508,80.,154.60508));
#26695=CARTESIAN_POINT('Origin',(187.775,80.,154.60508));
#26696=CARTESIAN_POINT('',(184.60508,4.16333634234434E-14,154.60508));
#26697=CARTESIAN_POINT('',(184.60508,4.16333634234434E-14,154.60508));
#26698=CARTESIAN_POINT('Origin',(187.775,1.38777878078145E-14,154.60508));
#26699=CARTESIAN_POINT('Origin',(184.60508,4.16333634234434E-14,154.6));
#26700=CARTESIAN_POINT('',(184.60508,80.,154.6));
#26701=CARTESIAN_POINT('',(184.60508,80.,154.6));
#26702=CARTESIAN_POINT('',(184.60508,4.16333634234434E-14,154.6));
#26703=CARTESIAN_POINT('',(184.60508,4.16333634234434E-14,154.6));
#26704=CARTESIAN_POINT('',(184.60508,4.16333634234434E-14,154.6));
#26705=CARTESIAN_POINT('Origin',(210.00508,1.38777878078145E-14,154.6));
#26706=CARTESIAN_POINT('',(210.00508,80.,154.6));
#26707=CARTESIAN_POINT('',(210.00508,1.38777878078145E-14,154.6));
#26708=CARTESIAN_POINT('Origin',(187.775,1.38777878078145E-14,154.60508));
#26709=CARTESIAN_POINT('Origin',(187.775,80.,154.60508));
#26710=CARTESIAN_POINT('Origin',(9.99492,80.,-180.));
#26711=CARTESIAN_POINT('',(9.99491999999973,-9.72456449527445E-15,-154.6));
#26712=CARTESIAN_POINT('',(9.99492,4.62223186652937E-30,-180.));
#26713=CARTESIAN_POINT('',(9.99492,4.62223186652937E-30,-180.));
#26714=CARTESIAN_POINT('',(9.99491999999973,80.,-154.6));
#26715=CARTESIAN_POINT('',(9.99491999999973,80.,-154.6));
#26716=CARTESIAN_POINT('',(9.99492,80.,-180.));
#26717=CARTESIAN_POINT('',(9.99492,80.,-180.));
#26718=CARTESIAN_POINT('',(9.99492,80.,-180.));
#26719=CARTESIAN_POINT('Origin',(10.,80.,-180.));
#26720=CARTESIAN_POINT('',(10.,3.08148791101958E-30,-180.));
#26721=CARTESIAN_POINT('',(10.,4.62223186652937E-30,-180.));
#26722=CARTESIAN_POINT('',(10.,80.,-180.));
#26723=CARTESIAN_POINT('',(10.,80.,-180.));
#26724=CARTESIAN_POINT('',(10.,80.,-180.));
#26725=CARTESIAN_POINT('Origin',(9.99999999999996,80.,-176.83008));
#26726=CARTESIAN_POINT('',(13.16992,-1.21362564901026E-15,-176.83008));
#26727=CARTESIAN_POINT('Origin',(9.99999999999996,-1.21362564901025E-15,
-176.83008));
#26728=CARTESIAN_POINT('',(13.16992,80.,-176.83008));
#26729=CARTESIAN_POINT('Origin',(9.99999999999996,80.,-176.83008));
#26730=CARTESIAN_POINT('',(13.16992,80.,-176.83008));
#26731=CARTESIAN_POINT('Origin',(13.1699199999998,80.,-162.5375));
#26732=CARTESIAN_POINT('',(13.1699199999998,-6.68563809050119E-15,-162.5375));
#26733=CARTESIAN_POINT('',(13.1699199999998,-6.68563809050119E-15,-162.5375));
#26734=CARTESIAN_POINT('',(13.1699199999998,80.,-162.5375));
#26735=CARTESIAN_POINT('',(13.1699199999998,80.,-162.5375));
#26736=CARTESIAN_POINT('',(13.1699199999998,80.,-162.5375));
#26737=CARTESIAN_POINT('Origin',(17.9324199999998,80.,-162.5375));
#26738=CARTESIAN_POINT('',(17.9324199999998,-8.50899393336517E-15,-157.775));
#26739=CARTESIAN_POINT('Origin',(17.9324199999998,-6.68563809050121E-15,
-162.5375));
#26740=CARTESIAN_POINT('',(17.9324199999998,80.,-157.775));
#26741=CARTESIAN_POINT('Origin',(17.9324199999998,80.,-162.5375));
#26742=CARTESIAN_POINT('',(17.9324199999998,80.,-157.775));
#26743=CARTESIAN_POINT('Origin',(32.2249999999998,80.,-157.775));
#26744=CARTESIAN_POINT('',(32.2249999999998,-8.50899393336523E-15,-157.775));
#26745=CARTESIAN_POINT('',(32.2249999999998,-8.50899393336523E-15,-157.775));
#26746=CARTESIAN_POINT('',(32.2249999999998,80.,-157.775));
#26747=CARTESIAN_POINT('',(32.2249999999998,80.,-157.775));
#26748=CARTESIAN_POINT('',(32.2249999999998,80.,-157.775));
#26749=CARTESIAN_POINT('Origin',(32.2249999999997,80.,-154.60508));
#26750=CARTESIAN_POINT('',(35.3949199999997,-9.72261958237549E-15,-154.60508));
#26751=CARTESIAN_POINT('Origin',(32.2249999999997,-9.72261958237548E-15,
-154.60508));
#26752=CARTESIAN_POINT('',(35.3949199999997,80.,-154.60508));
#26753=CARTESIAN_POINT('Origin',(32.2249999999997,80.,-154.60508));
#26754=CARTESIAN_POINT('',(35.3949199999997,80.,-154.60508));
#26755=CARTESIAN_POINT('Origin',(35.3949199999997,80.,-154.6));
#26756=CARTESIAN_POINT('',(35.3949199999997,-9.72456449527455E-15,-154.6));
#26757=CARTESIAN_POINT('',(35.3949199999997,-9.72456449527455E-15,-154.6));
#26758=CARTESIAN_POINT('',(35.3949199999997,80.,-154.6));
#26759=CARTESIAN_POINT('',(35.3949199999997,80.,-154.6));
#26760=CARTESIAN_POINT('',(35.3949199999997,80.,-154.6));
#26761=CARTESIAN_POINT('Origin',(9.99491999999973,80.,-154.6));
#26762=CARTESIAN_POINT('',(9.99491999999973,-9.72456449527445E-15,-154.6));
#26763=CARTESIAN_POINT('',(9.99491999999973,80.,-154.6));
#26764=CARTESIAN_POINT('Origin',(32.2249999999997,80.,-154.60508));
#26765=CARTESIAN_POINT('Origin',(32.2249999999997,-9.72261958237548E-15,
-154.60508));
#26766=CARTESIAN_POINT('Origin',(210.00508,4.16333634234434E-14,-180.));
#26767=CARTESIAN_POINT('',(210.00508,80.,-154.6));
#26768=CARTESIAN_POINT('',(210.00508,80.0000000000001,-180.));
#26769=CARTESIAN_POINT('',(210.00508,80.0000000000001,-180.));
#26770=CARTESIAN_POINT('',(210.00508,1.38777878078145E-14,-154.6));
#26771=CARTESIAN_POINT('',(210.00508,1.38777878078145E-14,-154.6));
#26772=CARTESIAN_POINT('',(210.00508,4.16333634234434E-14,-180.));
#26773=CARTESIAN_POINT('',(210.00508,4.16333634234434E-14,-180.));
#26774=CARTESIAN_POINT('',(210.00508,4.16333634234434E-14,-180.));
#26775=CARTESIAN_POINT('Origin',(210.,4.16333634234434E-14,-180.));
#26776=CARTESIAN_POINT('',(210.,80.0000000000001,-180.));
#26777=CARTESIAN_POINT('',(210.,80.0000000000001,-180.));
#26778=CARTESIAN_POINT('',(210.,4.16333634234434E-14,-180.));
#26779=CARTESIAN_POINT('',(210.,4.16333634234434E-14,-180.));
#26780=CARTESIAN_POINT('',(210.,4.16333634234434E-14,-180.));
#26781=CARTESIAN_POINT('Origin',(210.,2.77555756156289E-14,-176.83008));
#26782=CARTESIAN_POINT('',(206.83008,80.,-176.83008));
#26783=CARTESIAN_POINT('Origin',(210.,80.,-176.83008));
#26784=CARTESIAN_POINT('',(206.83008,2.77555756156289E-14,-176.83008));
#26785=CARTESIAN_POINT('Origin',(210.,2.77555756156289E-14,-176.83008));
#26786=CARTESIAN_POINT('',(206.83008,2.77555756156289E-14,-176.83008));
#26787=CARTESIAN_POINT('Origin',(206.83008,2.77555756156289E-14,-162.5375));
#26788=CARTESIAN_POINT('',(206.83008,80.,-162.5375));
#26789=CARTESIAN_POINT('',(206.83008,80.,-162.5375));
#26790=CARTESIAN_POINT('',(206.83008,2.77555756156289E-14,-162.5375));
#26791=CARTESIAN_POINT('',(206.83008,2.77555756156289E-14,-162.5375));
#26792=CARTESIAN_POINT('',(206.83008,2.77555756156289E-14,-162.5375));
#26793=CARTESIAN_POINT('Origin',(202.06758,2.77555756156289E-14,-162.5375));
#26794=CARTESIAN_POINT('',(202.06758,80.,-157.775));
#26795=CARTESIAN_POINT('Origin',(202.06758,80.,-162.5375));
#26796=CARTESIAN_POINT('',(202.06758,1.38777878078145E-14,-157.775));
#26797=CARTESIAN_POINT('Origin',(202.06758,2.77555756156289E-14,-162.5375));
#26798=CARTESIAN_POINT('',(202.06758,1.38777878078145E-14,-157.775));
#26799=CARTESIAN_POINT('Origin',(187.775,1.38777878078145E-14,-157.775));
#26800=CARTESIAN_POINT('',(187.775,80.,-157.775));
#26801=CARTESIAN_POINT('',(187.775,80.,-157.775));
#26802=CARTESIAN_POINT('',(187.775,1.38777878078145E-14,-157.775));
#26803=CARTESIAN_POINT('',(187.775,1.38777878078145E-14,-157.775));
#26804=CARTESIAN_POINT('',(187.775,1.38777878078145E-14,-157.775));
#26805=CARTESIAN_POINT('Origin',(187.775,1.38777878078145E-14,-154.60508));
#26806=CARTESIAN_POINT('',(184.60508,80.,-154.60508));
#26807=CARTESIAN_POINT('Origin',(187.775,80.,-154.60508));
#26808=CARTESIAN_POINT('',(184.60508,1.38777878078145E-14,-154.60508));
#26809=CARTESIAN_POINT('Origin',(187.775,1.38777878078145E-14,-154.60508));
#26810=CARTESIAN_POINT('',(184.60508,1.38777878078145E-14,-154.60508));
#26811=CARTESIAN_POINT('Origin',(184.60508,1.38777878078145E-14,-154.6));
#26812=CARTESIAN_POINT('',(184.60508,80.,-154.6));
#26813=CARTESIAN_POINT('',(184.60508,80.,-154.6));
#26814=CARTESIAN_POINT('',(184.60508,1.38777878078145E-14,-154.6));
#26815=CARTESIAN_POINT('',(184.60508,1.38777878078145E-14,-154.6));
#26816=CARTESIAN_POINT('',(184.60508,1.38777878078145E-14,-154.6));
#26817=CARTESIAN_POINT('Origin',(210.00508,1.38777878078145E-14,-154.6));
#26818=CARTESIAN_POINT('',(210.00508,80.,-154.6));
#26819=CARTESIAN_POINT('',(210.00508,1.38777878078145E-14,-154.6));
#26820=CARTESIAN_POINT('Origin',(187.775,1.38777878078145E-14,-154.60508));
#26821=CARTESIAN_POINT('Origin',(187.775,80.,-154.60508));
#26822=CARTESIAN_POINT('Origin',(502.23008,4.16333634234434E-14,124.99492));
#26823=CARTESIAN_POINT('',(480.,-1.2490009027033E-13,125.));
#26824=CARTESIAN_POINT('',(480.,-1.2490009027033E-13,99.6));
#26825=CARTESIAN_POINT('',(480.,-1.2490009027033E-13,99.6));
#26826=CARTESIAN_POINT('',(480.00508,-8.32667268468867E-14,99.6));
#26827=CARTESIAN_POINT('',(480.00508,-8.32667268468867E-14,99.6));
#26828=CARTESIAN_POINT('',(483.175,-4.16333634234434E-14,102.76992));
#26829=CARTESIAN_POINT('Origin',(480.00508,-1.2490009027033E-13,102.76992));
#26830=CARTESIAN_POINT('',(483.175,-4.16333634234434E-14,117.0625));
#26831=CARTESIAN_POINT('',(483.175,-4.16333634234434E-14,117.0625));
#26832=CARTESIAN_POINT('',(487.9375,-8.32667268468867E-14,121.825));
#26833=CARTESIAN_POINT('Origin',(487.9375,-8.32667268468867E-14,117.0625));
#26834=CARTESIAN_POINT('',(502.23008,4.16333634234434E-14,121.825));
#26835=CARTESIAN_POINT('',(502.23008,4.16333634234434E-14,121.825));
#26836=CARTESIAN_POINT('',(505.4,-4.16333634234434E-14,124.99492));
#26837=CARTESIAN_POINT('Origin',(502.23008,4.16333634234434E-14,124.99492));
#26838=CARTESIAN_POINT('',(505.4,-8.32667268468867E-14,125.));
#26839=CARTESIAN_POINT('',(505.4,-8.32667268468867E-14,125.));
#26840=CARTESIAN_POINT('',(480.,-1.2490009027033E-13,125.));
#26841=CARTESIAN_POINT('Origin',(480.,-1.2490009027033E-13,125.));
#26842=CARTESIAN_POINT('',(505.4,132.,125.));
#26843=CARTESIAN_POINT('',(505.4,-8.32667268468867E-14,125.));
#26844=CARTESIAN_POINT('',(480.,132.,125.));
#26845=CARTESIAN_POINT('',(479.999999999999,132.,125.));
#26846=CARTESIAN_POINT('',(480.,-1.2490009027033E-13,125.));
#26847=CARTESIAN_POINT('Origin',(505.4,-8.32667268468867E-14,125.));
#26848=CARTESIAN_POINT('',(505.4,131.99492,124.99492));
#26849=CARTESIAN_POINT('',(505.4,-4.16333634234434E-14,124.99492));
#26850=CARTESIAN_POINT('',(505.4,66.0000000000001,59.0000000000001));
#26851=CARTESIAN_POINT('Origin',(502.23008,4.16333634234434E-14,124.99492));
#26852=CARTESIAN_POINT('',(502.23008,128.825,121.825));
#26853=CARTESIAN_POINT('',(502.23008,4.16333634234434E-14,121.825));
#26854=CARTESIAN_POINT('Origin',(502.230079999999,131.994920000002,124.994920000002));
#26855=CARTESIAN_POINT('Origin',(502.23008,4.16333634234434E-14,121.825));
#26856=CARTESIAN_POINT('',(487.9375,128.825,121.825));
#26857=CARTESIAN_POINT('',(487.9375,-8.32667268468867E-14,121.825));
#26858=CARTESIAN_POINT('',(502.230079999999,128.825,121.825));
#26859=CARTESIAN_POINT('Origin',(487.9375,-8.32667268468867E-14,117.0625));
#26860=CARTESIAN_POINT('',(483.175,124.0625,117.0625));
#26861=CARTESIAN_POINT('',(483.175,-4.16333634234434E-14,117.0625));
#26862=CARTESIAN_POINT('Origin',(487.937500000006,124.062499999993,117.062499999993));
#26863=CARTESIAN_POINT('Origin',(483.175,-4.16333634234434E-14,117.0625));
#26864=CARTESIAN_POINT('',(483.175,109.76992,102.76992));
#26865=CARTESIAN_POINT('',(483.175,-4.16333634234434E-14,102.76992));
#26866=CARTESIAN_POINT('',(483.175000000001,62.03125,55.03125));
#26867=CARTESIAN_POINT('Origin',(480.00508,-1.2490009027033E-13,102.76992));
#26868=CARTESIAN_POINT('',(480.00508,106.6,99.6));
#26869=CARTESIAN_POINT('',(480.00508,-8.32667268468867E-14,99.6));
#26870=CARTESIAN_POINT('Origin',(480.005080000002,109.769919999998,102.769919999998));
#26871=CARTESIAN_POINT('Origin',(480.00508,-8.32667268468867E-14,99.6));
#26872=CARTESIAN_POINT('',(480.,106.6,99.6));
#26873=CARTESIAN_POINT('',(480.,-1.2490009027033E-13,99.6));
#26874=CARTESIAN_POINT('',(480.00508,106.6,99.6));
#26875=CARTESIAN_POINT('Origin',(480.,-1.2490009027033E-13,99.6));
#26876=CARTESIAN_POINT('',(480.000000000001,53.3,46.3));
#26877=CARTESIAN_POINT('Origin',(487.322189922481,124.67781007752,117.677810077519));
#26878=CARTESIAN_POINT('Origin',(480.,106.6,125.));
#26879=CARTESIAN_POINT('',(480.,106.6,-99.6));
#26880=CARTESIAN_POINT('',(480.,132.,-125.));
#26881=CARTESIAN_POINT('',(480.000000000001,-5.70000000000001,12.7));
#26882=CARTESIAN_POINT('',(480.,106.6,99.6000000000001));
#26883=CARTESIAN_POINT('',(480.,106.6,125.));
#26884=CARTESIAN_POINT('',(480.,132.,125.));
#26885=CARTESIAN_POINT('',(480.,119.3,112.3));
#26886=CARTESIAN_POINT('',(480.,132.,125.));
#26887=CARTESIAN_POINT('Origin',(480.00508,106.6,125.));
#26888=CARTESIAN_POINT('',(480.00508,106.6,-99.6000000000001));
#26889=CARTESIAN_POINT('',(480.00508,106.6,-99.6000000000001));
#26890=CARTESIAN_POINT('',(480.00508,106.6,99.6000000000001));
#26891=CARTESIAN_POINT('',(480.00508,106.6,125.));
#26892=CARTESIAN_POINT('',(480.00508,106.6,99.6000000000001));
#26893=CARTESIAN_POINT('Origin',(480.00508,109.76992,125.));
#26894=CARTESIAN_POINT('',(483.175,109.76992,-102.76992));
#26895=CARTESIAN_POINT('Origin',(480.005079999996,109.769920000004,-102.769920000004));
#26896=CARTESIAN_POINT('',(483.175,109.76992,102.76992));
#26897=CARTESIAN_POINT('',(483.175,109.76992,125.));
#26898=CARTESIAN_POINT('Origin',(480.005080000004,109.769919999996,102.769919999996));
#26899=CARTESIAN_POINT('Origin',(483.175,124.0625,125.));
#26900=CARTESIAN_POINT('',(483.175,124.0625,-117.0625));
#26901=CARTESIAN_POINT('',(483.175000000001,3.03124999999993,3.96874999999999));
#26902=CARTESIAN_POINT('',(483.175,124.0625,117.0625));
#26903=CARTESIAN_POINT('',(483.175,124.0625,125.));
#26904=CARTESIAN_POINT('',(483.175,128.03125,121.03125));
#26905=CARTESIAN_POINT('Origin',(487.9375,124.0625,125.));
#26906=CARTESIAN_POINT('',(487.9375,128.825,-121.825));
#26907=CARTESIAN_POINT('Origin',(487.9375,124.062500000001,-117.062500000001));
#26908=CARTESIAN_POINT('',(487.9375,128.825,121.825));
#26909=CARTESIAN_POINT('',(487.9375,128.825,125.));
#26910=CARTESIAN_POINT('Origin',(487.937500000005,124.062499999995,117.062499999995));
#26911=CARTESIAN_POINT('Origin',(502.23008,128.825,125.));
#26912=CARTESIAN_POINT('',(502.23008,128.825,-121.825));
#26913=CARTESIAN_POINT('',(502.230079999997,128.825,-121.825));
#26914=CARTESIAN_POINT('',(502.23008,128.825,121.825));
#26915=CARTESIAN_POINT('',(502.23008,128.825,125.));
#26916=CARTESIAN_POINT('',(502.23008,128.825,121.825));
#26917=CARTESIAN_POINT('Origin',(502.23008,131.99492,125.));
#26918=CARTESIAN_POINT('',(505.4,131.99492,-124.99492));
#26919=CARTESIAN_POINT('Origin',(502.230079999997,131.994920000003,-124.994920000003));
#26920=CARTESIAN_POINT('',(505.4,131.99492,124.99492));
#26921=CARTESIAN_POINT('',(505.4,131.99492,125.));
#26922=CARTESIAN_POINT('Origin',(502.230080000004,131.994919999996,124.994919999996));
#26923=CARTESIAN_POINT('Origin',(505.4,132.,125.));
#26924=CARTESIAN_POINT('',(505.4,132.,-125.));
#26925=CARTESIAN_POINT('',(505.4,7.00000000000003,-1.11022170113618E-13));
#26926=CARTESIAN_POINT('',(505.4,132.,125.));
#26927=CARTESIAN_POINT('',(505.4,132.,125.));
#26928=CARTESIAN_POINT('',(505.4,132.,125.));
#26929=CARTESIAN_POINT('Origin',(480.,132.,125.));
#26930=CARTESIAN_POINT('',(479.999999999997,132.,-125.));
#26931=CARTESIAN_POINT('',(480.,132.,125.));
#26932=CARTESIAN_POINT('Origin',(487.322189922481,124.677810077519,117.67781007752));
#26933=CARTESIAN_POINT('Origin',(487.322189922481,124.677810077519,-117.67781007752));
#26934=CARTESIAN_POINT('Origin',(502.23008,-5.55111512312578E-14,-124.99492));
#26935=CARTESIAN_POINT('',(480.,-8.32667268468867E-14,-125.));
#26936=CARTESIAN_POINT('',(480.,-1.38777878078145E-13,-99.6));
#26937=CARTESIAN_POINT('',(480.,-1.38777878078145E-13,-99.6));
#26938=CARTESIAN_POINT('',(505.4,-8.32667268468867E-14,-125.));
#26939=CARTESIAN_POINT('',(480.,-8.32667268468867E-14,-125.));
#26940=CARTESIAN_POINT('',(505.4,-8.32667268468867E-14,-124.99492));
#26941=CARTESIAN_POINT('',(505.4,-8.32667268468867E-14,-125.));
#26942=CARTESIAN_POINT('',(502.23008,-1.11022302462516E-13,-121.825));
#26943=CARTESIAN_POINT('Origin',(502.23008,-5.55111512312578E-14,-124.99492));
#26944=CARTESIAN_POINT('',(487.9375,-1.11022302462516E-13,-121.825));
#26945=CARTESIAN_POINT('',(502.23008,-1.11022302462516E-13,-121.825));
#26946=CARTESIAN_POINT('',(483.175,-8.32667268468867E-14,-117.0625));
#26947=CARTESIAN_POINT('Origin',(487.9375,-1.11022302462516E-13,-117.0625));
#26948=CARTESIAN_POINT('',(483.175,-2.77555756156289E-14,-102.76992));
#26949=CARTESIAN_POINT('',(483.175,-8.32667268468867E-14,-117.0625));
#26950=CARTESIAN_POINT('',(480.00508,-1.11022302462516E-13,-99.6));
#26951=CARTESIAN_POINT('Origin',(480.00508,-1.11022302462516E-13,-102.76992));
#26952=CARTESIAN_POINT('',(480.00508,-1.11022302462516E-13,-99.6));
#26953=CARTESIAN_POINT('Origin',(480.,132.,-125.));
#26954=CARTESIAN_POINT('',(480.,132.,-125.));
#26955=CARTESIAN_POINT('',(480.,132.,-125.));
#26956=CARTESIAN_POINT('',(505.4,132.,-125.));
#26957=CARTESIAN_POINT('',(480.,132.,-125.));
#26958=CARTESIAN_POINT('',(505.4,132.,-125.));
#26959=CARTESIAN_POINT('Origin',(505.4,132.,-125.));
#26960=CARTESIAN_POINT('',(505.4,131.99492,-124.99492));
#26961=CARTESIAN_POINT('',(505.4,132.,-125.));
#26962=CARTESIAN_POINT('',(505.4,132.,-124.99492));
#26963=CARTESIAN_POINT('Origin',(502.23008,132.,-124.99492));
#26964=CARTESIAN_POINT('',(502.23008,128.825,-121.825));
#26965=CARTESIAN_POINT('Origin',(502.230080000001,131.99492,-124.99492));
#26966=CARTESIAN_POINT('',(502.23008,132.,-121.825));
#26967=CARTESIAN_POINT('Origin',(502.23008,132.,-121.825));
#26968=CARTESIAN_POINT('',(487.9375,128.825,-121.825));
#26969=CARTESIAN_POINT('',(502.23008,128.825,-121.825));
#26970=CARTESIAN_POINT('',(487.9375,132.,-121.825));
#26971=CARTESIAN_POINT('Origin',(487.9375,132.,-117.0625));
#26972=CARTESIAN_POINT('',(483.175,124.0625,-117.0625));
#26973=CARTESIAN_POINT('Origin',(487.937499999997,124.062500000003,-117.062500000003));
#26974=CARTESIAN_POINT('',(483.175,132.,-117.0625));
#26975=CARTESIAN_POINT('Origin',(483.175,132.,-117.0625));
#26976=CARTESIAN_POINT('',(483.175,109.76992,-102.76992));
#26977=CARTESIAN_POINT('',(483.175,128.03125,-121.03125));
#26978=CARTESIAN_POINT('',(483.175,132.,-102.76992));
#26979=CARTESIAN_POINT('Origin',(480.00508,132.,-102.76992));
#26980=CARTESIAN_POINT('',(480.00508,106.6,-99.6));
#26981=CARTESIAN_POINT('Origin',(480.005079999996,109.769920000005,-102.769920000005));
#26982=CARTESIAN_POINT('',(480.00508,132.,-99.6));
#26983=CARTESIAN_POINT('Origin',(480.00508,132.,-99.6));
#26984=CARTESIAN_POINT('',(480.,106.6,-99.6));
#26985=CARTESIAN_POINT('',(480.00508,106.6,-99.6));
#26986=CARTESIAN_POINT('',(480.,132.,-99.6));
#26987=CARTESIAN_POINT('Origin',(480.,132.,-99.6));
#26988=CARTESIAN_POINT('',(480.,119.3,-112.3));
#26989=CARTESIAN_POINT('Origin',(487.322189922481,124.67781007752,-117.677810077519));
#26990=CARTESIAN_POINT('Origin',(659.76992,-5.55111512312578E-14,124.99492));
#26991=CARTESIAN_POINT('',(682.,-1.11022302462516E-13,125.));
#26992=CARTESIAN_POINT('',(682.,-5.55111512312578E-14,99.6));
#26993=CARTESIAN_POINT('',(682.,-5.55111512312578E-14,99.6));
#26994=CARTESIAN_POINT('',(656.6,-5.55111512312578E-14,125.));
#26995=CARTESIAN_POINT('',(682.,-1.11022302462516E-13,125.));
#26996=CARTESIAN_POINT('',(656.6,-5.55111512312578E-14,124.99492));
#26997=CARTESIAN_POINT('',(656.6,-5.55111512312578E-14,125.));
#26998=CARTESIAN_POINT('',(659.76992,-8.32667268468867E-14,121.825));
#26999=CARTESIAN_POINT('Origin',(659.76992,-5.55111512312578E-14,124.99492));
#27000=CARTESIAN_POINT('',(674.0625,-8.32667268468867E-14,121.825));
#27001=CARTESIAN_POINT('',(659.76992,-8.32667268468867E-14,121.825));
#27002=CARTESIAN_POINT('',(678.825,-2.77555756156289E-14,117.0625));
#27003=CARTESIAN_POINT('Origin',(674.0625,-5.55111512312578E-14,117.0625));
#27004=CARTESIAN_POINT('',(678.825,-2.77555756156289E-14,102.76992));
#27005=CARTESIAN_POINT('',(678.825,-2.77555756156289E-14,117.0625));
#27006=CARTESIAN_POINT('',(681.99492,0.,99.6));
#27007=CARTESIAN_POINT('Origin',(681.99492,0.,102.76992));
#27008=CARTESIAN_POINT('',(681.99492,0.,99.6));
#27009=CARTESIAN_POINT('Origin',(682.,132.,125.));
#27010=CARTESIAN_POINT('',(682.,132.,125.));
#27011=CARTESIAN_POINT('',(682.,132.,125.));
#27012=CARTESIAN_POINT('',(656.6,132.,125.));
#27013=CARTESIAN_POINT('',(682.,132.,125.));
#27014=CARTESIAN_POINT('',(656.6,132.,125.));
#27015=CARTESIAN_POINT('Origin',(656.6,132.,125.));
#27016=CARTESIAN_POINT('',(656.6,131.99492,124.99492));
#27017=CARTESIAN_POINT('',(656.6,132.,125.));
#27018=CARTESIAN_POINT('',(656.6,132.,124.99492));
#27019=CARTESIAN_POINT('Origin',(659.76992,132.,124.99492));
#27020=CARTESIAN_POINT('',(659.76992,128.825,121.825));
#27021=CARTESIAN_POINT('Origin',(659.769919999989,131.99491999999,124.99491999999));
#27022=CARTESIAN_POINT('',(659.76992,132.,121.825));
#27023=CARTESIAN_POINT('Origin',(659.76992,132.,121.825));
#27024=CARTESIAN_POINT('',(674.0625,128.825,121.825));
#27025=CARTESIAN_POINT('',(659.76992,128.825,121.825));
#27026=CARTESIAN_POINT('',(674.0625,132.,121.825));
#27027=CARTESIAN_POINT('Origin',(674.0625,132.,117.0625));
#27028=CARTESIAN_POINT('',(678.825,124.0625,117.0625));
#27029=CARTESIAN_POINT('Origin',(674.062500000003,124.062500000003,117.062500000003));
#27030=CARTESIAN_POINT('',(678.825,132.,117.0625));
#27031=CARTESIAN_POINT('Origin',(678.825,132.,117.0625));
#27032=CARTESIAN_POINT('',(678.825,109.76992,102.76992));
#27033=CARTESIAN_POINT('',(678.825,128.03125,121.03125));
#27034=CARTESIAN_POINT('',(678.825,132.,102.76992));
#27035=CARTESIAN_POINT('Origin',(681.99492,132.,102.76992));
#27036=CARTESIAN_POINT('',(681.99492,106.6,99.6));
#27037=CARTESIAN_POINT('Origin',(681.994919999999,109.769919999999,102.769919999998));
#27038=CARTESIAN_POINT('',(681.99492,132.,99.6));
#27039=CARTESIAN_POINT('Origin',(681.99492,132.,99.6));
#27040=CARTESIAN_POINT('',(682.,106.6,99.6));
#27041=CARTESIAN_POINT('',(681.99492,106.6,99.6));
#27042=CARTESIAN_POINT('',(682.,132.,99.6));
#27043=CARTESIAN_POINT('Origin',(682.,132.,99.6));
#27044=CARTESIAN_POINT('',(682.,119.3,112.3));
#27045=CARTESIAN_POINT('Origin',(674.677810077519,124.677810077519,117.677810077519));
#27046=CARTESIAN_POINT('Origin',(682.,106.6,-125.));
#27047=CARTESIAN_POINT('',(682.000000000002,132.,-125.));
#27048=CARTESIAN_POINT('',(682.,106.6,-99.6000000000001));
#27049=CARTESIAN_POINT('',(682.,119.3,-112.3));
#27050=CARTESIAN_POINT('',(682.,132.,125.));
#27051=CARTESIAN_POINT('',(682.,132.,-125.));
#27052=CARTESIAN_POINT('',(682.,106.6,99.6000000000001));
#27053=CARTESIAN_POINT('',(681.999999999999,-5.70000000000004,-12.7));
#27054=CARTESIAN_POINT('',(682.,106.6,-125.));
#27055=CARTESIAN_POINT('Origin',(681.99492,106.6,-125.));
#27056=CARTESIAN_POINT('',(681.99492,106.6,-99.6));
#27057=CARTESIAN_POINT('',(681.99492,106.6,-99.6));
#27058=CARTESIAN_POINT('',(681.99492,106.6,99.6000000000001));
#27059=CARTESIAN_POINT('',(681.994919999999,106.6,99.6000000000001));
#27060=CARTESIAN_POINT('',(681.99492,106.6,-125.));
#27061=CARTESIAN_POINT('Origin',(681.99492,109.76992,-125.));
#27062=CARTESIAN_POINT('',(678.825,109.76992,-102.76992));
#27063=CARTESIAN_POINT('Origin',(681.994919999996,109.769919999996,-102.769919999996));
#27064=CARTESIAN_POINT('',(678.825,109.76992,102.76992));
#27065=CARTESIAN_POINT('Origin',(681.994920000006,109.769920000006,102.769920000006));
#27066=CARTESIAN_POINT('',(678.825,109.76992,-125.));
#27067=CARTESIAN_POINT('Origin',(678.825,124.0625,-125.));
#27068=CARTESIAN_POINT('',(678.825,124.0625,-117.0625));
#27069=CARTESIAN_POINT('',(678.825,128.03125,-121.03125));
#27070=CARTESIAN_POINT('',(678.825,124.0625,117.0625));
#27071=CARTESIAN_POINT('',(678.825,3.03124999999999,-3.96875000000002));
#27072=CARTESIAN_POINT('',(678.825,124.0625,-125.));
#27073=CARTESIAN_POINT('Origin',(674.0625,124.0625,-125.));
#27074=CARTESIAN_POINT('',(674.0625,128.825,-121.825));
#27075=CARTESIAN_POINT('Origin',(674.062500000007,124.062500000007,-117.062500000008));
#27076=CARTESIAN_POINT('',(674.0625,128.825,121.825));
#27077=CARTESIAN_POINT('Origin',(674.062500000002,124.062500000003,117.062500000003));
#27078=CARTESIAN_POINT('',(674.0625,128.825,-125.));
#27079=CARTESIAN_POINT('Origin',(659.76992,128.825,-125.));
#27080=CARTESIAN_POINT('',(659.76992,128.825,-121.825));
#27081=CARTESIAN_POINT('',(659.76992,128.825,-121.825));
#27082=CARTESIAN_POINT('',(659.76992,128.825,121.825));
#27083=CARTESIAN_POINT('',(659.769920000001,128.825,121.825));
#27084=CARTESIAN_POINT('',(659.76992,128.825,-125.));
#27085=CARTESIAN_POINT('Origin',(659.76992,131.99492,-125.));
#27086=CARTESIAN_POINT('',(656.6,131.99492,-124.99492));
#27087=CARTESIAN_POINT('Origin',(659.769919999996,131.994919999995,-124.994919999995));
#27088=CARTESIAN_POINT('',(656.6,131.99492,124.99492));
#27089=CARTESIAN_POINT('Origin',(659.769919999998,131.994919999999,124.99492));
#27090=CARTESIAN_POINT('',(656.6,131.99492,-125.));
#27091=CARTESIAN_POINT('Origin',(656.6,132.,-125.));
#27092=CARTESIAN_POINT('',(656.6,132.,-125.));
#27093=CARTESIAN_POINT('',(656.6,132.,-125.));
#27094=CARTESIAN_POINT('',(656.599999999998,132.,125.));
#27095=CARTESIAN_POINT('',(656.600000000001,6.99999999999999,2.77554962062901E-14));
#27096=CARTESIAN_POINT('',(656.6,132.,-125.));
#27097=CARTESIAN_POINT('Origin',(682.,132.,-125.));
#27098=CARTESIAN_POINT('',(682.,132.,-125.));
#27099=CARTESIAN_POINT('',(682.000000000001,132.,125.));
#27100=CARTESIAN_POINT('Origin',(674.677810077519,124.677810077519,117.67781007752));
#27101=CARTESIAN_POINT('Origin',(674.67781007752,124.677810077519,-117.67781007752));
#27102=CARTESIAN_POINT('Origin',(659.76992,-4.16333634234434E-14,-124.99492));
#27103=CARTESIAN_POINT('',(682.,-2.77555756156289E-14,-125.));
#27104=CARTESIAN_POINT('',(682.,-5.55111512312578E-14,-99.6));
#27105=CARTESIAN_POINT('',(682.,-5.55111512312578E-14,-99.6));
#27106=CARTESIAN_POINT('',(681.99492,-4.16333634234434E-14,-99.6));
#27107=CARTESIAN_POINT('',(681.99492,-4.16333634234434E-14,-99.6));
#27108=CARTESIAN_POINT('',(678.825,-2.77555756156289E-14,-102.76992));
#27109=CARTESIAN_POINT('Origin',(681.99492,-5.55111512312578E-14,-102.76992));
#27110=CARTESIAN_POINT('',(678.825,0.,-117.0625));
#27111=CARTESIAN_POINT('',(678.825,0.,-117.0625));
#27112=CARTESIAN_POINT('',(674.0625,-2.77555756156289E-14,-121.825));
#27113=CARTESIAN_POINT('Origin',(674.0625,-4.16333634234434E-14,-117.0625));
#27114=CARTESIAN_POINT('',(659.76992,-1.38777878078145E-14,-121.825));
#27115=CARTESIAN_POINT('',(659.76992,-1.38777878078145E-14,-121.825));
#27116=CARTESIAN_POINT('',(656.6,-1.38777878078145E-14,-124.99492));
#27117=CARTESIAN_POINT('Origin',(659.76992,-4.16333634234434E-14,-124.99492));
#27118=CARTESIAN_POINT('',(656.6,-4.16333634234434E-14,-125.));
#27119=CARTESIAN_POINT('',(656.6,-4.16333634234434E-14,-125.));
#27120=CARTESIAN_POINT('',(682.,-2.77555756156289E-14,-125.));
#27121=CARTESIAN_POINT('Origin',(682.,-2.77555756156289E-14,-125.));
#27122=CARTESIAN_POINT('',(656.6,132.,-125.));
#27123=CARTESIAN_POINT('',(656.6,-4.16333634234434E-14,-125.));
#27124=CARTESIAN_POINT('',(682.,132.,-125.));
#27125=CARTESIAN_POINT('',(682.000000000001,132.,-125.));
#27126=CARTESIAN_POINT('',(682.,-2.77555756156289E-14,-125.));
#27127=CARTESIAN_POINT('Origin',(656.6,-4.16333634234434E-14,-125.));
#27128=CARTESIAN_POINT('',(656.6,131.99492,-124.99492));
#27129=CARTESIAN_POINT('',(656.6,-1.38777878078145E-14,-124.99492));
#27130=CARTESIAN_POINT('',(656.600000000001,66.0000000000001,-59.));
#27131=CARTESIAN_POINT('Origin',(659.76992,-4.16333634234434E-14,-124.99492));
#27132=CARTESIAN_POINT('',(659.76992,128.825,-121.825));
#27133=CARTESIAN_POINT('',(659.76992,-1.38777878078145E-14,-121.825));
#27134=CARTESIAN_POINT('Origin',(659.769920000007,131.994920000008,-124.994920000007));
#27135=CARTESIAN_POINT('Origin',(659.76992,-1.38777878078145E-14,-121.825));
#27136=CARTESIAN_POINT('',(674.062500000001,128.825,-121.825));
#27137=CARTESIAN_POINT('',(674.0625,-2.77555756156289E-14,-121.825));
#27138=CARTESIAN_POINT('',(659.769920000001,128.825,-121.825));
#27139=CARTESIAN_POINT('Origin',(674.0625,-4.16333634234434E-14,-117.0625));
#27140=CARTESIAN_POINT('',(678.825,124.0625,-117.0625));
#27141=CARTESIAN_POINT('',(678.825,0.,-117.0625));
#27142=CARTESIAN_POINT('Origin',(674.0625,124.062499999999,-117.062499999999));
#27143=CARTESIAN_POINT('Origin',(678.825,0.,-117.0625));
#27144=CARTESIAN_POINT('',(678.825,109.76992,-102.76992));
#27145=CARTESIAN_POINT('',(678.825,-2.77555756156289E-14,-102.76992));
#27146=CARTESIAN_POINT('',(678.825,62.03125,-55.03125));
#27147=CARTESIAN_POINT('Origin',(681.99492,-5.55111512312578E-14,-102.76992));
#27148=CARTESIAN_POINT('',(681.99492,106.6,-99.6));
#27149=CARTESIAN_POINT('',(681.99492,-4.16333634234434E-14,-99.6));
#27150=CARTESIAN_POINT('Origin',(681.994919999999,109.769919999999,-102.769919999998));
#27151=CARTESIAN_POINT('Origin',(681.99492,-4.16333634234434E-14,-99.6));
#27152=CARTESIAN_POINT('',(682.000000000001,106.6,-99.6));
#27153=CARTESIAN_POINT('',(682.,-5.55111512312578E-14,-99.6));
#27154=CARTESIAN_POINT('',(681.99492,106.6,-99.6));
#27155=CARTESIAN_POINT('Origin',(682.,-5.55111512312578E-14,-99.6));
#27156=CARTESIAN_POINT('',(682.,53.3,-46.3));
#27157=CARTESIAN_POINT('Origin',(674.67781007752,124.67781007752,-117.677810077519));
#27158=CARTESIAN_POINT('Origin',(528.5,132.,-64.5));
#27159=CARTESIAN_POINT('',(528.5,132.,-69.));
#27160=CARTESIAN_POINT('',(528.5,132.,-60.));
#27161=CARTESIAN_POINT('Origin',(528.5,132.,-64.5));
#27162=CARTESIAN_POINT('',(528.5,140.,-69.));
#27163=CARTESIAN_POINT('',(528.5,132.,-69.));
#27164=CARTESIAN_POINT('',(528.5,140.,-60.));
#27165=CARTESIAN_POINT('Origin',(528.5,140.,-64.5));
#27166=CARTESIAN_POINT('',(528.5,132.,-60.));
#27167=CARTESIAN_POINT('Origin',(628.5,132.000000000001,-64.5));
#27168=CARTESIAN_POINT('',(628.5,132.000000000001,-69.));
#27169=CARTESIAN_POINT('',(628.5,132.000000000001,-60.));
#27170=CARTESIAN_POINT('Origin',(628.5,132.000000000001,-64.5));
#27171=CARTESIAN_POINT('',(628.5,140.000000000001,-69.));
#27172=CARTESIAN_POINT('',(628.5,132.000000000001,-69.));
#27173=CARTESIAN_POINT('',(628.5,140.000000000001,-60.));
#27174=CARTESIAN_POINT('Origin',(628.5,140.000000000001,-64.5));
#27175=CARTESIAN_POINT('',(628.5,132.000000000001,-60.));
#27176=CARTESIAN_POINT('Origin',(628.5,132.000000000001,64.5));
#27177=CARTESIAN_POINT('',(628.5,132.000000000001,60.));
#27178=CARTESIAN_POINT('',(628.5,132.000000000001,69.));
#27179=CARTESIAN_POINT('Origin',(628.5,132.000000000001,64.5));
#27180=CARTESIAN_POINT('',(628.5,140.000000000001,60.));
#27181=CARTESIAN_POINT('',(628.5,132.000000000001,60.));
#27182=CARTESIAN_POINT('',(628.5,140.000000000001,69.));
#27183=CARTESIAN_POINT('Origin',(628.5,140.000000000001,64.5));
#27184=CARTESIAN_POINT('',(628.5,132.000000000001,69.));
#27185=CARTESIAN_POINT('Origin',(528.5,132.,64.5));
#27186=CARTESIAN_POINT('',(528.5,132.,60.));
#27187=CARTESIAN_POINT('',(528.5,132.,69.));
#27188=CARTESIAN_POINT('Origin',(528.5,132.,64.5));
#27189=CARTESIAN_POINT('',(528.5,140.,60.));
#27190=CARTESIAN_POINT('',(528.5,132.,60.));
#27191=CARTESIAN_POINT('',(528.5,140.,69.));
#27192=CARTESIAN_POINT('Origin',(528.5,140.,64.5));
#27193=CARTESIAN_POINT('',(528.5,132.,69.));
#27194=CARTESIAN_POINT('Origin',(471.,140.,90.));
#27195=CARTESIAN_POINT('',(471.,132.,-79.9999999999999));
#27196=CARTESIAN_POINT('',(471.,132.,79.9999999999999));
#27197=CARTESIAN_POINT('',(471.,132.,90.));
#27198=CARTESIAN_POINT('',(471.,140.,79.9999999999999));
#27199=CARTESIAN_POINT('',(471.,140.,79.9999999999999));
#27200=CARTESIAN_POINT('',(471.,140.,-79.9999999999999));
#27201=CARTESIAN_POINT('',(471.,140.,90.));
#27202=CARTESIAN_POINT('',(471.,140.,-79.9999999999999));
#27203=CARTESIAN_POINT('Origin',(471.,140.,90.));
#27204=CARTESIAN_POINT('',(481.,140.,90.));
#27205=CARTESIAN_POINT('',(681.,140.000000000002,90.));
#27206=CARTESIAN_POINT('',(471.,140.,90.));
#27207=CARTESIAN_POINT('',(481.,132.,90.));
#27208=CARTESIAN_POINT('',(481.,140.,90.));
#27209=CARTESIAN_POINT('',(681.,132.000000000002,90.));
#27210=CARTESIAN_POINT('',(471.,132.,90.));
#27211=CARTESIAN_POINT('',(681.,140.000000000002,90.));
#27212=CARTESIAN_POINT('Origin',(691.,140.000000000002,90.));
#27213=CARTESIAN_POINT('',(691.,132.000000000002,80.));
#27214=CARTESIAN_POINT('',(691.,132.000000000002,-80.));
#27215=CARTESIAN_POINT('',(691.,132.000000000002,90.));
#27216=CARTESIAN_POINT('',(691.,140.000000000002,-80.));
#27217=CARTESIAN_POINT('',(691.,140.000000000002,-80.));
#27218=CARTESIAN_POINT('',(691.,140.000000000002,80.));
#27219=CARTESIAN_POINT('',(691.,140.000000000002,90.));
#27220=CARTESIAN_POINT('',(691.,140.000000000002,80.));
#27221=CARTESIAN_POINT('Origin',(471.,140.,-90.));
#27222=CARTESIAN_POINT('',(681.,132.000000000002,-90.));
#27223=CARTESIAN_POINT('',(481.,132.,-90.));
#27224=CARTESIAN_POINT('',(471.,132.,-90.));
#27225=CARTESIAN_POINT('',(481.,140.,-90.));
#27226=CARTESIAN_POINT('',(481.,140.,-90.));
#27227=CARTESIAN_POINT('',(681.,140.000000000002,-90.));
#27228=CARTESIAN_POINT('',(471.,140.,-90.));
#27229=CARTESIAN_POINT('',(681.,140.000000000002,-90.));
#27230=CARTESIAN_POINT('Origin',(-1.44861900253085E-12,139.999999999995,
1.05879118406788E-22));
#27231=CARTESIAN_POINT('',(481.,140.,90.));
#27232=CARTESIAN_POINT('',(691.,140.000000000002,80.));
#27233=CARTESIAN_POINT('',(681.,140.000000000002,-90.));
#27234=CARTESIAN_POINT('',(471.,140.,-79.9999999999999));
#27235=CARTESIAN_POINT('',(533.5,140.000000000001,-60.));
#27236=CARTESIAN_POINT('',(528.5,140.,-60.));
#27237=CARTESIAN_POINT('',(533.5,140.000000000001,-69.));
#27238=CARTESIAN_POINT('',(528.5,140.,-69.));
#27239=CARTESIAN_POINT('Origin',(533.5,140.000000000001,-64.5));
#27240=CARTESIAN_POINT('',(633.5,140.000000000002,-60.));
#27241=CARTESIAN_POINT('',(628.5,140.000000000001,-60.));
#27242=CARTESIAN_POINT('',(633.5,140.000000000002,-69.));
#27243=CARTESIAN_POINT('',(628.5,140.000000000001,-69.));
#27244=CARTESIAN_POINT('Origin',(633.5,140.000000000002,-64.5));
#27245=CARTESIAN_POINT('',(633.5,140.000000000002,69.));
#27246=CARTESIAN_POINT('',(628.5,140.000000000001,69.));
#27247=CARTESIAN_POINT('',(633.5,140.000000000002,60.));
#27248=CARTESIAN_POINT('',(628.5,140.000000000001,60.));
#27249=CARTESIAN_POINT('Origin',(633.5,140.000000000002,64.5));
#27250=CARTESIAN_POINT('',(533.5,140.000000000001,69.));
#27251=CARTESIAN_POINT('',(528.5,140.,69.));
#27252=CARTESIAN_POINT('',(533.5,140.000000000001,60.));
#27253=CARTESIAN_POINT('',(528.5,140.,60.));
#27254=CARTESIAN_POINT('Origin',(533.5,140.000000000001,64.5));
#27255=CARTESIAN_POINT('Origin',(-1.36557432028889E-12,131.999999999995,
0.));
#27256=CARTESIAN_POINT('',(195.500000000002,131.999999999997,-195.500000000001));
#27257=CARTESIAN_POINT('',(195.499999999998,131.999999999997,195.500000000001));
#27258=CARTESIAN_POINT('',(385.499999999998,131.999999999999,-385.500000000001));
#27259=CARTESIAN_POINT('',(385.499999999996,131.999999999999,385.500000000001));
#27260=CARTESIAN_POINT('',(533.5,132.000000000001,-60.));
#27261=CARTESIAN_POINT('',(528.5,132.,-60.));
#27262=CARTESIAN_POINT('',(533.5,132.000000000001,-69.));
#27263=CARTESIAN_POINT('Origin',(533.5,132.000000000001,-64.5));
#27264=CARTESIAN_POINT('',(528.5,132.,-69.));
#27265=CARTESIAN_POINT('',(633.5,132.000000000002,-60.));
#27266=CARTESIAN_POINT('',(628.5,132.000000000001,-60.));
#27267=CARTESIAN_POINT('',(633.5,132.000000000002,-69.));
#27268=CARTESIAN_POINT('Origin',(633.5,132.000000000002,-64.5));
#27269=CARTESIAN_POINT('',(628.5,132.000000000001,-69.));
#27270=CARTESIAN_POINT('',(633.5,132.000000000002,69.));
#27271=CARTESIAN_POINT('',(628.5,132.000000000001,69.));
#27272=CARTESIAN_POINT('',(633.5,132.000000000002,60.));
#27273=CARTESIAN_POINT('Origin',(633.5,132.000000000002,64.5));
#27274=CARTESIAN_POINT('',(628.5,132.000000000001,60.));
#27275=CARTESIAN_POINT('',(533.5,132.000000000001,69.));
#27276=CARTESIAN_POINT('',(528.5,132.,69.));
#27277=CARTESIAN_POINT('',(533.5,132.000000000001,60.));
#27278=CARTESIAN_POINT('Origin',(533.5,132.000000000001,64.5));
#27279=CARTESIAN_POINT('',(528.5,132.,60.));
#27280=CARTESIAN_POINT('Origin',(528.5,132.,60.));
#27281=CARTESIAN_POINT('',(533.5,132.000000000001,60.));
#27282=CARTESIAN_POINT('Origin',(533.5,132.000000000001,64.5));
#27283=CARTESIAN_POINT('',(533.5,132.000000000001,69.));
#27284=CARTESIAN_POINT('Origin',(528.5,132.,69.));
#27285=CARTESIAN_POINT('Origin',(628.5,132.000000000001,60.));
#27286=CARTESIAN_POINT('',(633.5,132.000000000002,60.));
#27287=CARTESIAN_POINT('Origin',(633.5,132.000000000002,64.5));
#27288=CARTESIAN_POINT('',(633.5,132.000000000002,69.));
#27289=CARTESIAN_POINT('Origin',(628.5,132.000000000001,69.));
#27290=CARTESIAN_POINT('Origin',(628.5,132.000000000001,-69.));
#27291=CARTESIAN_POINT('',(633.5,132.000000000002,-69.));
#27292=CARTESIAN_POINT('Origin',(633.5,132.000000000002,-64.5));
#27293=CARTESIAN_POINT('',(633.5,132.000000000002,-60.));
#27294=CARTESIAN_POINT('Origin',(628.5,132.000000000001,-60.));
#27295=CARTESIAN_POINT('Origin',(528.5,132.,-69.));
#27296=CARTESIAN_POINT('',(533.5,132.000000000001,-69.));
#27297=CARTESIAN_POINT('Origin',(533.5,132.000000000001,-64.5));
#27298=CARTESIAN_POINT('',(533.5,132.000000000001,-60.));
#27299=CARTESIAN_POINT('Origin',(528.5,132.,-60.));
#27300=CARTESIAN_POINT('Origin',(481.,140.,90.));
#27301=CARTESIAN_POINT('Origin',(471.,140.,-79.9999999999999));
#27302=CARTESIAN_POINT('Origin',(681.,140.000000000002,-90.));
#27303=CARTESIAN_POINT('Origin',(691.,140.000000000002,80.));
#27304=CARTESIAN_POINT('Origin',(290.,150.2,-91.9999999999992));
#27305=CARTESIAN_POINT('',(290.,143.6468,-100.749999999999));
#27306=CARTESIAN_POINT('Origin',(290.,143.6468,-91.9999999999992));
#27307=CARTESIAN_POINT('',(290.,150.2,-100.749999999999));
#27308=CARTESIAN_POINT('',(290.,150.2,-100.749999999999));
#27309=CARTESIAN_POINT('Origin',(290.,150.2,-91.9999999999992));
#27310=CARTESIAN_POINT('Origin',(290.,150.2,92.0000000000008));
#27311=CARTESIAN_POINT('',(290.,143.6468,83.2500000000008));
#27312=CARTESIAN_POINT('Origin',(290.,143.6468,92.0000000000008));
#27313=CARTESIAN_POINT('',(290.,150.2,83.2500000000008));
#27314=CARTESIAN_POINT('',(290.,150.2,83.2500000000008));
#27315=CARTESIAN_POINT('Origin',(290.,150.2,92.0000000000008));
#27316=CARTESIAN_POINT('Origin',(251.9,150.2,180.));
#27317=CARTESIAN_POINT('',(251.9,112.1508,-141.9508));
#27318=CARTESIAN_POINT('',(251.9,150.2,-180.));
#27319=CARTESIAN_POINT('',(251.900000000002,-29.8000000000002,1.11022302462516E-13));
#27320=CARTESIAN_POINT('',(251.9,112.1508,141.9508));
#27321=CARTESIAN_POINT('',(251.9,112.1508,180.));
#27322=CARTESIAN_POINT('',(251.9,150.2,180.));
#27323=CARTESIAN_POINT('',(251.9,150.2,180.));
#27324=CARTESIAN_POINT('',(251.9,150.2,180.));
#27325=CARTESIAN_POINT('Origin',(251.9,112.1508,180.));
#27326=CARTESIAN_POINT('',(254.057664864162,112.1508,-141.9508));
#27327=CARTESIAN_POINT('',(251.9,112.1508,-141.9508));
#27328=CARTESIAN_POINT('',(254.057664864162,112.1508,141.9508));
#27329=CARTESIAN_POINT('',(254.057664864162,112.1508,180.));
#27330=CARTESIAN_POINT('',(251.9,112.1508,141.9508));
#27331=CARTESIAN_POINT('Origin',(254.057664864162,114.6908,180.));
#27332=CARTESIAN_POINT('',(256.563100490752,114.273196933659,-144.073196933659));
#27333=CARTESIAN_POINT('Origin',(254.057664864164,114.690799999998,-144.490799999998));
#27334=CARTESIAN_POINT('',(256.563100490752,114.273196933659,144.073196933659));
#27335=CARTESIAN_POINT('',(256.563100490752,114.273196933659,180.));
#27336=CARTESIAN_POINT('Origin',(254.05766486416,114.690800000002,144.490800000002));
#27337=CARTESIAN_POINT('Origin',(260.503909842616,137.916328279119,180.));
#27338=CARTESIAN_POINT('',(260.503909842617,137.916328279119,-167.71632827912));
#27339=CARTESIAN_POINT('',(231.92245785816,-33.5598744437294,3.75987444372938));
#27340=CARTESIAN_POINT('',(260.503909842617,137.916328279119,167.716328279119));
#27341=CARTESIAN_POINT('',(260.503909842617,137.916328279119,180.));
#27342=CARTESIAN_POINT('',(261.51359832984,143.974017294229,173.774017294229));
#27343=CARTESIAN_POINT('Origin',(267.268586034408,136.7888,180.));
#27344=CARTESIAN_POINT('',(267.268586034408,143.6468,-173.4468));
#27345=CARTESIAN_POINT('Origin',(267.268586034408,136.788799999999,-166.588799999999));
#27346=CARTESIAN_POINT('',(267.268586034408,143.6468,173.4468));
#27347=CARTESIAN_POINT('',(267.268586034408,143.6468,180.));
#27348=CARTESIAN_POINT('Origin',(267.268586034408,136.788799999999,166.5888));
#27349=CARTESIAN_POINT('Origin',(312.731413965592,143.6468,180.));
#27350=CARTESIAN_POINT('',(312.731413965592,143.6468,-173.4468));
#27351=CARTESIAN_POINT('',(312.731413965589,143.6468,-173.4468));
#27352=CARTESIAN_POINT('',(312.731413965592,143.6468,173.4468));
#27353=CARTESIAN_POINT('',(312.731413965592,143.6468,180.));
#27354=CARTESIAN_POINT('',(312.731413965592,143.6468,173.4468));
#27355=CARTESIAN_POINT('Origin',(312.731413965592,136.7888,180.));
#27356=CARTESIAN_POINT('',(319.496090157384,137.91632827912,-167.71632827912));
#27357=CARTESIAN_POINT('Origin',(312.731413965593,136.788800000001,-166.588800000001));
#27358=CARTESIAN_POINT('',(319.496090157384,137.91632827912,167.71632827912));
#27359=CARTESIAN_POINT('',(319.496090157384,137.91632827912,180.));
#27360=CARTESIAN_POINT('Origin',(312.731413965592,136.788799999999,166.588799999999));
#27361=CARTESIAN_POINT('Origin',(319.496090157384,137.91632827912,180.));
#27362=CARTESIAN_POINT('',(323.436899509249,114.27319693366,-144.07319693366));
#27363=CARTESIAN_POINT('',(348.077542141844,-33.5598744437285,3.75987444372849));
#27364=CARTESIAN_POINT('',(323.436899509249,114.27319693366,144.07319693366));
#27365=CARTESIAN_POINT('',(323.436899509249,114.27319693366,180.));
#27366=CARTESIAN_POINT('',(318.48640167016,143.974017294229,173.774017294229));
#27367=CARTESIAN_POINT('Origin',(325.942335135838,114.6908,180.));
#27368=CARTESIAN_POINT('',(325.942335135838,112.1508,-141.9508));
#27369=CARTESIAN_POINT('Origin',(325.942335135832,114.690799999993,-144.490799999993));
#27370=CARTESIAN_POINT('',(325.942335135838,112.1508,141.9508));
#27371=CARTESIAN_POINT('',(325.942335135838,112.1508,180.));
#27372=CARTESIAN_POINT('Origin',(325.942335135844,114.690800000007,144.490800000007));
#27373=CARTESIAN_POINT('Origin',(328.1,112.1508,180.));
#27374=CARTESIAN_POINT('',(328.1,112.1508,-141.9508));
#27375=CARTESIAN_POINT('',(328.1,112.1508,-141.9508));
#27376=CARTESIAN_POINT('',(328.1,112.1508,141.9508));
#27377=CARTESIAN_POINT('',(328.1,112.1508,180.));
#27378=CARTESIAN_POINT('',(328.1,112.1508,141.9508));
#27379=CARTESIAN_POINT('Origin',(328.1,150.2,180.));
#27380=CARTESIAN_POINT('',(328.1,150.2,-180.));
#27381=CARTESIAN_POINT('',(328.100000000002,-29.7999999999998,-2.4980018054066E-13));
#27382=CARTESIAN_POINT('',(328.1,150.2,180.));
#27383=CARTESIAN_POINT('',(328.1,150.2,180.));
#27384=CARTESIAN_POINT('',(328.1,150.2,180.));
#27385=CARTESIAN_POINT('Origin',(251.9,150.2,180.));
#27386=CARTESIAN_POINT('',(251.899999999996,150.2,-180.));
#27387=CARTESIAN_POINT('',(251.9,150.2,180.));
#27388=CARTESIAN_POINT('Origin',(290.,139.06874412503,168.86874412503));
#27389=CARTESIAN_POINT('Origin',(290.,139.06874412503,-168.86874412503));
#27390=CARTESIAN_POINT('Origin',(45.,80.0050800000034,169.));
#27391=CARTESIAN_POINT('',(45.,76.83008,164.5));
#27392=CARTESIAN_POINT('Origin',(45.,76.8300800000001,169.));
#27393=CARTESIAN_POINT('',(45.,80.0050800000034,164.5));
#27394=CARTESIAN_POINT('',(45.,80.0050800000034,164.5));
#27395=CARTESIAN_POINT('Origin',(45.,80.0050800000034,169.));
#27396=CARTESIAN_POINT('Origin',(175.,80.0050800000034,169.));
#27397=CARTESIAN_POINT('',(175.,76.83008,164.5));
#27398=CARTESIAN_POINT('Origin',(175.,76.8300800000001,169.));
#27399=CARTESIAN_POINT('',(175.,80.0050800000034,164.5));
#27400=CARTESIAN_POINT('',(175.,80.0050800000034,164.5));
#27401=CARTESIAN_POINT('Origin',(175.,80.0050800000034,169.));
#27402=CARTESIAN_POINT('Origin',(210.,80.00508,180.));
#27403=CARTESIAN_POINT('',(10.,80.0050800000003,154.6));
#27404=CARTESIAN_POINT('',(10.,80.00508,180.));
#27405=CARTESIAN_POINT('',(10.,80.00508,180.));
#27406=CARTESIAN_POINT('',(210.,80.00508,180.));
#27407=CARTESIAN_POINT('',(210.,80.00508,180.));
#27408=CARTESIAN_POINT('',(210.,80.0050800000003,154.6));
#27409=CARTESIAN_POINT('',(210.,80.00508,180.));
#27410=CARTESIAN_POINT('',(210.,80.0050800000003,154.6));
#27411=CARTESIAN_POINT('Origin',(210.,80.,180.));
#27412=CARTESIAN_POINT('',(10.,80.,180.));
#27413=CARTESIAN_POINT('',(10.,80.,180.));
#27414=CARTESIAN_POINT('',(210.,80.,180.));
#27415=CARTESIAN_POINT('',(210.,80.,180.));
#27416=CARTESIAN_POINT('',(210.,80.,180.));
#27417=CARTESIAN_POINT('Origin',(210.,80.0000000000001,176.83008));
#27418=CARTESIAN_POINT('',(10.,76.8300800000001,176.83008));
#27419=CARTESIAN_POINT('Origin',(10.,80.0000000000001,176.83008));
#27420=CARTESIAN_POINT('',(210.,76.8300800000001,176.83008));
#27421=CARTESIAN_POINT('',(210.,76.8300800000001,176.83008));
#27422=CARTESIAN_POINT('Origin',(210.,80.0000000000001,176.83008));
#27423=CARTESIAN_POINT('Origin',(210.,76.8300800000002,162.5375));
#27424=CARTESIAN_POINT('',(10.,76.8300800000002,162.5375));
#27425=CARTESIAN_POINT('',(10.,76.8300800000002,162.5375));
#27426=CARTESIAN_POINT('',(210.,76.8300800000002,162.5375));
#27427=CARTESIAN_POINT('',(210.,76.8300800000002,162.5375));
#27428=CARTESIAN_POINT('',(210.,76.8300800000002,162.5375));
#27429=CARTESIAN_POINT('Origin',(210.,72.0675800000002,162.5375));
#27430=CARTESIAN_POINT('',(10.,72.0675800000002,157.775));
#27431=CARTESIAN_POINT('Origin',(10.,72.0675800000002,162.5375));
#27432=CARTESIAN_POINT('',(210.,72.0675800000002,157.775));
#27433=CARTESIAN_POINT('',(210.,72.0675800000002,157.775));
#27434=CARTESIAN_POINT('Origin',(210.,72.0675800000002,162.5375));
#27435=CARTESIAN_POINT('Origin',(210.,57.7750000000002,157.775));
#27436=CARTESIAN_POINT('',(10.,57.7750000000002,157.775));
#27437=CARTESIAN_POINT('',(10.,57.7750000000002,157.775));
#27438=CARTESIAN_POINT('',(210.,57.7750000000002,157.775));
#27439=CARTESIAN_POINT('',(210.,57.7750000000002,157.775));
#27440=CARTESIAN_POINT('',(210.,57.7750000000002,157.775));
#27441=CARTESIAN_POINT('Origin',(210.,57.7750000000002,154.60508));
#27442=CARTESIAN_POINT('',(10.,54.6050800000003,154.60508));
#27443=CARTESIAN_POINT('Origin',(10.,57.7750000000002,154.60508));
#27444=CARTESIAN_POINT('',(210.,54.6050800000003,154.60508));
#27445=CARTESIAN_POINT('',(210.,54.6050800000003,154.60508));
#27446=CARTESIAN_POINT('Origin',(210.,57.7750000000002,154.60508));
#27447=CARTESIAN_POINT('Origin',(210.,54.6050800000003,154.6));
#27448=CARTESIAN_POINT('',(10.,54.6050800000003,154.6));
#27449=CARTESIAN_POINT('',(10.,54.6050800000003,154.6));
#27450=CARTESIAN_POINT('',(210.,54.6050800000003,154.6));
#27451=CARTESIAN_POINT('',(210.,54.6050800000003,154.6));
#27452=CARTESIAN_POINT('',(210.,54.6050800000003,154.6));
#27453=CARTESIAN_POINT('Origin',(210.,80.0050800000003,154.6));
#27454=CARTESIAN_POINT('',(10.,80.0050800000003,154.6));
#27455=CARTESIAN_POINT('',(210.,80.0050800000003,154.6));
#27456=CARTESIAN_POINT('Origin',(210.,57.7750000000002,154.60508));
#27457=CARTESIAN_POINT('Origin',(10.,57.7750000000002,154.60508));
#27458=CARTESIAN_POINT('Origin',(45.,80.0050800000001,-169.));
#27459=CARTESIAN_POINT('',(45.,76.8300800000001,-173.5));
#27460=CARTESIAN_POINT('Origin',(45.,76.8300800000001,-169.));
#27461=CARTESIAN_POINT('',(45.,80.0050800000001,-173.5));
#27462=CARTESIAN_POINT('',(45.,80.0050800000001,-173.5));
#27463=CARTESIAN_POINT('Origin',(45.,80.0050800000001,-169.));
#27464=CARTESIAN_POINT('Origin',(175.,80.0050800000001,-169.));
#27465=CARTESIAN_POINT('',(175.,76.8300800000001,-173.5));
#27466=CARTESIAN_POINT('Origin',(175.,76.8300800000001,-169.));
#27467=CARTESIAN_POINT('',(175.,80.0050800000001,-173.5));
#27468=CARTESIAN_POINT('',(175.,80.0050800000001,-173.5));
#27469=CARTESIAN_POINT('Origin',(175.,80.0050800000001,-169.));
#27470=CARTESIAN_POINT('Origin',(210.,80.00508,-180.));
#27471=CARTESIAN_POINT('',(10.,80.0050800000003,-154.6));
#27472=CARTESIAN_POINT('',(10.,80.00508,-180.));
#27473=CARTESIAN_POINT('',(10.,80.00508,-180.));
#27474=CARTESIAN_POINT('',(210.,80.0050800000003,-154.6));
#27475=CARTESIAN_POINT('',(210.,80.0050800000003,-154.6));
#27476=CARTESIAN_POINT('',(210.,80.00508,-180.));
#27477=CARTESIAN_POINT('',(210.,80.00508,-180.));
#27478=CARTESIAN_POINT('',(210.,80.00508,-180.));
#27479=CARTESIAN_POINT('Origin',(210.,80.,-180.));
#27480=CARTESIAN_POINT('',(10.,80.,-180.));
#27481=CARTESIAN_POINT('',(10.,80.,-180.));
#27482=CARTESIAN_POINT('',(210.,80.,-180.));
#27483=CARTESIAN_POINT('',(210.,80.,-180.));
#27484=CARTESIAN_POINT('',(210.,80.,-180.));
#27485=CARTESIAN_POINT('Origin',(210.,80.0000000000001,-176.83008));
#27486=CARTESIAN_POINT('',(10.,76.8300800000001,-176.83008));
#27487=CARTESIAN_POINT('Origin',(10.,80.0000000000001,-176.83008));
#27488=CARTESIAN_POINT('',(210.,76.8300800000001,-176.83008));
#27489=CARTESIAN_POINT('Origin',(210.,80.0000000000001,-176.83008));
#27490=CARTESIAN_POINT('',(210.,76.8300800000001,-176.83008));
#27491=CARTESIAN_POINT('Origin',(210.,76.8300800000002,-162.5375));
#27492=CARTESIAN_POINT('',(10.,76.8300800000002,-162.5375));
#27493=CARTESIAN_POINT('',(10.,76.8300800000002,-162.5375));
#27494=CARTESIAN_POINT('',(210.,76.8300800000002,-162.5375));
#27495=CARTESIAN_POINT('',(210.,76.8300800000002,-162.5375));
#27496=CARTESIAN_POINT('',(210.,76.8300800000002,-162.5375));
#27497=CARTESIAN_POINT('Origin',(210.,72.0675800000002,-162.5375));
#27498=CARTESIAN_POINT('',(10.,72.0675800000002,-157.775));
#27499=CARTESIAN_POINT('Origin',(10.,72.0675800000002,-162.5375));
#27500=CARTESIAN_POINT('',(210.,72.0675800000002,-157.775));
#27501=CARTESIAN_POINT('Origin',(210.,72.0675800000002,-162.5375));
#27502=CARTESIAN_POINT('',(210.,72.0675800000002,-157.775));
#27503=CARTESIAN_POINT('Origin',(210.,57.7750000000002,-157.775));
#27504=CARTESIAN_POINT('',(10.,57.7750000000002,-157.775));
#27505=CARTESIAN_POINT('',(10.,57.7750000000002,-157.775));
#27506=CARTESIAN_POINT('',(210.,57.7750000000002,-157.775));
#27507=CARTESIAN_POINT('',(210.,57.7750000000002,-157.775));
#27508=CARTESIAN_POINT('',(210.,57.7750000000002,-157.775));
#27509=CARTESIAN_POINT('Origin',(210.,57.7750000000002,-154.60508));
#27510=CARTESIAN_POINT('',(10.,54.6050800000003,-154.60508));
#27511=CARTESIAN_POINT('Origin',(10.,57.7750000000002,-154.60508));
#27512=CARTESIAN_POINT('',(210.,54.6050800000003,-154.60508));
#27513=CARTESIAN_POINT('Origin',(210.,57.7750000000002,-154.60508));
#27514=CARTESIAN_POINT('',(210.,54.6050800000003,-154.60508));
#27515=CARTESIAN_POINT('Origin',(210.,54.6050800000003,-154.6));
#27516=CARTESIAN_POINT('',(10.,54.6050800000003,-154.6));
#27517=CARTESIAN_POINT('',(10.,54.6050800000003,-154.6));
#27518=CARTESIAN_POINT('',(210.,54.6050800000003,-154.6));
#27519=CARTESIAN_POINT('',(210.,54.6050800000003,-154.6));
#27520=CARTESIAN_POINT('',(210.,54.6050800000003,-154.6));
#27521=CARTESIAN_POINT('Origin',(210.,80.0050800000003,-154.6));
#27522=CARTESIAN_POINT('',(10.,80.0050800000003,-154.6));
#27523=CARTESIAN_POINT('',(210.,80.0050800000003,-154.6));
#27524=CARTESIAN_POINT('Origin',(210.,57.7750000000002,-154.60508));
#27525=CARTESIAN_POINT('Origin',(10.,57.7750000000002,-154.60508));
#27534=UNCERTAINTY_MEASURE_WITH_UNIT(LENGTH_MEASURE(0.01),#27542,
'DISTANCE_ACCURACY_VALUE',
'Maximum model space distance between geometric entities at asserted c
onnectivities');
#27535=UNCERTAINTY_MEASURE_WITH_UNIT(LENGTH_MEASURE(0.01),#27542,
'DISTANCE_ACCURACY_VALUE',
'Maximum model space distance between geometric entities at asserted c
onnectivities');
#27540=(
GEOMETRIC_REPRESENTATION_CONTEXT(3)
GLOBAL_UNCERTAINTY_ASSIGNED_CONTEXT((#27534))
GLOBAL_UNIT_ASSIGNED_CONTEXT((#27542,#27544,#27545))
REPRESENTATION_CONTEXT('','3D')
);
#27541=(
GEOMETRIC_REPRESENTATION_CONTEXT(3)
GLOBAL_UNCERTAINTY_ASSIGNED_CONTEXT((#27535))
GLOBAL_UNIT_ASSIGNED_CONTEXT((#27542,#27544,#27545))
REPRESENTATION_CONTEXT('','3D')
);
#27542=(
LENGTH_UNIT()
NAMED_UNIT(*)
SI_UNIT(.MILLI.,.METRE.)
);
#27544=(
NAMED_UNIT(*)
PLANE_ANGLE_UNIT()
SI_UNIT($,.RADIAN.)
);
#27545=(
NAMED_UNIT(*)
SI_UNIT($,.STERADIAN.)
SOLID_ANGLE_UNIT()
);
#27550=SHAPE_DEFINITION_REPRESENTATION(#27555,#27564);
#27555=PRODUCT_DEFINITION_SHAPE('',$,#27570);
#27564=SHAPE_REPRESENTATION('',(#12666),#27540);
#27565=PRODUCT_DEFINITION_CONTEXT('part definition',#27582,'design');
#27570=PRODUCT_DEFINITION('4. Frame','4. Frame',#27575,#27565);
#27575=PRODUCT_DEFINITION_FORMATION('',$,#27588);
#27582=APPLICATION_CONTEXT(
'Core Data for Automotive Mechanical Design Process');
#27583=PRODUCT_CONTEXT('part definition',#27582,'mechanical');
#27588=PRODUCT('4. Frame','4. Frame',$,(#27583));
#27590=PRESENTATION_STYLE_ASSIGNMENT((#27594));
#27594=SURFACE_STYLE_USAGE(.BOTH.,#27598);
#27598=SURFACE_SIDE_STYLE('',(#27602));
#27602=SURFACE_STYLE_FILL_AREA(#27606);
#27606=FILL_AREA_STYLE('Opaque(20,51,87)',(#27610));
#27610=FILL_AREA_STYLE_COLOUR('Opaque(20,51,87)',#27614);
#27614=COLOUR_RGB('Opaque(20,51,87)',0.0784313725490196,0.2,0.341176470588235);
ENDSEC;
END-ISO-10303-21;
